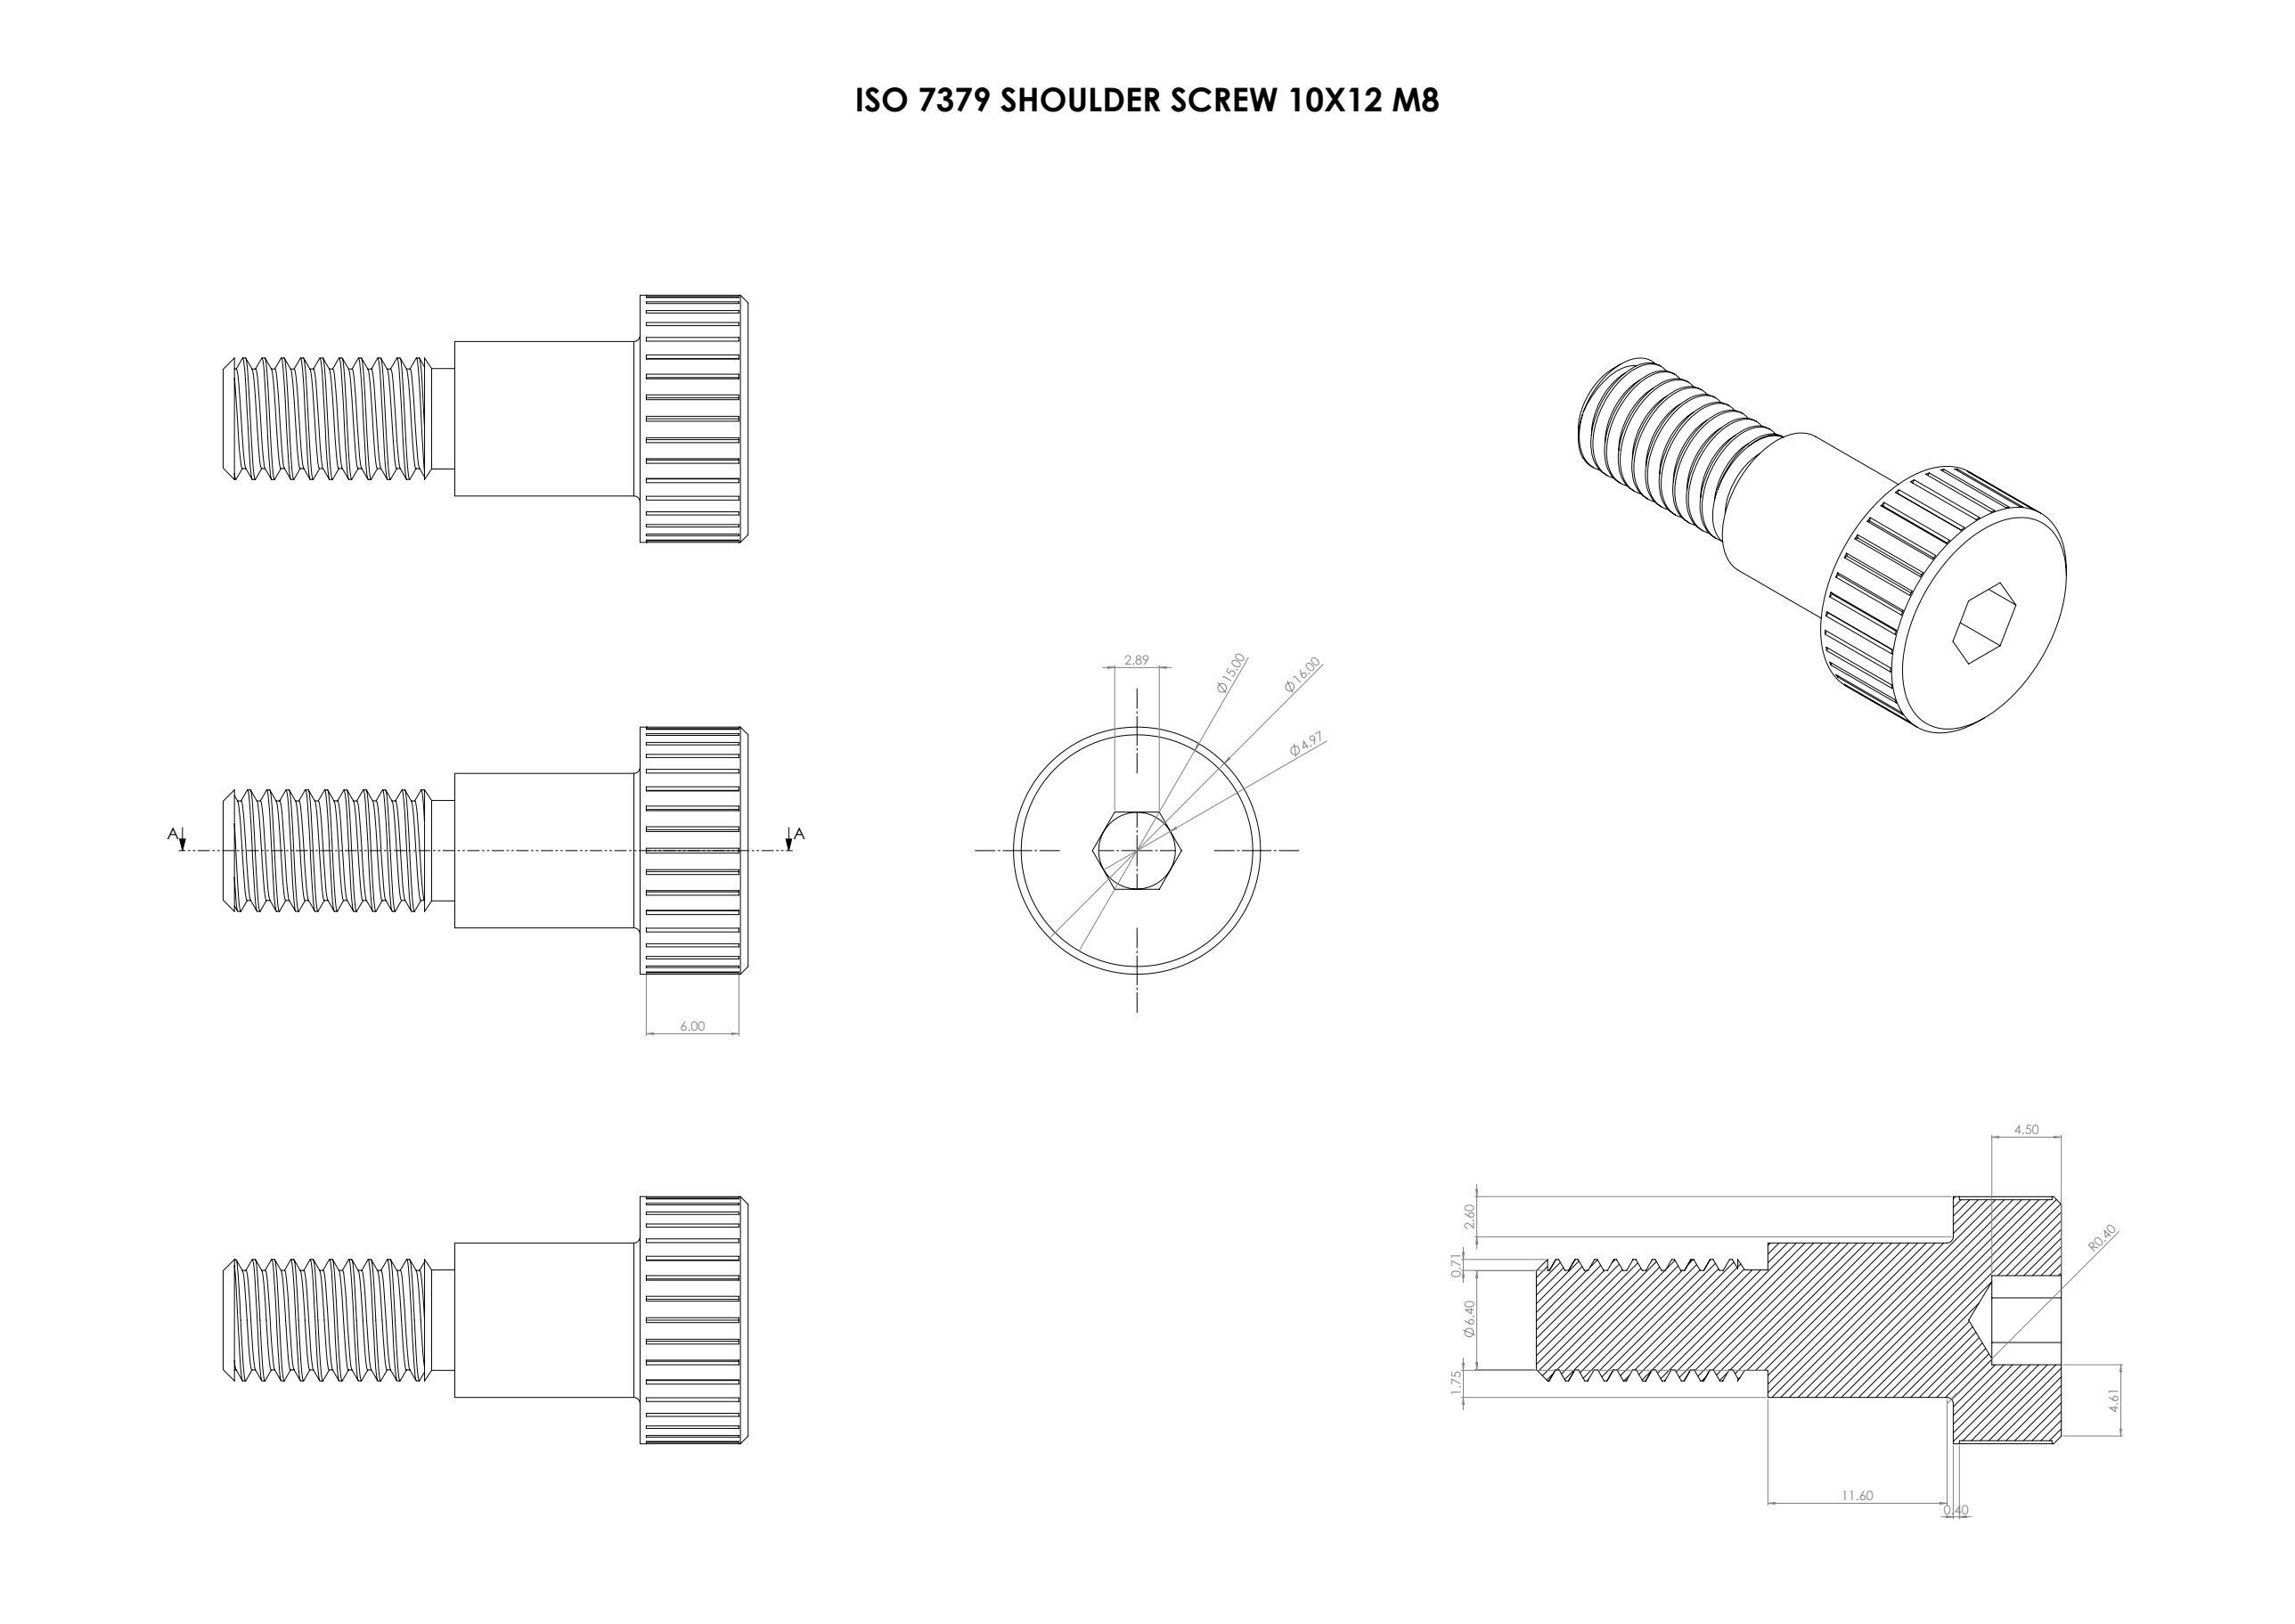
ISO-10303-21;
HEADER;
/* Generated by software containing ST-Developer
 * from STEP Tools, Inc. (www.steptools.com) 
 */

FILE_DESCRIPTION(
/* description */ (''),
/* implementation_level */ '2;1');

FILE_NAME(
/* name */ '11_ISO_7379_Shoulder_Screw_10x12_M8.step',
/* time_stamp */ '2026-10-21T01:56:51-07:00',
/* author */ (''),
/* organization */ (''),
/* preprocessor_version */ 'ST-DEVELOPER v20.2',
/* originating_system */ 'Autodesk Translation Framework v15.15.0.0',
/* authorisation */ '');

FILE_SCHEMA (('AUTOMOTIVE_DESIGN { 1 0 10303 214 3 1 1 }'));
ENDSEC;

DATA;
#10=MECHANICAL_DESIGN_GEOMETRIC_PRESENTATION_REPRESENTATION('',(#275),#82384);
#159=TOROIDAL_SURFACE('',#32042,5.4,0.4);
#237=SHAPE_REPRESENTATION_RELATIONSHIP('SRR','None',#82471,#256);
#256=ADVANCED_BREP_SHAPE_REPRESENTATION('',(#294),#82370);
#275=STYLED_ITEM('',(#82638),#294);
#294=MANIFOLD_SOLID_BREP('Body1',#30666);
#419=B_SPLINE_SURFACE_WITH_KNOTS('',3,3,((#47318,#47319,#47320,#47321,#47322,
#47323,#47324,#47325,#47326,#47327,#47328,#47329,#47330,#47331,#47332,#47333,
#47334,#47335,#47336,#47337,#47338,#47339,#47340,#47341,#47342,#47343,#47344,
#47345,#47346,#47347,#47348,#47349,#47350,#47351,#47352,#47353,#47354,#47355,
#47356,#47357,#47358,#47359,#47360,#47361,#47362,#47363,#47364,#47365,#47366,
#47367,#47368,#47369,#47370,#47371,#47372,#47373,#47374,#47375,#47376,#47377,
#47378,#47379,#47380,#47381,#47382,#47383,#47384),(#47385,#47386,#47387,
#47388,#47389,#47390,#47391,#47392,#47393,#47394,#47395,#47396,#47397,#47398,
#47399,#47400,#47401,#47402,#47403,#47404,#47405,#47406,#47407,#47408,#47409,
#47410,#47411,#47412,#47413,#47414,#47415,#47416,#47417,#47418,#47419,#47420,
#47421,#47422,#47423,#47424,#47425,#47426,#47427,#47428,#47429,#47430,#47431,
#47432,#47433,#47434,#47435,#47436,#47437,#47438,#47439,#47440,#47441,#47442,
#47443,#47444,#47445,#47446,#47447,#47448,#47449,#47450,#47451),(#47452,
#47453,#47454,#47455,#47456,#47457,#47458,#47459,#47460,#47461,#47462,#47463,
#47464,#47465,#47466,#47467,#47468,#47469,#47470,#47471,#47472,#47473,#47474,
#47475,#47476,#47477,#47478,#47479,#47480,#47481,#47482,#47483,#47484,#47485,
#47486,#47487,#47488,#47489,#47490,#47491,#47492,#47493,#47494,#47495,#47496,
#47497,#47498,#47499,#47500,#47501,#47502,#47503,#47504,#47505,#47506,#47507,
#47508,#47509,#47510,#47511,#47512,#47513,#47514,#47515,#47516,#47517,#47518),
(#47519,#47520,#47521,#47522,#47523,#47524,#47525,#47526,#47527,#47528,
#47529,#47530,#47531,#47532,#47533,#47534,#47535,#47536,#47537,#47538,#47539,
#47540,#47541,#47542,#47543,#47544,#47545,#47546,#47547,#47548,#47549,#47550,
#47551,#47552,#47553,#47554,#47555,#47556,#47557,#47558,#47559,#47560,#47561,
#47562,#47563,#47564,#47565,#47566,#47567,#47568,#47569,#47570,#47571,#47572,
#47573,#47574,#47575,#47576,#47577,#47578,#47579,#47580,#47581,#47582,#47583,
#47584,#47585)),.UNSPECIFIED.,.F.,.F.,.F.,(4,4),(4,1,1,1,1,1,1,1,1,1,1,
1,1,1,1,1,1,1,1,1,1,1,1,1,1,1,1,1,1,1,1,1,1,1,1,1,1,1,1,1,1,1,1,1,1,1,1,
1,1,1,1,1,1,1,1,1,1,1,1,1,1,1,1,1,4),(0.,0.0820126057383863),(8.31473274985803,
9.31389506365537,10.3130573774527,11.3122196912501,12.3113820050474,13.3105443188447,
14.3097066326421,15.3088689464394,16.3080312602368,17.3071935740341,18.3063558878314,
19.3055182016288,20.3046805154261,21.3038428292235,22.3030051430208,23.3021674568182,
24.3013297706155,25.3004920844128,26.2996543982102,27.2988167120075,28.2979790258049,
29.2971413396022,30.2963036533995,31.2954659671969,32.2946282809942,33.2937905947916,
34.2929529085889,35.2921152223863,36.2912775361836,37.2904398499809,38.2896021637783,
39.2887644775756,40.287926791373,41.2870891051703,42.2862514189677,43.285413732765,
44.2845760465623,45.2837383603597,46.282900674157,47.2820629879544,48.2812253017517,
49.280387615549,50.2795499293464,51.2787122431437,52.2778745569411,53.2770368707384,
54.2761991845358,55.2753614983331,56.2745238121304,57.2736861259278,58.2728484397251,
59.2720107535225,60.2711730673198,61.2703353811171,62.2694976949145,63.2686600087118,
64.2678223225092,65.2669846363065,66.2661469501039,67.2653092639012,68.2644715776985,
69.2636338914959,70.2627962052932,71.2619585190906,72.2611208328879),
 .UNSPECIFIED.);
#420=B_SPLINE_SURFACE_WITH_KNOTS('',3,3,((#47821,#47822,#47823,#47824,#47825,
#47826,#47827,#47828,#47829,#47830,#47831,#47832,#47833,#47834,#47835,#47836,
#47837,#47838,#47839,#47840,#47841,#47842,#47843,#47844,#47845,#47846,#47847,
#47848,#47849,#47850,#47851,#47852,#47853,#47854,#47855,#47856,#47857,#47858,
#47859,#47860,#47861,#47862,#47863,#47864,#47865,#47866,#47867,#47868,#47869,
#47870,#47871,#47872,#47873,#47874,#47875,#47876,#47877,#47878,#47879,#47880,
#47881,#47882,#47883,#47884,#47885,#47886,#47887),(#47888,#47889,#47890,
#47891,#47892,#47893,#47894,#47895,#47896,#47897,#47898,#47899,#47900,#47901,
#47902,#47903,#47904,#47905,#47906,#47907,#47908,#47909,#47910,#47911,#47912,
#47913,#47914,#47915,#47916,#47917,#47918,#47919,#47920,#47921,#47922,#47923,
#47924,#47925,#47926,#47927,#47928,#47929,#47930,#47931,#47932,#47933,#47934,
#47935,#47936,#47937,#47938,#47939,#47940,#47941,#47942,#47943,#47944,#47945,
#47946,#47947,#47948,#47949,#47950,#47951,#47952,#47953,#47954),(#47955,
#47956,#47957,#47958,#47959,#47960,#47961,#47962,#47963,#47964,#47965,#47966,
#47967,#47968,#47969,#47970,#47971,#47972,#47973,#47974,#47975,#47976,#47977,
#47978,#47979,#47980,#47981,#47982,#47983,#47984,#47985,#47986,#47987,#47988,
#47989,#47990,#47991,#47992,#47993,#47994,#47995,#47996,#47997,#47998,#47999,
#48000,#48001,#48002,#48003,#48004,#48005,#48006,#48007,#48008,#48009,#48010,
#48011,#48012,#48013,#48014,#48015,#48016,#48017,#48018,#48019,#48020,#48021),
(#48022,#48023,#48024,#48025,#48026,#48027,#48028,#48029,#48030,#48031,
#48032,#48033,#48034,#48035,#48036,#48037,#48038,#48039,#48040,#48041,#48042,
#48043,#48044,#48045,#48046,#48047,#48048,#48049,#48050,#48051,#48052,#48053,
#48054,#48055,#48056,#48057,#48058,#48059,#48060,#48061,#48062,#48063,#48064,
#48065,#48066,#48067,#48068,#48069,#48070,#48071,#48072,#48073,#48074,#48075,
#48076,#48077,#48078,#48079,#48080,#48081,#48082,#48083,#48084,#48085,#48086,
#48087,#48088)),.UNSPECIFIED.,.F.,.F.,.F.,(4,4),(4,1,1,1,1,1,1,1,1,1,1,
1,1,1,1,1,1,1,1,1,1,1,1,1,1,1,1,1,1,1,1,1,1,1,1,1,1,1,1,1,1,1,1,1,1,1,1,
1,1,1,1,1,1,1,1,1,1,1,1,1,1,1,1,1,4),(0.,0.0820126057383863),(11.6152142277547,
12.614376541552,13.6135388553494,14.6127011691467,15.6118634829441,16.6110257967414,
17.6101881105388,18.6093504243361,19.6085127381334,20.6076750519308,21.6068373657281,
22.6059996795255,23.6051619933228,24.6043243071202,25.6034866209175,26.6026489347148,
27.6018112485122,28.6009735623095,29.6001358761069,30.5992981899042,31.5984605037015,
32.5976228174989,33.5967851312962,34.5959474450936,35.5951097588909,36.5942720726883,
37.5934343864856,38.5925967002829,39.5917590140803,40.5909213278776,41.590083641675,
42.5892459554723,43.5884082692696,44.587570583067,45.5867328968643,46.5858952106617,
47.585057524459,48.5842198382564,49.5833821520537,50.582544465851,51.5817067796484,
52.5808690934457,53.5800314072431,54.5791937210404,55.5783560348378,56.5775183486351,
57.5766806624324,58.5758429762298,59.5750052900271,60.5741676038245,61.5733299176218,
62.5724922314191,63.5716545452165,64.5708168590138,65.5699791728112,66.5691414866085,
67.5683038004059,68.5674661142032,69.5666284280005,70.5657907417979,71.5649530555952,
72.5641153693926,73.5632776831899,74.5624399969873,75.5616023107846),
 .UNSPECIFIED.);
#548=CYLINDRICAL_SURFACE('',#31785,3.933);
#549=CYLINDRICAL_SURFACE('',#31787,3.933);
#550=CYLINDRICAL_SURFACE('',#31788,3.933);
#551=CYLINDRICAL_SURFACE('',#31789,3.933);
#552=CYLINDRICAL_SURFACE('',#31790,3.933);
#553=CYLINDRICAL_SURFACE('',#31791,3.933);
#554=CYLINDRICAL_SURFACE('',#31792,3.933);
#555=CYLINDRICAL_SURFACE('',#31793,3.933);
#556=CYLINDRICAL_SURFACE('',#31794,3.933);
#557=CYLINDRICAL_SURFACE('',#31795,3.933);
#558=CYLINDRICAL_SURFACE('',#31796,3.22275);
#559=CYLINDRICAL_SURFACE('',#31798,3.22275);
#560=CYLINDRICAL_SURFACE('',#31799,3.22275);
#561=CYLINDRICAL_SURFACE('',#31800,3.22275);
#562=CYLINDRICAL_SURFACE('',#31801,3.22275);
#563=CYLINDRICAL_SURFACE('',#31802,3.22275);
#564=CYLINDRICAL_SURFACE('',#31803,3.22275);
#565=CYLINDRICAL_SURFACE('',#31804,3.22275);
#566=CYLINDRICAL_SURFACE('',#31805,3.22275);
#567=CYLINDRICAL_SURFACE('',#31806,3.22275);
#568=CYLINDRICAL_SURFACE('',#31814,3.22275);
#569=CYLINDRICAL_SURFACE('',#32047,5.);
#570=CYLINDRICAL_SURFACE('',#32054,3.933);
#571=CYLINDRICAL_SURFACE('',#32058,3.25);
#572=CYLINDRICAL_SURFACE('',#32061,8.);
#1430=CIRCLE('',#31786,3.933);
#1431=CIRCLE('',#31797,3.22275);
#1432=CIRCLE('',#31808,3.933);
#1433=CIRCLE('',#31809,3.933);
#1434=CIRCLE('',#31811,3.933);
#1435=CIRCLE('',#31812,3.933);
#1436=CIRCLE('',#31813,3.22275);
#1437=CIRCLE('',#31817,8.);
#1438=CIRCLE('',#31820,8.);
#1439=CIRCLE('',#31823,8.);
#1440=CIRCLE('',#31826,8.);
#1441=CIRCLE('',#31829,8.);
#1442=CIRCLE('',#31832,8.);
#1443=CIRCLE('',#31835,8.);
#1444=CIRCLE('',#31838,8.);
#1445=CIRCLE('',#31841,8.);
#1446=CIRCLE('',#31844,8.);
#1447=CIRCLE('',#31847,8.);
#1448=CIRCLE('',#31850,8.);
#1449=CIRCLE('',#31853,8.);
#1450=CIRCLE('',#31856,8.);
#1451=CIRCLE('',#31859,8.);
#1452=CIRCLE('',#31862,8.);
#1453=CIRCLE('',#31865,8.);
#1454=CIRCLE('',#31868,8.);
#1455=CIRCLE('',#31871,8.);
#1456=CIRCLE('',#31874,8.);
#1457=CIRCLE('',#31877,8.);
#1458=CIRCLE('',#31880,8.);
#1459=CIRCLE('',#31883,8.);
#1460=CIRCLE('',#31886,8.);
#1461=CIRCLE('',#31889,8.);
#1462=CIRCLE('',#31892,8.);
#1463=CIRCLE('',#31895,8.);
#1464=CIRCLE('',#31898,8.);
#1465=CIRCLE('',#31901,8.);
#1466=CIRCLE('',#31904,8.);
#1467=CIRCLE('',#31907,8.);
#1468=CIRCLE('',#31910,8.);
#1469=CIRCLE('',#31913,8.);
#1470=CIRCLE('',#31916,8.);
#1471=CIRCLE('',#31919,8.);
#1472=CIRCLE('',#31920,8.);
#1473=CIRCLE('',#31923,8.);
#1474=CIRCLE('',#31924,8.);
#1475=CIRCLE('',#31927,8.);
#1476=CIRCLE('',#31930,8.);
#1477=CIRCLE('',#31933,8.);
#1478=CIRCLE('',#31936,8.);
#1479=CIRCLE('',#31939,8.);
#1480=CIRCLE('',#31942,8.);
#1481=CIRCLE('',#31945,8.);
#1482=CIRCLE('',#31948,8.);
#1483=CIRCLE('',#31951,8.);
#1484=CIRCLE('',#31954,8.);
#1485=CIRCLE('',#31957,8.);
#1486=CIRCLE('',#31960,8.);
#1487=CIRCLE('',#31963,8.);
#1488=CIRCLE('',#31966,8.);
#1489=CIRCLE('',#31969,8.);
#1490=CIRCLE('',#31972,8.);
#1491=CIRCLE('',#31975,8.);
#1492=CIRCLE('',#31978,8.);
#1493=CIRCLE('',#31981,8.);
#1494=CIRCLE('',#31984,8.);
#1495=CIRCLE('',#31987,8.);
#1496=CIRCLE('',#31990,8.);
#1497=CIRCLE('',#31993,8.);
#1498=CIRCLE('',#31996,8.);
#1499=CIRCLE('',#31999,8.);
#1500=CIRCLE('',#32002,8.);
#1501=CIRCLE('',#32005,8.);
#1502=CIRCLE('',#32008,8.);
#1503=CIRCLE('',#32011,8.);
#1504=CIRCLE('',#32014,8.);
#1505=CIRCLE('',#32017,8.);
#1506=CIRCLE('',#32020,8.);
#1507=CIRCLE('',#32023,8.);
#1508=CIRCLE('',#32026,8.);
#1509=CIRCLE('',#32029,8.);
#1510=CIRCLE('',#32032,8.);
#1511=CIRCLE('',#32034,2.48346726553949);
#1512=CIRCLE('',#32043,5.);
#1513=CIRCLE('',#32044,0.4);
#1514=CIRCLE('',#32045,5.4);
#1515=CIRCLE('',#32046,5.);
#1516=CIRCLE('',#32048,5.);
#1517=CIRCLE('',#32050,8.);
#1518=CIRCLE('',#32052,3.2);
#1519=CIRCLE('',#32055,3.933);
#1520=CIRCLE('',#32057,3.25);
#1521=CIRCLE('',#32059,3.25);
#1522=CIRCLE('',#32062,8.);
#1523=CIRCLE('',#32064,7.5);
#2031=CONICAL_SURFACE('',#32033,1.25,1.02681050468488);
#2032=CONICAL_SURFACE('',#32053,3.6,0.785398163397448);
#2033=CONICAL_SURFACE('',#32056,3.625,0.982793723247331);
#2034=CONICAL_SURFACE('',#32063,7.75,0.78539816339745);
#2326=B_SPLINE_CURVE_WITH_KNOTS('',3,(#46419,#46420,#46421,#46422,#46423,
#46424,#46425,#46426,#46427,#46428),.UNSPECIFIED.,.F.,.F.,(4,3,3,4),(-4.0927490401942,
-3.99664925518937,-2.99748694139203,-2.06120159751576),.UNSPECIFIED.);
#2327=B_SPLINE_CURVE_WITH_KNOTS('',3,(#46431,#46432,#46433,#46434,#46435,
#46436,#46437),.UNSPECIFIED.,.F.,.F.,(4,3,4),(0.,0.999162313797346,1.11004521091126),
 .UNSPECIFIED.);
#2328=B_SPLINE_CURVE_WITH_KNOTS('',3,(#46442,#46443,#46444,#46445,#46446,
#46447,#46448,#46449,#46450,#46451,#46452,#46453,#46454,#46455,#46456,#46457,
#46458,#46459,#46460,#46461,#46462,#46463),.UNSPECIFIED.,.F.,.F.,(4,3,3,
3,3,3,3,4),(-10.3759343473738,-9.99162313797342,-8.99246082417608,-7.99329851037874,
-6.9941361965814,-5.99497388278405,-4.99581156898671,-4.0927490401942),
 .UNSPECIFIED.);
#2329=B_SPLINE_CURVE_WITH_KNOTS('',3,(#46464,#46465,#46466,#46467,#46468,
#46469,#46470,#46471,#46472,#46473,#46474,#46475,#46476,#46477,#46478,#46479,
#46480,#46481,#46482,#46483,#46484,#46485),.UNSPECIFIED.,.F.,.F.,(4,3,3,
3,3,3,3,4),(1.11004521091126,1.99832462759469,2.99748694139203,3.99664925518937,
4.99581156898671,5.99497388278405,6.9941361965814,7.39323051809085),
 .UNSPECIFIED.);
#2330=B_SPLINE_CURVE_WITH_KNOTS('',3,(#46490,#46491,#46492,#46493,#46494,
#46495,#46496,#46497,#46498,#46499,#46500,#46501,#46502,#46503,#46504,#46505,
#46506,#46507,#46508,#46509,#46510,#46511),.UNSPECIFIED.,.F.,.F.,(4,3,3,
3,3,3,3,4),(-16.6591196545534,-15.9865970207575,-14.9874347069601,-13.9882723931628,
-12.9891100793654,-11.9899477655681,-10.9907854517708,-10.3759343473738),
 .UNSPECIFIED.);
#2331=B_SPLINE_CURVE_WITH_KNOTS('',3,(#46512,#46513,#46514,#46515,#46516,
#46517,#46518,#46519,#46520,#46521,#46522,#46523,#46524,#46525,#46526,#46527,
#46528,#46529,#46530,#46531,#46532,#46533),.UNSPECIFIED.,.F.,.F.,(4,3,3,
3,3,3,3,4),(7.39323051809085,7.99329851037874,8.99246082417608,9.99162313797342,
10.9907854517708,11.9899477655681,12.9891100793654,13.6764158252704),
 .UNSPECIFIED.);
#2332=B_SPLINE_CURVE_WITH_KNOTS('',3,(#46538,#46539,#46540,#46541,#46542,
#46543,#46544,#46545,#46546,#46547,#46548,#46549,#46550,#46551,#46552,#46553,
#46554,#46555,#46556,#46557,#46558,#46559),.UNSPECIFIED.,.F.,.F.,(4,3,3,
3,3,3,3,4),(-22.942304961733,-21.9815709035415,-20.9824085897442,-19.9832462759468,
-18.9840839621495,-17.9849216483522,-16.9857593345548,-16.6591196545534),
 .UNSPECIFIED.);
#2333=B_SPLINE_CURVE_WITH_KNOTS('',3,(#46560,#46561,#46562,#46563,#46564,
#46565,#46566,#46567,#46568,#46569,#46570,#46571,#46572,#46573,#46574,#46575,
#46576,#46577,#46578,#46579,#46580,#46581),.UNSPECIFIED.,.F.,.F.,(4,3,3,
3,3,3,3,4),(13.6764158252704,13.9882723931628,14.9874347069601,15.9865970207575,
16.9857593345548,17.9849216483522,18.9840839621495,19.95960113245),
 .UNSPECIFIED.);
#2334=B_SPLINE_CURVE_WITH_KNOTS('',3,(#46586,#46587,#46588,#46589,#46590,
#46591,#46592,#46593,#46594,#46595,#46596,#46597,#46598,#46599,#46600,#46601,
#46602,#46603,#46604,#46605,#46606,#46607,#46608,#46609,#46610),
 .UNSPECIFIED.,.F.,.F.,(4,3,3,3,3,3,3,3,4),(-29.2254902689126,-28.9757071001229,
-27.9765447863256,-26.9773824725282,-25.9782201587309,-24.9790578449336,
-23.9798955311362,-22.9807332173389,-22.942304961733),.UNSPECIFIED.);
#2335=B_SPLINE_CURVE_WITH_KNOTS('',3,(#46611,#46612,#46613,#46614,#46615,
#46616,#46617,#46618,#46619,#46620,#46621,#46622,#46623,#46624,#46625,#46626,
#46627,#46628,#46629,#46630,#46631,#46632,#46633,#46634,#46635),
 .UNSPECIFIED.,.F.,.F.,(4,3,3,3,3,3,3,3,4),(19.95960113245,19.9832462759468,
20.9824085897442,21.9815709035415,22.9807332173389,23.9798955311362,24.9790578449335,
25.9782201587309,26.2427864396296),.UNSPECIFIED.);
#2336=B_SPLINE_CURVE_WITH_KNOTS('',3,(#46640,#46641,#46642,#46643,#46644,
#46645,#46646,#46647,#46648,#46649,#46650,#46651,#46652,#46653,#46654,#46655,
#46656,#46657,#46658,#46659,#46660,#46661),.UNSPECIFIED.,.F.,.F.,(4,3,3,
3,3,3,3,4),(-35.5086755760921,-34.970680982907,-33.9715186691096,-32.9723563553123,
-31.9731940415149,-30.9740317277176,-29.9748694139203,-29.2254902689126),
 .UNSPECIFIED.);
#2337=B_SPLINE_CURVE_WITH_KNOTS('',3,(#46662,#46663,#46664,#46665,#46666,
#46667,#46668,#46669,#46670,#46671,#46672,#46673,#46674,#46675,#46676,#46677,
#46678,#46679,#46680,#46681,#46682,#46683),.UNSPECIFIED.,.F.,.F.,(4,3,3,
3,3,3,3,4),(26.2427864396296,26.9773824725282,27.9765447863256,28.9757071001229,
29.9748694139203,30.9740317277176,31.9731940415149,32.5259717468092),
 .UNSPECIFIED.);
#2338=B_SPLINE_CURVE_WITH_KNOTS('',3,(#46688,#46689,#46690,#46691,#46692,
#46693,#46694,#46695,#46696,#46697,#46698,#46699,#46700,#46701,#46702,#46703,
#46704,#46705,#46706,#46707,#46708,#46709),.UNSPECIFIED.,.F.,.F.,(4,3,3,
3,3,3,3,4),(-41.7918608832717,-40.965654865691,-39.9664925518937,-38.9673302380963,
-37.968167924299,-36.9690056105017,-35.9698432967043,-35.5086755760921),
 .UNSPECIFIED.);
#2339=B_SPLINE_CURVE_WITH_KNOTS('',3,(#46710,#46711,#46712,#46713,#46714,
#46715,#46716,#46717,#46718,#46719,#46720,#46721,#46722,#46723,#46724,#46725,
#46726,#46727,#46728,#46729,#46730,#46731),.UNSPECIFIED.,.F.,.F.,(4,3,3,
3,3,3,3,4),(32.5259717468092,32.9723563553123,33.9715186691096,34.970680982907,
35.9698432967043,36.9690056105017,37.968167924299,38.8091570539888),
 .UNSPECIFIED.);
#2340=B_SPLINE_CURVE_WITH_KNOTS('',3,(#46736,#46737,#46738,#46739,#46740,
#46741,#46742,#46743,#46744,#46745,#46746,#46747,#46748,#46749,#46750,#46751,
#46752,#46753,#46754,#46755,#46756,#46757,#46758,#46759,#46760),
 .UNSPECIFIED.,.F.,.F.,(4,3,3,3,3,3,3,3,4),(-48.0750461904513,-47.9597910622724,
-46.9606287484751,-45.9614664346777,-44.9623041208804,-43.9631418070831,
-42.9639794932857,-41.9648171794884,-41.7918608832717),.UNSPECIFIED.);
#2341=B_SPLINE_CURVE_WITH_KNOTS('',3,(#46761,#46762,#46763,#46764,#46765,
#46766,#46767,#46768,#46769,#46770,#46771,#46772,#46773,#46774,#46775,#46776,
#46777,#46778,#46779,#46780,#46781,#46782,#46783,#46784,#46785),
 .UNSPECIFIED.,.F.,.F.,(4,3,3,3,3,3,3,3,4),(38.8091570539888,38.9673302380963,
39.9664925518937,40.965654865691,41.9648171794884,42.9639794932857,43.963141807083,
44.9623041208804,45.0923423611684),.UNSPECIFIED.);
#2342=B_SPLINE_CURVE_WITH_KNOTS('',3,(#46790,#46791,#46792,#46793,#46794,
#46795,#46796,#46797,#46798,#46799,#46800,#46801,#46802,#46803,#46804,#46805,
#46806,#46807,#46808,#46809,#46810,#46811),.UNSPECIFIED.,.F.,.F.,(4,3,3,
3,3,3,3,4),(-54.3582314976309,-53.9547649450565,-52.9556026312591,-51.9564403174618,
-50.9572780036644,-49.9581156898671,-48.9589533760698,-48.0750461904513),
 .UNSPECIFIED.);
#2343=B_SPLINE_CURVE_WITH_KNOTS('',3,(#46812,#46813,#46814,#46815,#46816,
#46817,#46818,#46819,#46820,#46821,#46822,#46823,#46824,#46825,#46826,#46827,
#46828,#46829,#46830,#46831,#46832,#46833),.UNSPECIFIED.,.F.,.F.,(4,3,3,
3,3,3,3,4),(45.0923423611684,45.9614664346777,46.9606287484751,47.9597910622724,
48.9589533760698,49.9581156898671,50.9572780036644,51.375527668348),
 .UNSPECIFIED.);
#2344=B_SPLINE_CURVE_WITH_KNOTS('',3,(#46838,#46839,#46840,#46841,#46842,
#46843,#46844,#46845,#46846,#46847,#46848,#46849,#46850,#46851,#46852,#46853,
#46854,#46855,#46856,#46857,#46858,#46859),.UNSPECIFIED.,.F.,.F.,(4,3,3,
3,3,3,3,4),(-60.6414168048105,-59.9497388278405,-58.9505765140432,-57.9514142002458,
-56.9522518864485,-55.9530895726512,-54.9539272588538,-54.3582314976309),
 .UNSPECIFIED.);
#2345=B_SPLINE_CURVE_WITH_KNOTS('',3,(#46860,#46861,#46862,#46863,#46864,
#46865,#46866,#46867,#46868,#46869,#46870,#46871,#46872,#46873,#46874,#46875,
#46876,#46877,#46878,#46879,#46880,#46881),.UNSPECIFIED.,.F.,.F.,(4,3,3,
3,3,3,3,4),(51.375527668348,51.9564403174618,52.9556026312591,53.9547649450565,
54.9539272588538,55.9530895726512,56.9522518864485,57.6587129755276),
 .UNSPECIFIED.);
#2346=B_SPLINE_CURVE_WITH_KNOTS('',3,(#46887,#46888,#46889,#46890,#46891),
 .UNSPECIFIED.,.F.,.F.,(4,1,4),(72.2566310325653,72.5641153693926,73.5004007132688),
 .UNSPECIFIED.);
#2347=B_SPLINE_CURVE_WITH_KNOTS('',3,(#46894,#46895,#46896,#46897),
 .UNSPECIFIED.,.F.,.F.,(4,4),(72.2566310325652,72.2611208328879),
 .UNSPECIFIED.);
#2348=B_SPLINE_CURVE_WITH_KNOTS('',3,(#46902,#46903,#46904,#46905,#46906,
#46907,#46908,#46909,#46910,#46911),.UNSPECIFIED.,.F.,.F.,(4,1,1,1,1,1,
1,4),(65.9734457253856,66.5691414866085,67.5683038004059,68.5674661142032,
69.5666284280005,70.5657907417979,71.5649530555952,72.2566310325653),
 .UNSPECIFIED.);
#2349=B_SPLINE_CURVE_WITH_KNOTS('',3,(#46912,#46913,#46914,#46915,#46916,
#46917,#46918,#46919,#46920,#46921),.UNSPECIFIED.,.F.,.F.,(4,1,1,1,1,1,
1,4),(65.9734457253856,66.2661469501039,67.2653092639012,68.2644715776985,
69.2636338914959,70.2627962052932,71.2619585190906,72.2566310325652),
 .UNSPECIFIED.);
#2350=B_SPLINE_CURVE_WITH_KNOTS('',3,(#46926,#46927,#46928,#46929,#46930,
#46931,#46932,#46933,#46934,#46935),.UNSPECIFIED.,.F.,.F.,(4,1,1,1,1,1,
1,4),(59.6902604182061,60.5741676038245,61.5733299176218,62.5724922314191,
63.5716545452165,64.5708168590138,65.5699791728112,65.9734457253856),
 .UNSPECIFIED.);
#2351=B_SPLINE_CURVE_WITH_KNOTS('',3,(#46936,#46937,#46938,#46939,#46940,
#46941,#46942,#46943,#46944,#46945),.UNSPECIFIED.,.F.,.F.,(4,1,1,1,1,1,
1,4),(59.6902604182061,60.2711730673198,61.2703353811171,62.2694976949145,
63.2686600087118,64.2678223225092,65.2669846363065,65.9734457253856),
 .UNSPECIFIED.);
#2352=B_SPLINE_CURVE_WITH_KNOTS('',3,(#46950,#46951,#46952,#46953,#46954,
#46955,#46956,#46957,#46958,#46959,#46960),.UNSPECIFIED.,.F.,.F.,(4,1,1,
1,1,1,1,1,4),(53.4070751110265,53.5800314072431,54.5791937210404,55.5783560348378,
56.5775183486351,57.5766806624324,58.5758429762298,59.5750052900271,59.6902604182061),
 .UNSPECIFIED.);
#2353=B_SPLINE_CURVE_WITH_KNOTS('',3,(#46961,#46962,#46963,#46964,#46965,
#46966,#46967,#46968,#46969,#46970),.UNSPECIFIED.,.F.,.F.,(4,1,1,1,1,1,
1,4),(53.4070751110265,54.2761991845358,55.2753614983331,56.2745238121304,
57.2736861259278,58.2728484397251,59.2720107535225,59.6902604182061),
 .UNSPECIFIED.);
#2354=B_SPLINE_CURVE_WITH_KNOTS('',3,(#46975,#46976,#46977,#46978,#46979,
#46980,#46981,#46982,#46983,#46984),.UNSPECIFIED.,.F.,.F.,(4,1,1,1,1,1,
1,4),(47.1238898038469,47.585057524459,48.5842198382564,49.5833821520537,
50.582544465851,51.5817067796484,52.5808690934457,53.4070751110265),
 .UNSPECIFIED.);
#2355=B_SPLINE_CURVE_WITH_KNOTS('',3,(#46985,#46986,#46987,#46988,#46989,
#46990,#46991,#46992,#46993,#46994,#46995),.UNSPECIFIED.,.F.,.F.,(4,1,1,
1,1,1,1,1,4),(47.1238898038469,47.2820629879544,48.2812253017517,49.280387615549,
50.2795499293464,51.2787122431437,52.2778745569411,53.2770368707384,53.4070751110265),
 .UNSPECIFIED.);
#2356=B_SPLINE_CURVE_WITH_KNOTS('',3,(#47000,#47001,#47002,#47003,#47004,
#47005,#47006,#47007,#47008,#47009),.UNSPECIFIED.,.F.,.F.,(4,1,1,1,1,1,
1,4),(40.8407044966673,41.590083641675,42.5892459554723,43.5884082692696,
44.587570583067,45.5867328968643,46.5858952106617,47.1238898038469),
 .UNSPECIFIED.);
#2357=B_SPLINE_CURVE_WITH_KNOTS('',3,(#47010,#47011,#47012,#47013,#47014,
#47015,#47016,#47017,#47018,#47019),.UNSPECIFIED.,.F.,.F.,(4,1,1,1,1,1,
1,4),(40.8407044966673,41.2870891051703,42.2862514189677,43.285413732765,
44.2845760465623,45.2837383603597,46.282900674157,47.1238898038469),
 .UNSPECIFIED.);
#2358=B_SPLINE_CURVE_WITH_KNOTS('',3,(#47024,#47025,#47026,#47027,#47028,
#47029,#47030,#47031,#47032,#47033,#47034),.UNSPECIFIED.,.F.,.F.,(4,1,1,
1,1,1,1,1,4),(34.5575191894877,34.5959474450936,35.5951097588909,36.5942720726883,
37.5934343864856,38.5925967002829,39.5917590140803,40.5909213278776,40.8407044966673),
 .UNSPECIFIED.);
#2359=B_SPLINE_CURVE_WITH_KNOTS('',3,(#47035,#47036,#47037,#47038,#47039,
#47040,#47041,#47042,#47043,#47044),.UNSPECIFIED.,.F.,.F.,(4,1,1,1,1,1,
1,4),(34.5575191894877,35.2921152223863,36.2912775361836,37.2904398499809,
38.2896021637783,39.2887644775756,40.287926791373,40.8407044966673),
 .UNSPECIFIED.);
#2360=B_SPLINE_CURVE_WITH_KNOTS('',3,(#47049,#47050,#47051,#47052,#47053,
#47054,#47055,#47056,#47057,#47058),.UNSPECIFIED.,.F.,.F.,(4,1,1,1,1,1,
1,4),(28.2743338823081,28.6009735623095,29.6001358761069,30.5992981899042,
31.5984605037015,32.5976228174989,33.5967851312962,34.5575191894877),
 .UNSPECIFIED.);
#2361=B_SPLINE_CURVE_WITH_KNOTS('',3,(#47059,#47060,#47061,#47062,#47063,
#47064,#47065,#47066,#47067,#47068,#47069),.UNSPECIFIED.,.F.,.F.,(4,1,1,
1,1,1,1,1,4),(28.2743338823081,28.2979790258049,29.2971413396022,30.2963036533995,
31.2954659671969,32.2946282809942,33.2937905947916,34.2929529085889,34.5575191894877),
 .UNSPECIFIED.);
#2362=B_SPLINE_CURVE_WITH_KNOTS('',3,(#47074,#47075,#47076,#47077,#47078,
#47079,#47080,#47081,#47082,#47083),.UNSPECIFIED.,.F.,.F.,(4,1,1,1,1,1,
1,4),(21.9911485751285,22.6059996795255,23.6051619933228,24.6043243071202,
25.6034866209175,26.6026489347148,27.6018112485122,28.2743338823081),
 .UNSPECIFIED.);
#2363=B_SPLINE_CURVE_WITH_KNOTS('',3,(#47084,#47085,#47086,#47087,#47088,
#47089,#47090,#47091,#47092,#47093),.UNSPECIFIED.,.F.,.F.,(4,1,1,1,1,1,
1,4),(21.9911485751285,22.3030051430208,23.3021674568182,24.3013297706155,
25.3004920844128,26.2996543982102,27.2988167120075,28.2743338823081),
 .UNSPECIFIED.);
#2364=B_SPLINE_CURVE_WITH_KNOTS('',3,(#47098,#47099,#47100,#47101,#47102,
#47103,#47104,#47105,#47106,#47107),.UNSPECIFIED.,.F.,.F.,(4,1,1,1,1,1,
1,4),(15.7079632679489,16.6110257967414,17.6101881105388,18.6093504243361,
19.6085127381334,20.6076750519308,21.6068373657281,21.9911485751285),
 .UNSPECIFIED.);
#2365=B_SPLINE_CURVE_WITH_KNOTS('',3,(#47108,#47109,#47110,#47111,#47112,
#47113,#47114,#47115,#47116,#47117),.UNSPECIFIED.,.F.,.F.,(4,1,1,1,1,1,
1,4),(15.7079632679489,16.3080312602368,17.3071935740341,18.3063558878314,
19.3055182016288,20.3046805154261,21.3038428292235,21.9911485751285),
 .UNSPECIFIED.);
#2366=B_SPLINE_CURVE_WITH_KNOTS('',3,(#47120,#47121,#47122,#47123,#47124,
#47125,#47126,#47127,#47128,#47129,#47130,#47131,#47132,#47133,#47134,#47135,
#47136,#47137,#47138,#47139,#47140,#47141,#47142,#47143,#47144,#47145,#47146,
#47147,#47148,#47149,#47150,#47151,#47152,#47153,#47154,#47155,#47156,#47157,
#47158,#47159,#47160,#47161,#47162,#47163,#47164,#47165,#47166,#47167,#47168,
#47169,#47170,#47171,#47172,#47173,#47174,#47175,#47176,#47177,#47178,#47179,
#47180,#47181,#47182,#47183,#47184,#47185,#47186,#47187,#47188,#47189,#47190,
#47191,#47192,#47193,#47194,#47195,#47196,#47197,#47198,#47199,#47200,#47201,
#47202,#47203,#47204,#47205,#47206,#47207,#47208,#47209,#47210,#47211,#47212,
#47213,#47214,#47215,#47216),.UNSPECIFIED.,.F.,.F.,(4,3,3,3,3,3,3,3,3,3,
3,3,3,3,3,3,3,3,3,3,3,3,3,3,3,3,3,3,3,3,3,3,4),(-0.744397949170578,-0.723859366608779,
-0.692778390163693,-0.673163388835089,-0.66062832497008,-0.654997428133838,
-0.623000635306235,-0.592492852006209,-0.579145696812448,-0.572539965631915,
-0.567831580001411,-0.534463688691448,-0.50057067124518,-0.46675792585302,
-0.444803036616271,-0.438632777591669,-0.432866104431837,-0.397950947955525,
-0.378938368906026,-0.345225723678728,-0.310871405360981,-0.300047867503053,
-0.295192728302996,-0.260846341462991,-0.225369180435003,-0.189533834845717,
-0.165842105490003,-0.154268999879935,-0.147059086804718,-0.110294315103539,
-0.0734873168420825,-0.0367436584210412,0.),.UNSPECIFIED.);
#2367=B_SPLINE_CURVE_WITH_KNOTS('',3,(#47221,#47222,#47223,#47224,#47225,
#47226,#47227,#47228,#47229,#47230,#47231,#47232,#47233,#47234,#47235,#47236,
#47237,#47238,#47239,#47240,#47241,#47242,#47243,#47244,#47245,#47246,#47247,
#47248,#47249,#47250,#47251,#47252,#47253,#47254,#47255,#47256,#47257,#47258,
#47259,#47260,#47261,#47262,#47263,#47264,#47265,#47266,#47267,#47268,#47269,
#47270,#47271,#47272,#47273,#47274,#47275,#47276,#47277,#47278,#47279,#47280,
#47281,#47282,#47283,#47284,#47285,#47286,#47287,#47288,#47289,#47290,#47291,
#47292,#47293,#47294,#47295,#47296,#47297,#47298,#47299,#47300,#47301,#47302,
#47303,#47304,#47305,#47306,#47307,#47308,#47309,#47310,#47311,#47312,#47313,
#47314,#47315,#47316,#47317),.UNSPECIFIED.,.F.,.F.,(4,3,3,3,3,3,3,3,3,3,
3,3,3,3,3,3,3,3,3,3,3,3,3,3,3,3,3,3,3,3,3,3,4),(-0.741270768406328,-0.716584367599815,
-0.680056248148676,-0.658907114297353,-0.642813303176804,-0.636134709402922,
-0.599326634043495,-0.567119568103997,-0.553028976755466,-0.544366227927849,
-0.537678034880734,-0.502276348317679,-0.467136809341096,-0.43303532712436,
-0.410194021975148,-0.39912856359863,-0.394448100777585,-0.360831295807122,
-0.341670106527509,-0.307405657582616,-0.272989575876299,-0.262610092909626,
-0.257322277143721,-0.223891952452371,-0.190429464967423,-0.15737798688834,
-0.137705738527298,-0.128679290433546,-0.124522260753379,-0.0923095570632588,
-0.0605443501164106,-0.0297602312950581,0.),.UNSPECIFIED.);
#2368=B_SPLINE_CURVE_WITH_KNOTS('',3,(#47586,#47587,#47588,#47589,#47590,
#47591,#47592,#47593,#47594,#47595,#47596,#47597,#47598,#47599,#47600,#47601),
 .UNSPECIFIED.,.F.,.F.,(4,3,3,3,3,4),(57.6587129755276,57.9514142002458,
58.9505765140432,59.9497388278405,60.9489011416379,61.8851864855141),
 .UNSPECIFIED.);
#2369=B_SPLINE_CURVE_WITH_KNOTS('',3,(#47603,#47604,#47605,#47606,#47607,
#47608,#47609,#47610,#47611,#47612,#47613,#47614,#47615,#47616,#47617,#47618,
#47619,#47620,#47621,#47622,#47623,#47624,#47625,#47626,#47627,#47628,#47629,
#47630,#47631,#47632,#47633,#47634,#47635,#47636,#47637,#47638,#47639,#47640,
#47641,#47642,#47643,#47644,#47645,#47646,#47647,#47648,#47649,#47650,#47651,
#47652,#47653,#47654,#47655,#47656,#47657,#47658,#47659,#47660,#47661,#47662,
#47663,#47664,#47665,#47666,#47667,#47668,#47669,#47670,#47671,#47672,#47673,
#47674,#47675,#47676,#47677,#47678,#47679,#47680,#47681,#47682,#47683,#47684,
#47685,#47686,#47687,#47688,#47689,#47690,#47691,#47692,#47693,#47694,#47695,
#47696,#47697,#47698,#47699),.UNSPECIFIED.,.F.,.F.,(4,3,3,3,3,3,3,3,3,3,
3,3,3,3,3,3,3,3,3,3,3,3,3,3,3,3,3,3,3,3,3,3,4),(-0.744397949170611,-0.723859366608811,
-0.692778425140133,-0.673163421625501,-0.66062836032772,-0.654997464717496,
-0.623000702910192,-0.592492911159671,-0.579145752268819,-0.572540185113237,
-0.567831953655538,-0.53446408683659,-0.50057107660485,-0.466758326635226,
-0.444803337202926,-0.438637144898971,-0.432867617692046,-0.397952458797699,
-0.378938368906029,-0.345225738440821,-0.310871437714059,-0.300047912343567,
-0.295192811934132,-0.260846440789055,-0.225369298521846,-0.189533961517898,
-0.16584221632816,-0.154269162505787,-0.147059061291272,-0.110294295968454,
-0.0734872911176007,-0.0367436455588004,0.),.UNSPECIFIED.);
#2370=B_SPLINE_CURVE_WITH_KNOTS('',3,(#47700,#47701,#47702,#47703,#47704,
#47705,#47706,#47707,#47708),.UNSPECIFIED.,.F.,.F.,(4,1,1,1,1,1,4),(10.3759343473738,
11.3122196912501,12.3113820050474,13.3105443188447,14.3097066326421,15.3088689464394,
15.7079632679489),.UNSPECIFIED.);
#2371=B_SPLINE_CURVE_WITH_KNOTS('',3,(#47714,#47715,#47716,#47717,#47718,
#47719,#47720,#47721,#47722,#47723,#47724,#47725,#47726,#47727,#47728,#47729,
#47730,#47731,#47732,#47733,#47734,#47735,#47736,#47737,#47738,#47739,#47740,
#47741,#47742,#47743,#47744,#47745,#47746,#47747,#47748,#47749,#47750,#47751,
#47752,#47753,#47754,#47755,#47756,#47757,#47758,#47759,#47760,#47761,#47762,
#47763,#47764,#47765,#47766,#47767,#47768,#47769,#47770,#47771,#47772,#47773,
#47774,#47775,#47776,#47777,#47778,#47779,#47780,#47781,#47782,#47783,#47784,
#47785,#47786,#47787,#47788,#47789,#47790,#47791,#47792,#47793,#47794,#47795,
#47796,#47797,#47798,#47799,#47800,#47801,#47802,#47803,#47804,#47805,#47806,
#47807,#47808,#47809,#47810),.UNSPECIFIED.,.F.,.F.,(4,3,3,3,3,3,3,3,3,3,
3,3,3,3,3,3,3,3,3,3,3,3,3,3,3,3,3,3,3,3,3,3,4),(-0.741270768406356,-0.716584367599843,
-0.680056245830011,-0.658907112123604,-0.642813301702322,-0.636134706984057,
-0.599326631926989,-0.567119566252054,-0.55302897501927,-0.54436621135304,
-0.537678029406459,-0.502276340484753,-0.467136787004678,-0.433035266636814,
-0.410193976609488,-0.399128488173405,-0.394447934771061,-0.360831102765067,
-0.341670106527508,-0.307405637245107,-0.272989559930472,-0.262610069828679,
-0.257322284490531,-0.223891948269394,-0.190429473282791,-0.157378031219309,
-0.137705777316896,-0.128679430637047,-0.124522456571441,-0.0923097812005346,
-0.0605446165933425,-0.0297605544881402,0.),.UNSPECIFIED.);
#2372=B_SPLINE_CURVE_WITH_KNOTS('',3,(#47813,#47814,#47815,#47816,#47817,
#47818,#47819,#47820),.UNSPECIFIED.,.F.,.F.,(4,1,1,1,1,4),(11.6152142277547,
12.614376541552,13.6135388553494,14.6127011691467,15.6118634829441,15.7079632679489),
 .UNSPECIFIED.);
#2373=B_SPLINE_CURVE_WITH_KNOTS('',3,(#48089,#48090,#48091,#48092,#48093,
#48094,#48095,#48096,#48097,#48098,#48099,#48100,#48101),.UNSPECIFIED.,
 .F.,.F.,(4,3,3,3,4),(-63.9463880830299,-62.9472257692326,-61.9480634554352,
-60.9489011416379,-60.6414168048105),.UNSPECIFIED.);
#3445=FACE_BOUND('',#6276,.T.);
#3446=FACE_BOUND('',#6280,.T.);
#3447=FACE_BOUND('',#6287,.T.);
#3448=FACE_BOUND('',#6289,.T.);
#3449=FACE_BOUND('',#6290,.T.);
#3450=FACE_BOUND('',#6291,.T.);
#3451=FACE_BOUND('',#6292,.T.);
#3452=FACE_BOUND('',#6293,.T.);
#3453=FACE_BOUND('',#6294,.T.);
#3454=FACE_BOUND('',#6295,.T.);
#3455=FACE_BOUND('',#6296,.T.);
#3456=FACE_BOUND('',#6297,.T.);
#3457=FACE_BOUND('',#6298,.T.);
#3458=FACE_BOUND('',#6299,.T.);
#3459=FACE_BOUND('',#6300,.T.);
#3460=FACE_BOUND('',#6301,.T.);
#3461=FACE_BOUND('',#6302,.T.);
#3462=FACE_BOUND('',#6303,.T.);
#3463=FACE_BOUND('',#6304,.T.);
#3464=FACE_BOUND('',#6305,.T.);
#3465=FACE_BOUND('',#6306,.T.);
#3466=FACE_BOUND('',#6307,.T.);
#3467=FACE_BOUND('',#6308,.T.);
#3468=FACE_BOUND('',#6309,.T.);
#3469=FACE_BOUND('',#6310,.T.);
#3470=FACE_BOUND('',#6311,.T.);
#3471=FACE_BOUND('',#6312,.T.);
#3472=FACE_BOUND('',#6313,.T.);
#3473=FACE_BOUND('',#6314,.T.);
#3474=FACE_BOUND('',#6315,.T.);
#3475=FACE_BOUND('',#6316,.T.);
#3476=FACE_BOUND('',#6317,.T.);
#3477=FACE_BOUND('',#6318,.T.);
#3478=FACE_BOUND('',#6319,.T.);
#3479=FACE_BOUND('',#6320,.T.);
#3480=FACE_BOUND('',#6321,.T.);
#3481=FACE_BOUND('',#6322,.T.);
#3482=FACE_BOUND('',#6323,.T.);
#3483=FACE_BOUND('',#6326,.T.);
#4182=FACE_OUTER_BOUND('',#6099,.T.);
#4183=FACE_OUTER_BOUND('',#6100,.T.);
#4184=FACE_OUTER_BOUND('',#6101,.T.);
#4185=FACE_OUTER_BOUND('',#6102,.T.);
#4186=FACE_OUTER_BOUND('',#6103,.T.);
#4187=FACE_OUTER_BOUND('',#6104,.T.);
#4188=FACE_OUTER_BOUND('',#6105,.T.);
#4189=FACE_OUTER_BOUND('',#6106,.T.);
#4190=FACE_OUTER_BOUND('',#6107,.T.);
#4191=FACE_OUTER_BOUND('',#6108,.T.);
#4192=FACE_OUTER_BOUND('',#6109,.T.);
#4193=FACE_OUTER_BOUND('',#6110,.T.);
#4194=FACE_OUTER_BOUND('',#6111,.T.);
#4195=FACE_OUTER_BOUND('',#6112,.T.);
#4196=FACE_OUTER_BOUND('',#6113,.T.);
#4197=FACE_OUTER_BOUND('',#6114,.T.);
#4198=FACE_OUTER_BOUND('',#6115,.T.);
#4199=FACE_OUTER_BOUND('',#6116,.T.);
#4200=FACE_OUTER_BOUND('',#6117,.T.);
#4201=FACE_OUTER_BOUND('',#6118,.T.);
#4202=FACE_OUTER_BOUND('',#6119,.T.);
#4203=FACE_OUTER_BOUND('',#6120,.T.);
#4204=FACE_OUTER_BOUND('',#6121,.T.);
#4205=FACE_OUTER_BOUND('',#6122,.T.);
#4206=FACE_OUTER_BOUND('',#6123,.T.);
#4207=FACE_OUTER_BOUND('',#6124,.T.);
#4208=FACE_OUTER_BOUND('',#6125,.T.);
#4209=FACE_OUTER_BOUND('',#6126,.T.);
#4210=FACE_OUTER_BOUND('',#6127,.T.);
#4211=FACE_OUTER_BOUND('',#6128,.T.);
#4212=FACE_OUTER_BOUND('',#6129,.T.);
#4213=FACE_OUTER_BOUND('',#6130,.T.);
#4214=FACE_OUTER_BOUND('',#6131,.T.);
#4215=FACE_OUTER_BOUND('',#6132,.T.);
#4216=FACE_OUTER_BOUND('',#6133,.T.);
#4217=FACE_OUTER_BOUND('',#6134,.T.);
#4218=FACE_OUTER_BOUND('',#6135,.T.);
#4219=FACE_OUTER_BOUND('',#6136,.T.);
#4220=FACE_OUTER_BOUND('',#6137,.T.);
#4221=FACE_OUTER_BOUND('',#6138,.T.);
#4222=FACE_OUTER_BOUND('',#6139,.T.);
#4223=FACE_OUTER_BOUND('',#6140,.T.);
#4224=FACE_OUTER_BOUND('',#6141,.T.);
#4225=FACE_OUTER_BOUND('',#6142,.T.);
#4226=FACE_OUTER_BOUND('',#6143,.T.);
#4227=FACE_OUTER_BOUND('',#6144,.T.);
#4228=FACE_OUTER_BOUND('',#6145,.T.);
#4229=FACE_OUTER_BOUND('',#6146,.T.);
#4230=FACE_OUTER_BOUND('',#6147,.T.);
#4231=FACE_OUTER_BOUND('',#6148,.T.);
#4232=FACE_OUTER_BOUND('',#6149,.T.);
#4233=FACE_OUTER_BOUND('',#6150,.T.);
#4234=FACE_OUTER_BOUND('',#6151,.T.);
#4235=FACE_OUTER_BOUND('',#6152,.T.);
#4236=FACE_OUTER_BOUND('',#6153,.T.);
#4237=FACE_OUTER_BOUND('',#6154,.T.);
#4238=FACE_OUTER_BOUND('',#6155,.T.);
#4239=FACE_OUTER_BOUND('',#6156,.T.);
#4240=FACE_OUTER_BOUND('',#6157,.T.);
#4241=FACE_OUTER_BOUND('',#6158,.T.);
#4242=FACE_OUTER_BOUND('',#6159,.T.);
#4243=FACE_OUTER_BOUND('',#6160,.T.);
#4244=FACE_OUTER_BOUND('',#6161,.T.);
#4245=FACE_OUTER_BOUND('',#6162,.T.);
#4246=FACE_OUTER_BOUND('',#6163,.T.);
#4247=FACE_OUTER_BOUND('',#6164,.T.);
#4248=FACE_OUTER_BOUND('',#6165,.T.);
#4249=FACE_OUTER_BOUND('',#6166,.T.);
#4250=FACE_OUTER_BOUND('',#6167,.T.);
#4251=FACE_OUTER_BOUND('',#6168,.T.);
#4252=FACE_OUTER_BOUND('',#6169,.T.);
#4253=FACE_OUTER_BOUND('',#6170,.T.);
#4254=FACE_OUTER_BOUND('',#6171,.T.);
#4255=FACE_OUTER_BOUND('',#6172,.T.);
#4256=FACE_OUTER_BOUND('',#6173,.T.);
#4257=FACE_OUTER_BOUND('',#6174,.T.);
#4258=FACE_OUTER_BOUND('',#6175,.T.);
#4259=FACE_OUTER_BOUND('',#6176,.T.);
#4260=FACE_OUTER_BOUND('',#6177,.T.);
#4261=FACE_OUTER_BOUND('',#6178,.T.);
#4262=FACE_OUTER_BOUND('',#6179,.T.);
#4263=FACE_OUTER_BOUND('',#6180,.T.);
#4264=FACE_OUTER_BOUND('',#6181,.T.);
#4265=FACE_OUTER_BOUND('',#6182,.T.);
#4266=FACE_OUTER_BOUND('',#6183,.T.);
#4267=FACE_OUTER_BOUND('',#6184,.T.);
#4268=FACE_OUTER_BOUND('',#6185,.T.);
#4269=FACE_OUTER_BOUND('',#6186,.T.);
#4270=FACE_OUTER_BOUND('',#6187,.T.);
#4271=FACE_OUTER_BOUND('',#6188,.T.);
#4272=FACE_OUTER_BOUND('',#6189,.T.);
#4273=FACE_OUTER_BOUND('',#6190,.T.);
#4274=FACE_OUTER_BOUND('',#6191,.T.);
#4275=FACE_OUTER_BOUND('',#6192,.T.);
#4276=FACE_OUTER_BOUND('',#6193,.T.);
#4277=FACE_OUTER_BOUND('',#6194,.T.);
#4278=FACE_OUTER_BOUND('',#6195,.T.);
#4279=FACE_OUTER_BOUND('',#6196,.T.);
#4280=FACE_OUTER_BOUND('',#6197,.T.);
#4281=FACE_OUTER_BOUND('',#6198,.T.);
#4282=FACE_OUTER_BOUND('',#6199,.T.);
#4283=FACE_OUTER_BOUND('',#6200,.T.);
#4284=FACE_OUTER_BOUND('',#6201,.T.);
#4285=FACE_OUTER_BOUND('',#6202,.T.);
#4286=FACE_OUTER_BOUND('',#6203,.T.);
#4287=FACE_OUTER_BOUND('',#6204,.T.);
#4288=FACE_OUTER_BOUND('',#6205,.T.);
#4289=FACE_OUTER_BOUND('',#6206,.T.);
#4290=FACE_OUTER_BOUND('',#6207,.T.);
#4291=FACE_OUTER_BOUND('',#6208,.T.);
#4292=FACE_OUTER_BOUND('',#6209,.T.);
#4293=FACE_OUTER_BOUND('',#6210,.T.);
#4294=FACE_OUTER_BOUND('',#6211,.T.);
#4295=FACE_OUTER_BOUND('',#6212,.T.);
#4296=FACE_OUTER_BOUND('',#6213,.T.);
#4297=FACE_OUTER_BOUND('',#6214,.T.);
#4298=FACE_OUTER_BOUND('',#6215,.T.);
#4299=FACE_OUTER_BOUND('',#6216,.T.);
#4300=FACE_OUTER_BOUND('',#6217,.T.);
#4301=FACE_OUTER_BOUND('',#6218,.T.);
#4302=FACE_OUTER_BOUND('',#6219,.T.);
#4303=FACE_OUTER_BOUND('',#6220,.T.);
#4304=FACE_OUTER_BOUND('',#6221,.T.);
#4305=FACE_OUTER_BOUND('',#6222,.T.);
#4306=FACE_OUTER_BOUND('',#6223,.T.);
#4307=FACE_OUTER_BOUND('',#6224,.T.);
#4308=FACE_OUTER_BOUND('',#6225,.T.);
#4309=FACE_OUTER_BOUND('',#6226,.T.);
#4310=FACE_OUTER_BOUND('',#6227,.T.);
#4311=FACE_OUTER_BOUND('',#6228,.T.);
#4312=FACE_OUTER_BOUND('',#6229,.T.);
#4313=FACE_OUTER_BOUND('',#6230,.T.);
#4314=FACE_OUTER_BOUND('',#6231,.T.);
#4315=FACE_OUTER_BOUND('',#6232,.T.);
#4316=FACE_OUTER_BOUND('',#6233,.T.);
#4317=FACE_OUTER_BOUND('',#6234,.T.);
#4318=FACE_OUTER_BOUND('',#6235,.T.);
#4319=FACE_OUTER_BOUND('',#6236,.T.);
#4320=FACE_OUTER_BOUND('',#6237,.T.);
#4321=FACE_OUTER_BOUND('',#6238,.T.);
#4322=FACE_OUTER_BOUND('',#6239,.T.);
#4323=FACE_OUTER_BOUND('',#6240,.T.);
#4324=FACE_OUTER_BOUND('',#6241,.T.);
#4325=FACE_OUTER_BOUND('',#6242,.T.);
#4326=FACE_OUTER_BOUND('',#6243,.T.);
#4327=FACE_OUTER_BOUND('',#6244,.T.);
#4328=FACE_OUTER_BOUND('',#6245,.T.);
#4329=FACE_OUTER_BOUND('',#6246,.T.);
#4330=FACE_OUTER_BOUND('',#6247,.T.);
#4331=FACE_OUTER_BOUND('',#6248,.T.);
#4332=FACE_OUTER_BOUND('',#6249,.T.);
#4333=FACE_OUTER_BOUND('',#6250,.T.);
#4334=FACE_OUTER_BOUND('',#6251,.T.);
#4335=FACE_OUTER_BOUND('',#6252,.T.);
#4336=FACE_OUTER_BOUND('',#6253,.T.);
#4337=FACE_OUTER_BOUND('',#6254,.T.);
#4338=FACE_OUTER_BOUND('',#6255,.T.);
#4339=FACE_OUTER_BOUND('',#6256,.T.);
#4340=FACE_OUTER_BOUND('',#6257,.T.);
#4341=FACE_OUTER_BOUND('',#6258,.T.);
#4342=FACE_OUTER_BOUND('',#6259,.T.);
#4343=FACE_OUTER_BOUND('',#6260,.T.);
#4344=FACE_OUTER_BOUND('',#6261,.T.);
#4345=FACE_OUTER_BOUND('',#6262,.T.);
#4346=FACE_OUTER_BOUND('',#6263,.T.);
#4347=FACE_OUTER_BOUND('',#6264,.T.);
#4348=FACE_OUTER_BOUND('',#6265,.T.);
#4349=FACE_OUTER_BOUND('',#6266,.T.);
#4350=FACE_OUTER_BOUND('',#6267,.T.);
#4351=FACE_OUTER_BOUND('',#6268,.T.);
#4352=FACE_OUTER_BOUND('',#6269,.T.);
#4353=FACE_OUTER_BOUND('',#6270,.T.);
#4354=FACE_OUTER_BOUND('',#6271,.T.);
#4355=FACE_OUTER_BOUND('',#6272,.T.);
#4356=FACE_OUTER_BOUND('',#6273,.T.);
#4357=FACE_OUTER_BOUND('',#6274,.T.);
#4358=FACE_OUTER_BOUND('',#6275,.T.);
#4359=FACE_OUTER_BOUND('',#6277,.T.);
#4360=FACE_OUTER_BOUND('',#6278,.T.);
#4361=FACE_OUTER_BOUND('',#6279,.T.);
#4362=FACE_OUTER_BOUND('',#6281,.T.);
#4363=FACE_OUTER_BOUND('',#6282,.T.);
#4364=FACE_OUTER_BOUND('',#6283,.T.);
#4365=FACE_OUTER_BOUND('',#6284,.T.);
#4366=FACE_OUTER_BOUND('',#6285,.T.);
#4367=FACE_OUTER_BOUND('',#6286,.T.);
#4368=FACE_OUTER_BOUND('',#6288,.T.);
#4369=FACE_OUTER_BOUND('',#6324,.T.);
#4370=FACE_OUTER_BOUND('',#6325,.T.);
#6099=EDGE_LOOP('',(#22147,#22148,#22149,#22150));
#6100=EDGE_LOOP('',(#22151,#22152,#22153,#22154));
#6101=EDGE_LOOP('',(#22155,#22156,#22157,#22158));
#6102=EDGE_LOOP('',(#22159,#22160,#22161,#22162));
#6103=EDGE_LOOP('',(#22163,#22164,#22165,#22166));
#6104=EDGE_LOOP('',(#22167,#22168,#22169,#22170));
#6105=EDGE_LOOP('',(#22171,#22172,#22173,#22174));
#6106=EDGE_LOOP('',(#22175,#22176,#22177,#22178));
#6107=EDGE_LOOP('',(#22179,#22180,#22181,#22182));
#6108=EDGE_LOOP('',(#22183,#22184,#22185,#22186));
#6109=EDGE_LOOP('',(#22187,#22188,#22189,#22190));
#6110=EDGE_LOOP('',(#22191,#22192,#22193,#22194));
#6111=EDGE_LOOP('',(#22195,#22196,#22197,#22198));
#6112=EDGE_LOOP('',(#22199,#22200,#22201,#22202));
#6113=EDGE_LOOP('',(#22203,#22204,#22205,#22206));
#6114=EDGE_LOOP('',(#22207,#22208,#22209,#22210));
#6115=EDGE_LOOP('',(#22211,#22212,#22213,#22214));
#6116=EDGE_LOOP('',(#22215,#22216,#22217,#22218));
#6117=EDGE_LOOP('',(#22219,#22220,#22221,#22222));
#6118=EDGE_LOOP('',(#22223,#22224,#22225,#22226));
#6119=EDGE_LOOP('',(#22227,#22228,#22229,#22230,#22231));
#6120=EDGE_LOOP('',(#22232,#22233,#22234,#22235,#22236,#22237,#22238,#22239,
#22240,#22241,#22242,#22243,#22244,#22245,#22246,#22247,#22248,#22249,#22250,
#22251,#22252,#22253,#22254,#22255));
#6121=EDGE_LOOP('',(#22256,#22257,#22258,#22259,#22260));
#6122=EDGE_LOOP('',(#22261,#22262,#22263,#22264));
#6123=EDGE_LOOP('',(#22265,#22266,#22267,#22268,#22269,#22270,#22271,#22272,
#22273,#22274,#22275,#22276,#22277,#22278,#22279,#22280,#22281,#22282,#22283,
#22284,#22285,#22286,#22287,#22288));
#6124=EDGE_LOOP('',(#22289,#22290,#22291,#22292));
#6125=EDGE_LOOP('',(#22293,#22294,#22295));
#6126=EDGE_LOOP('',(#22296,#22297,#22298,#22299));
#6127=EDGE_LOOP('',(#22300,#22301,#22302));
#6128=EDGE_LOOP('',(#22303,#22304,#22305,#22306));
#6129=EDGE_LOOP('',(#22307,#22308,#22309));
#6130=EDGE_LOOP('',(#22310,#22311,#22312,#22313));
#6131=EDGE_LOOP('',(#22314,#22315,#22316));
#6132=EDGE_LOOP('',(#22317,#22318,#22319,#22320));
#6133=EDGE_LOOP('',(#22321,#22322,#22323));
#6134=EDGE_LOOP('',(#22324,#22325,#22326,#22327));
#6135=EDGE_LOOP('',(#22328,#22329,#22330));
#6136=EDGE_LOOP('',(#22331,#22332,#22333,#22334));
#6137=EDGE_LOOP('',(#22335,#22336,#22337));
#6138=EDGE_LOOP('',(#22338,#22339,#22340,#22341));
#6139=EDGE_LOOP('',(#22342,#22343,#22344));
#6140=EDGE_LOOP('',(#22345,#22346,#22347,#22348));
#6141=EDGE_LOOP('',(#22349,#22350,#22351));
#6142=EDGE_LOOP('',(#22352,#22353,#22354,#22355));
#6143=EDGE_LOOP('',(#22356,#22357,#22358));
#6144=EDGE_LOOP('',(#22359,#22360,#22361,#22362));
#6145=EDGE_LOOP('',(#22363,#22364,#22365));
#6146=EDGE_LOOP('',(#22366,#22367,#22368,#22369));
#6147=EDGE_LOOP('',(#22370,#22371,#22372));
#6148=EDGE_LOOP('',(#22373,#22374,#22375,#22376));
#6149=EDGE_LOOP('',(#22377,#22378,#22379));
#6150=EDGE_LOOP('',(#22380,#22381,#22382,#22383));
#6151=EDGE_LOOP('',(#22384,#22385,#22386));
#6152=EDGE_LOOP('',(#22387,#22388,#22389,#22390));
#6153=EDGE_LOOP('',(#22391,#22392,#22393));
#6154=EDGE_LOOP('',(#22394,#22395,#22396,#22397));
#6155=EDGE_LOOP('',(#22398,#22399,#22400));
#6156=EDGE_LOOP('',(#22401,#22402,#22403,#22404));
#6157=EDGE_LOOP('',(#22405,#22406,#22407));
#6158=EDGE_LOOP('',(#22408,#22409,#22410,#22411));
#6159=EDGE_LOOP('',(#22412,#22413,#22414));
#6160=EDGE_LOOP('',(#22415,#22416,#22417,#22418));
#6161=EDGE_LOOP('',(#22419,#22420,#22421));
#6162=EDGE_LOOP('',(#22422,#22423,#22424,#22425));
#6163=EDGE_LOOP('',(#22426,#22427,#22428));
#6164=EDGE_LOOP('',(#22429,#22430,#22431,#22432));
#6165=EDGE_LOOP('',(#22433,#22434,#22435));
#6166=EDGE_LOOP('',(#22436,#22437,#22438,#22439));
#6167=EDGE_LOOP('',(#22440,#22441,#22442));
#6168=EDGE_LOOP('',(#22443,#22444,#22445,#22446));
#6169=EDGE_LOOP('',(#22447,#22448,#22449));
#6170=EDGE_LOOP('',(#22450,#22451,#22452,#22453));
#6171=EDGE_LOOP('',(#22454,#22455,#22456));
#6172=EDGE_LOOP('',(#22457,#22458,#22459,#22460));
#6173=EDGE_LOOP('',(#22461,#22462,#22463));
#6174=EDGE_LOOP('',(#22464,#22465,#22466,#22467));
#6175=EDGE_LOOP('',(#22468,#22469,#22470));
#6176=EDGE_LOOP('',(#22471,#22472,#22473,#22474));
#6177=EDGE_LOOP('',(#22475,#22476,#22477));
#6178=EDGE_LOOP('',(#22478,#22479,#22480,#22481));
#6179=EDGE_LOOP('',(#22482,#22483,#22484));
#6180=EDGE_LOOP('',(#22485,#22486,#22487,#22488));
#6181=EDGE_LOOP('',(#22489,#22490,#22491));
#6182=EDGE_LOOP('',(#22492,#22493,#22494,#22495));
#6183=EDGE_LOOP('',(#22496,#22497,#22498));
#6184=EDGE_LOOP('',(#22499,#22500,#22501,#22502));
#6185=EDGE_LOOP('',(#22503,#22504,#22505));
#6186=EDGE_LOOP('',(#22506,#22507,#22508,#22509));
#6187=EDGE_LOOP('',(#22510,#22511,#22512));
#6188=EDGE_LOOP('',(#22513,#22514,#22515,#22516));
#6189=EDGE_LOOP('',(#22517,#22518,#22519));
#6190=EDGE_LOOP('',(#22520,#22521,#22522,#22523));
#6191=EDGE_LOOP('',(#22524,#22525,#22526));
#6192=EDGE_LOOP('',(#22527,#22528,#22529,#22530));
#6193=EDGE_LOOP('',(#22531,#22532,#22533,#22534));
#6194=EDGE_LOOP('',(#22535,#22536,#22537,#22538));
#6195=EDGE_LOOP('',(#22539,#22540,#22541,#22542));
#6196=EDGE_LOOP('',(#22543,#22544,#22545,#22546));
#6197=EDGE_LOOP('',(#22547,#22548,#22549));
#6198=EDGE_LOOP('',(#22550,#22551,#22552,#22553));
#6199=EDGE_LOOP('',(#22554,#22555,#22556));
#6200=EDGE_LOOP('',(#22557,#22558,#22559,#22560));
#6201=EDGE_LOOP('',(#22561,#22562,#22563));
#6202=EDGE_LOOP('',(#22564,#22565,#22566,#22567));
#6203=EDGE_LOOP('',(#22568,#22569,#22570));
#6204=EDGE_LOOP('',(#22571,#22572,#22573,#22574));
#6205=EDGE_LOOP('',(#22575,#22576,#22577));
#6206=EDGE_LOOP('',(#22578,#22579,#22580,#22581));
#6207=EDGE_LOOP('',(#22582,#22583,#22584));
#6208=EDGE_LOOP('',(#22585,#22586,#22587,#22588));
#6209=EDGE_LOOP('',(#22589,#22590,#22591));
#6210=EDGE_LOOP('',(#22592,#22593,#22594,#22595));
#6211=EDGE_LOOP('',(#22596,#22597,#22598));
#6212=EDGE_LOOP('',(#22599,#22600,#22601,#22602));
#6213=EDGE_LOOP('',(#22603,#22604,#22605));
#6214=EDGE_LOOP('',(#22606,#22607,#22608,#22609));
#6215=EDGE_LOOP('',(#22610,#22611,#22612));
#6216=EDGE_LOOP('',(#22613,#22614,#22615,#22616));
#6217=EDGE_LOOP('',(#22617,#22618,#22619));
#6218=EDGE_LOOP('',(#22620,#22621,#22622,#22623));
#6219=EDGE_LOOP('',(#22624,#22625,#22626));
#6220=EDGE_LOOP('',(#22627,#22628,#22629,#22630));
#6221=EDGE_LOOP('',(#22631,#22632,#22633));
#6222=EDGE_LOOP('',(#22634,#22635,#22636,#22637));
#6223=EDGE_LOOP('',(#22638,#22639,#22640));
#6224=EDGE_LOOP('',(#22641,#22642,#22643,#22644));
#6225=EDGE_LOOP('',(#22645,#22646,#22647));
#6226=EDGE_LOOP('',(#22648,#22649,#22650,#22651));
#6227=EDGE_LOOP('',(#22652,#22653,#22654));
#6228=EDGE_LOOP('',(#22655,#22656,#22657,#22658));
#6229=EDGE_LOOP('',(#22659,#22660,#22661));
#6230=EDGE_LOOP('',(#22662,#22663,#22664,#22665));
#6231=EDGE_LOOP('',(#22666,#22667,#22668));
#6232=EDGE_LOOP('',(#22669,#22670,#22671,#22672));
#6233=EDGE_LOOP('',(#22673,#22674,#22675));
#6234=EDGE_LOOP('',(#22676,#22677,#22678,#22679));
#6235=EDGE_LOOP('',(#22680,#22681,#22682));
#6236=EDGE_LOOP('',(#22683,#22684,#22685,#22686));
#6237=EDGE_LOOP('',(#22687,#22688,#22689));
#6238=EDGE_LOOP('',(#22690,#22691,#22692,#22693));
#6239=EDGE_LOOP('',(#22694,#22695,#22696));
#6240=EDGE_LOOP('',(#22697,#22698,#22699,#22700));
#6241=EDGE_LOOP('',(#22701,#22702,#22703));
#6242=EDGE_LOOP('',(#22704,#22705,#22706,#22707));
#6243=EDGE_LOOP('',(#22708,#22709,#22710));
#6244=EDGE_LOOP('',(#22711,#22712,#22713,#22714));
#6245=EDGE_LOOP('',(#22715,#22716,#22717));
#6246=EDGE_LOOP('',(#22718,#22719,#22720,#22721));
#6247=EDGE_LOOP('',(#22722,#22723,#22724));
#6248=EDGE_LOOP('',(#22725,#22726,#22727,#22728));
#6249=EDGE_LOOP('',(#22729,#22730,#22731));
#6250=EDGE_LOOP('',(#22732,#22733,#22734,#22735));
#6251=EDGE_LOOP('',(#22736,#22737,#22738));
#6252=EDGE_LOOP('',(#22739,#22740,#22741,#22742));
#6253=EDGE_LOOP('',(#22743,#22744,#22745));
#6254=EDGE_LOOP('',(#22746,#22747,#22748,#22749));
#6255=EDGE_LOOP('',(#22750,#22751,#22752));
#6256=EDGE_LOOP('',(#22753,#22754,#22755,#22756));
#6257=EDGE_LOOP('',(#22757,#22758,#22759));
#6258=EDGE_LOOP('',(#22760,#22761,#22762,#22763));
#6259=EDGE_LOOP('',(#22764,#22765,#22766));
#6260=EDGE_LOOP('',(#22767,#22768,#22769,#22770));
#6261=EDGE_LOOP('',(#22771,#22772,#22773));
#6262=EDGE_LOOP('',(#22774,#22775,#22776,#22777));
#6263=EDGE_LOOP('',(#22778,#22779,#22780));
#6264=EDGE_LOOP('',(#22781,#22782,#22783,#22784));
#6265=EDGE_LOOP('',(#22785,#22786,#22787));
#6266=EDGE_LOOP('',(#22788,#22789,#22790,#22791));
#6267=EDGE_LOOP('',(#22792,#22793,#22794));
#6268=EDGE_LOOP('',(#22795,#22796,#22797));
#6269=EDGE_LOOP('',(#22798,#22799,#22800,#22801));
#6270=EDGE_LOOP('',(#22802,#22803,#22804,#22805));
#6271=EDGE_LOOP('',(#22806,#22807,#22808,#22809));
#6272=EDGE_LOOP('',(#22810,#22811,#22812,#22813));
#6273=EDGE_LOOP('',(#22814,#22815,#22816,#22817));
#6274=EDGE_LOOP('',(#22818,#22819,#22820,#22821));
#6275=EDGE_LOOP('',(#22822,#22823,#22824,#22825,#22826,#22827));
#6276=EDGE_LOOP('',(#22828));
#6277=EDGE_LOOP('',(#22829,#22830,#22831,#22832,#22833));
#6278=EDGE_LOOP('',(#22834,#22835,#22836,#22837,#22838));
#6279=EDGE_LOOP('',(#22839));
#6280=EDGE_LOOP('',(#22840));
#6281=EDGE_LOOP('',(#22841));
#6282=EDGE_LOOP('',(#22842,#22843,#22844,#22845,#22846,#22847));
#6283=EDGE_LOOP('',(#22848,#22849,#22850,#22851));
#6284=EDGE_LOOP('',(#22852,#22853,#22854,#22855,#22856,#22857));
#6285=EDGE_LOOP('',(#22858,#22859,#22860,#22861));
#6286=EDGE_LOOP('',(#22862));
#6287=EDGE_LOOP('',(#22863));
#6288=EDGE_LOOP('',(#22864,#22865,#22866,#22867,#22868,#22869,#22870,#22871,
#22872,#22873,#22874,#22875));
#6289=EDGE_LOOP('',(#22876,#22877,#22878,#22879));
#6290=EDGE_LOOP('',(#22880,#22881,#22882,#22883));
#6291=EDGE_LOOP('',(#22884,#22885,#22886,#22887));
#6292=EDGE_LOOP('',(#22888,#22889,#22890,#22891));
#6293=EDGE_LOOP('',(#22892,#22893,#22894,#22895));
#6294=EDGE_LOOP('',(#22896,#22897,#22898,#22899));
#6295=EDGE_LOOP('',(#22900,#22901,#22902,#22903));
#6296=EDGE_LOOP('',(#22904,#22905,#22906,#22907));
#6297=EDGE_LOOP('',(#22908,#22909,#22910,#22911));
#6298=EDGE_LOOP('',(#22912,#22913,#22914,#22915));
#6299=EDGE_LOOP('',(#22916,#22917,#22918,#22919));
#6300=EDGE_LOOP('',(#22920,#22921,#22922,#22923));
#6301=EDGE_LOOP('',(#22924,#22925,#22926,#22927));
#6302=EDGE_LOOP('',(#22928,#22929,#22930,#22931));
#6303=EDGE_LOOP('',(#22932,#22933,#22934,#22935));
#6304=EDGE_LOOP('',(#22936,#22937,#22938,#22939));
#6305=EDGE_LOOP('',(#22940,#22941,#22942,#22943));
#6306=EDGE_LOOP('',(#22944,#22945,#22946,#22947));
#6307=EDGE_LOOP('',(#22948,#22949,#22950,#22951));
#6308=EDGE_LOOP('',(#22952,#22953,#22954,#22955));
#6309=EDGE_LOOP('',(#22956,#22957,#22958,#22959));
#6310=EDGE_LOOP('',(#22960,#22961,#22962,#22963));
#6311=EDGE_LOOP('',(#22964,#22965,#22966,#22967));
#6312=EDGE_LOOP('',(#22968,#22969,#22970,#22971));
#6313=EDGE_LOOP('',(#22972,#22973,#22974,#22975));
#6314=EDGE_LOOP('',(#22976,#22977,#22978,#22979));
#6315=EDGE_LOOP('',(#22980,#22981,#22982,#22983));
#6316=EDGE_LOOP('',(#22984,#22985,#22986,#22987));
#6317=EDGE_LOOP('',(#22988,#22989,#22990,#22991));
#6318=EDGE_LOOP('',(#22992,#22993,#22994,#22995));
#6319=EDGE_LOOP('',(#22996,#22997,#22998,#22999));
#6320=EDGE_LOOP('',(#23000,#23001,#23002,#23003));
#6321=EDGE_LOOP('',(#23004,#23005,#23006,#23007));
#6322=EDGE_LOOP('',(#23008,#23009,#23010,#23011));
#6323=EDGE_LOOP('',(#23012,#23013,#23014,#23015));
#6324=EDGE_LOOP('',(#23016,#23017,#23018,#23019));
#6325=EDGE_LOOP('',(#23020));
#6326=EDGE_LOOP('',(#23021,#23022,#23023,#23024,#23025,#23026));
#8176=LINE('',#46417,#10482);
#8177=LINE('',#46441,#10483);
#8178=LINE('',#46489,#10484);
#8179=LINE('',#46537,#10485);
#8180=LINE('',#46585,#10486);
#8181=LINE('',#46639,#10487);
#8182=LINE('',#46687,#10488);
#8183=LINE('',#46735,#10489);
#8184=LINE('',#46789,#10490);
#8185=LINE('',#46837,#10491);
#8186=LINE('',#46885,#10492);
#8187=LINE('',#46901,#10493);
#8188=LINE('',#46925,#10494);
#8189=LINE('',#46949,#10495);
#8190=LINE('',#46974,#10496);
#8191=LINE('',#46999,#10497);
#8192=LINE('',#47023,#10498);
#8193=LINE('',#47048,#10499);
#8194=LINE('',#47073,#10500);
#8195=LINE('',#47097,#10501);
#8196=LINE('',#48105,#10502);
#8197=LINE('',#48107,#10503);
#8198=LINE('',#48109,#10504);
#8199=LINE('',#48110,#10505);
#8200=LINE('',#48114,#10506);
#8201=LINE('',#48117,#10507);
#8202=LINE('',#48118,#10508);
#8203=LINE('',#48124,#10509);
#8204=LINE('',#48126,#10510);
#8205=LINE('',#48128,#10511);
#8206=LINE('',#48129,#10512);
#8207=LINE('',#48133,#10513);
#8208=LINE('',#48136,#10514);
#8209=LINE('',#48137,#10515);
#8210=LINE('',#48143,#10516);
#8211=LINE('',#48145,#10517);
#8212=LINE('',#48147,#10518);
#8213=LINE('',#48148,#10519);
#8214=LINE('',#48152,#10520);
#8215=LINE('',#48155,#10521);
#8216=LINE('',#48156,#10522);
#8217=LINE('',#48162,#10523);
#8218=LINE('',#48164,#10524);
#8219=LINE('',#48166,#10525);
#8220=LINE('',#48167,#10526);
#8221=LINE('',#48171,#10527);
#8222=LINE('',#48174,#10528);
#8223=LINE('',#48175,#10529);
#8224=LINE('',#48181,#10530);
#8225=LINE('',#48183,#10531);
#8226=LINE('',#48185,#10532);
#8227=LINE('',#48186,#10533);
#8228=LINE('',#48190,#10534);
#8229=LINE('',#48193,#10535);
#8230=LINE('',#48194,#10536);
#8231=LINE('',#48200,#10537);
#8232=LINE('',#48202,#10538);
#8233=LINE('',#48204,#10539);
#8234=LINE('',#48205,#10540);
#8235=LINE('',#48209,#10541);
#8236=LINE('',#48212,#10542);
#8237=LINE('',#48213,#10543);
#8238=LINE('',#48219,#10544);
#8239=LINE('',#48221,#10545);
#8240=LINE('',#48223,#10546);
#8241=LINE('',#48224,#10547);
#8242=LINE('',#48228,#10548);
#8243=LINE('',#48231,#10549);
#8244=LINE('',#48232,#10550);
#8245=LINE('',#48238,#10551);
#8246=LINE('',#48240,#10552);
#8247=LINE('',#48242,#10553);
#8248=LINE('',#48243,#10554);
#8249=LINE('',#48247,#10555);
#8250=LINE('',#48250,#10556);
#8251=LINE('',#48251,#10557);
#8252=LINE('',#48257,#10558);
#8253=LINE('',#48259,#10559);
#8254=LINE('',#48261,#10560);
#8255=LINE('',#48262,#10561);
#8256=LINE('',#48266,#10562);
#8257=LINE('',#48269,#10563);
#8258=LINE('',#48270,#10564);
#8259=LINE('',#48276,#10565);
#8260=LINE('',#48278,#10566);
#8261=LINE('',#48280,#10567);
#8262=LINE('',#48281,#10568);
#8263=LINE('',#48285,#10569);
#8264=LINE('',#48288,#10570);
#8265=LINE('',#48289,#10571);
#8266=LINE('',#48295,#10572);
#8267=LINE('',#48297,#10573);
#8268=LINE('',#48299,#10574);
#8269=LINE('',#48300,#10575);
#8270=LINE('',#48304,#10576);
#8271=LINE('',#48307,#10577);
#8272=LINE('',#48308,#10578);
#8273=LINE('',#48314,#10579);
#8274=LINE('',#48316,#10580);
#8275=LINE('',#48318,#10581);
#8276=LINE('',#48319,#10582);
#8277=LINE('',#48323,#10583);
#8278=LINE('',#48326,#10584);
#8279=LINE('',#48327,#10585);
#8280=LINE('',#48333,#10586);
#8281=LINE('',#48335,#10587);
#8282=LINE('',#48337,#10588);
#8283=LINE('',#48338,#10589);
#8284=LINE('',#48342,#10590);
#8285=LINE('',#48345,#10591);
#8286=LINE('',#48346,#10592);
#8287=LINE('',#48352,#10593);
#8288=LINE('',#48354,#10594);
#8289=LINE('',#48356,#10595);
#8290=LINE('',#48357,#10596);
#8291=LINE('',#48361,#10597);
#8292=LINE('',#48364,#10598);
#8293=LINE('',#48365,#10599);
#8294=LINE('',#48371,#10600);
#8295=LINE('',#48373,#10601);
#8296=LINE('',#48375,#10602);
#8297=LINE('',#48376,#10603);
#8298=LINE('',#48380,#10604);
#8299=LINE('',#48383,#10605);
#8300=LINE('',#48384,#10606);
#8301=LINE('',#48390,#10607);
#8302=LINE('',#48392,#10608);
#8303=LINE('',#48394,#10609);
#8304=LINE('',#48395,#10610);
#8305=LINE('',#48399,#10611);
#8306=LINE('',#48402,#10612);
#8307=LINE('',#48403,#10613);
#8308=LINE('',#48409,#10614);
#8309=LINE('',#48411,#10615);
#8310=LINE('',#48413,#10616);
#8311=LINE('',#48414,#10617);
#8312=LINE('',#48418,#10618);
#8313=LINE('',#48421,#10619);
#8314=LINE('',#48422,#10620);
#8315=LINE('',#48428,#10621);
#8316=LINE('',#48430,#10622);
#8317=LINE('',#48432,#10623);
#8318=LINE('',#48433,#10624);
#8319=LINE('',#48438,#10625);
#8320=LINE('',#48442,#10626);
#8321=LINE('',#48443,#10627);
#8322=LINE('',#48451,#10628);
#8323=LINE('',#48453,#10629);
#8324=LINE('',#48455,#10630);
#8325=LINE('',#48456,#10631);
#8326=LINE('',#48460,#10632);
#8327=LINE('',#48463,#10633);
#8328=LINE('',#48464,#10634);
#8329=LINE('',#48470,#10635);
#8330=LINE('',#48472,#10636);
#8331=LINE('',#48474,#10637);
#8332=LINE('',#48475,#10638);
#8333=LINE('',#48479,#10639);
#8334=LINE('',#48482,#10640);
#8335=LINE('',#48483,#10641);
#8336=LINE('',#48489,#10642);
#8337=LINE('',#48491,#10643);
#8338=LINE('',#48493,#10644);
#8339=LINE('',#48494,#10645);
#8340=LINE('',#48498,#10646);
#8341=LINE('',#48501,#10647);
#8342=LINE('',#48502,#10648);
#8343=LINE('',#48508,#10649);
#8344=LINE('',#48510,#10650);
#8345=LINE('',#48512,#10651);
#8346=LINE('',#48513,#10652);
#8347=LINE('',#48517,#10653);
#8348=LINE('',#48520,#10654);
#8349=LINE('',#48521,#10655);
#8350=LINE('',#48527,#10656);
#8351=LINE('',#48529,#10657);
#8352=LINE('',#48531,#10658);
#8353=LINE('',#48532,#10659);
#8354=LINE('',#48536,#10660);
#8355=LINE('',#48539,#10661);
#8356=LINE('',#48540,#10662);
#8357=LINE('',#48546,#10663);
#8358=LINE('',#48548,#10664);
#8359=LINE('',#48550,#10665);
#8360=LINE('',#48551,#10666);
#8361=LINE('',#48555,#10667);
#8362=LINE('',#48558,#10668);
#8363=LINE('',#48559,#10669);
#8364=LINE('',#48565,#10670);
#8365=LINE('',#48567,#10671);
#8366=LINE('',#48569,#10672);
#8367=LINE('',#48570,#10673);
#8368=LINE('',#48574,#10674);
#8369=LINE('',#48577,#10675);
#8370=LINE('',#48578,#10676);
#8371=LINE('',#48584,#10677);
#8372=LINE('',#48586,#10678);
#8373=LINE('',#48588,#10679);
#8374=LINE('',#48589,#10680);
#8375=LINE('',#48593,#10681);
#8376=LINE('',#48596,#10682);
#8377=LINE('',#48597,#10683);
#8378=LINE('',#48603,#10684);
#8379=LINE('',#48605,#10685);
#8380=LINE('',#48607,#10686);
#8381=LINE('',#48608,#10687);
#8382=LINE('',#48612,#10688);
#8383=LINE('',#48615,#10689);
#8384=LINE('',#48616,#10690);
#8385=LINE('',#48622,#10691);
#8386=LINE('',#48624,#10692);
#8387=LINE('',#48626,#10693);
#8388=LINE('',#48627,#10694);
#8389=LINE('',#48631,#10695);
#8390=LINE('',#48634,#10696);
#8391=LINE('',#48635,#10697);
#8392=LINE('',#48641,#10698);
#8393=LINE('',#48643,#10699);
#8394=LINE('',#48645,#10700);
#8395=LINE('',#48646,#10701);
#8396=LINE('',#48650,#10702);
#8397=LINE('',#48653,#10703);
#8398=LINE('',#48654,#10704);
#8399=LINE('',#48660,#10705);
#8400=LINE('',#48662,#10706);
#8401=LINE('',#48664,#10707);
#8402=LINE('',#48665,#10708);
#8403=LINE('',#48669,#10709);
#8404=LINE('',#48672,#10710);
#8405=LINE('',#48673,#10711);
#8406=LINE('',#48679,#10712);
#8407=LINE('',#48681,#10713);
#8408=LINE('',#48683,#10714);
#8409=LINE('',#48684,#10715);
#8410=LINE('',#48688,#10716);
#8411=LINE('',#48691,#10717);
#8412=LINE('',#48692,#10718);
#8413=LINE('',#48698,#10719);
#8414=LINE('',#48700,#10720);
#8415=LINE('',#48702,#10721);
#8416=LINE('',#48703,#10722);
#8417=LINE('',#48707,#10723);
#8418=LINE('',#48710,#10724);
#8419=LINE('',#48711,#10725);
#8420=LINE('',#48717,#10726);
#8421=LINE('',#48719,#10727);
#8422=LINE('',#48721,#10728);
#8423=LINE('',#48722,#10729);
#8424=LINE('',#48726,#10730);
#8425=LINE('',#48729,#10731);
#8426=LINE('',#48730,#10732);
#8427=LINE('',#48736,#10733);
#8428=LINE('',#48738,#10734);
#8429=LINE('',#48740,#10735);
#8430=LINE('',#48741,#10736);
#8431=LINE('',#48745,#10737);
#8432=LINE('',#48748,#10738);
#8433=LINE('',#48749,#10739);
#8434=LINE('',#48755,#10740);
#8435=LINE('',#48757,#10741);
#8436=LINE('',#48759,#10742);
#8437=LINE('',#48760,#10743);
#8438=LINE('',#48764,#10744);
#8439=LINE('',#48767,#10745);
#8440=LINE('',#48768,#10746);
#8441=LINE('',#48774,#10747);
#8442=LINE('',#48776,#10748);
#8443=LINE('',#48778,#10749);
#8444=LINE('',#48779,#10750);
#8445=LINE('',#48783,#10751);
#8446=LINE('',#48786,#10752);
#8447=LINE('',#48787,#10753);
#8448=LINE('',#48793,#10754);
#8449=LINE('',#48798,#10755);
#8450=LINE('',#48800,#10756);
#8451=LINE('',#48802,#10757);
#8452=LINE('',#48803,#10758);
#8453=LINE('',#48806,#10759);
#8454=LINE('',#48808,#10760);
#8455=LINE('',#48809,#10761);
#8456=LINE('',#48812,#10762);
#8457=LINE('',#48814,#10763);
#8458=LINE('',#48815,#10764);
#8459=LINE('',#48818,#10765);
#8460=LINE('',#48820,#10766);
#8461=LINE('',#48821,#10767);
#8462=LINE('',#48824,#10768);
#8463=LINE('',#48826,#10769);
#8464=LINE('',#48827,#10770);
#8465=LINE('',#48829,#10771);
#8466=LINE('',#48830,#10772);
#8467=LINE('',#48842,#10773);
#8468=LINE('',#48851,#10774);
#8469=LINE('',#48857,#10775);
#8470=LINE('',#48861,#10776);
#8471=LINE('',#48866,#10777);
#8472=LINE('',#48867,#10778);
#8473=LINE('',#48871,#10779);
#10482=VECTOR('',#35999,4.);
#10483=VECTOR('',#36004,4.);
#10484=VECTOR('',#36007,4.);
#10485=VECTOR('',#36010,4.);
#10486=VECTOR('',#36013,4.);
#10487=VECTOR('',#36016,4.);
#10488=VECTOR('',#36019,4.);
#10489=VECTOR('',#36022,4.);
#10490=VECTOR('',#36025,4.);
#10491=VECTOR('',#36028,4.);
#10492=VECTOR('',#36031,3.22275);
#10493=VECTOR('',#36036,3.22275);
#10494=VECTOR('',#36039,3.22275);
#10495=VECTOR('',#36042,3.22275);
#10496=VECTOR('',#36045,3.22275);
#10497=VECTOR('',#36048,3.22275);
#10498=VECTOR('',#36051,3.22275);
#10499=VECTOR('',#36054,3.22275);
#10500=VECTOR('',#36057,3.22275);
#10501=VECTOR('',#36060,3.22275);
#10502=VECTOR('',#36079,10.);
#10503=VECTOR('',#36080,10.);
#10504=VECTOR('',#36081,10.);
#10505=VECTOR('',#36082,10.);
#10506=VECTOR('',#36087,10.);
#10507=VECTOR('',#36090,10.);
#10508=VECTOR('',#36091,10.);
#10509=VECTOR('',#36098,10.);
#10510=VECTOR('',#36099,10.);
#10511=VECTOR('',#36100,10.);
#10512=VECTOR('',#36101,10.);
#10513=VECTOR('',#36106,10.);
#10514=VECTOR('',#36109,10.);
#10515=VECTOR('',#36110,10.);
#10516=VECTOR('',#36117,10.);
#10517=VECTOR('',#36118,10.);
#10518=VECTOR('',#36119,10.);
#10519=VECTOR('',#36120,10.);
#10520=VECTOR('',#36125,10.);
#10521=VECTOR('',#36128,10.);
#10522=VECTOR('',#36129,10.);
#10523=VECTOR('',#36136,10.);
#10524=VECTOR('',#36137,10.);
#10525=VECTOR('',#36138,10.);
#10526=VECTOR('',#36139,10.);
#10527=VECTOR('',#36144,10.);
#10528=VECTOR('',#36147,10.);
#10529=VECTOR('',#36148,10.);
#10530=VECTOR('',#36155,10.);
#10531=VECTOR('',#36156,10.);
#10532=VECTOR('',#36157,10.);
#10533=VECTOR('',#36158,10.);
#10534=VECTOR('',#36163,10.);
#10535=VECTOR('',#36166,10.);
#10536=VECTOR('',#36167,10.);
#10537=VECTOR('',#36174,10.);
#10538=VECTOR('',#36175,10.);
#10539=VECTOR('',#36176,10.);
#10540=VECTOR('',#36177,10.);
#10541=VECTOR('',#36182,10.);
#10542=VECTOR('',#36185,10.);
#10543=VECTOR('',#36186,10.);
#10544=VECTOR('',#36193,10.);
#10545=VECTOR('',#36194,10.);
#10546=VECTOR('',#36195,10.);
#10547=VECTOR('',#36196,10.);
#10548=VECTOR('',#36201,10.);
#10549=VECTOR('',#36204,10.);
#10550=VECTOR('',#36205,10.);
#10551=VECTOR('',#36212,10.);
#10552=VECTOR('',#36213,10.);
#10553=VECTOR('',#36214,10.);
#10554=VECTOR('',#36215,10.);
#10555=VECTOR('',#36220,10.);
#10556=VECTOR('',#36223,10.);
#10557=VECTOR('',#36224,10.);
#10558=VECTOR('',#36231,10.);
#10559=VECTOR('',#36232,10.);
#10560=VECTOR('',#36233,10.);
#10561=VECTOR('',#36234,10.);
#10562=VECTOR('',#36239,10.);
#10563=VECTOR('',#36242,10.);
#10564=VECTOR('',#36243,10.);
#10565=VECTOR('',#36250,10.);
#10566=VECTOR('',#36251,10.);
#10567=VECTOR('',#36252,10.);
#10568=VECTOR('',#36253,10.);
#10569=VECTOR('',#36258,10.);
#10570=VECTOR('',#36261,10.);
#10571=VECTOR('',#36262,10.);
#10572=VECTOR('',#36269,10.);
#10573=VECTOR('',#36270,10.);
#10574=VECTOR('',#36271,10.);
#10575=VECTOR('',#36272,10.);
#10576=VECTOR('',#36277,10.);
#10577=VECTOR('',#36280,10.);
#10578=VECTOR('',#36281,10.);
#10579=VECTOR('',#36288,10.);
#10580=VECTOR('',#36289,10.);
#10581=VECTOR('',#36290,10.);
#10582=VECTOR('',#36291,10.);
#10583=VECTOR('',#36296,10.);
#10584=VECTOR('',#36299,10.);
#10585=VECTOR('',#36300,10.);
#10586=VECTOR('',#36307,10.);
#10587=VECTOR('',#36308,10.);
#10588=VECTOR('',#36309,10.);
#10589=VECTOR('',#36310,10.);
#10590=VECTOR('',#36315,10.);
#10591=VECTOR('',#36318,10.);
#10592=VECTOR('',#36319,10.);
#10593=VECTOR('',#36326,10.);
#10594=VECTOR('',#36327,10.);
#10595=VECTOR('',#36328,10.);
#10596=VECTOR('',#36329,10.);
#10597=VECTOR('',#36334,10.);
#10598=VECTOR('',#36337,10.);
#10599=VECTOR('',#36338,10.);
#10600=VECTOR('',#36345,10.);
#10601=VECTOR('',#36346,10.);
#10602=VECTOR('',#36347,10.);
#10603=VECTOR('',#36348,10.);
#10604=VECTOR('',#36353,10.);
#10605=VECTOR('',#36356,10.);
#10606=VECTOR('',#36357,10.);
#10607=VECTOR('',#36364,10.);
#10608=VECTOR('',#36365,10.);
#10609=VECTOR('',#36366,10.);
#10610=VECTOR('',#36367,10.);
#10611=VECTOR('',#36372,10.);
#10612=VECTOR('',#36375,10.);
#10613=VECTOR('',#36376,10.);
#10614=VECTOR('',#36383,10.);
#10615=VECTOR('',#36384,10.);
#10616=VECTOR('',#36385,10.);
#10617=VECTOR('',#36386,10.);
#10618=VECTOR('',#36391,10.);
#10619=VECTOR('',#36394,10.);
#10620=VECTOR('',#36395,10.);
#10621=VECTOR('',#36402,10.);
#10622=VECTOR('',#36403,10.);
#10623=VECTOR('',#36404,10.);
#10624=VECTOR('',#36405,10.);
#10625=VECTOR('',#36410,10.);
#10626=VECTOR('',#36415,10.);
#10627=VECTOR('',#36416,10.);
#10628=VECTOR('',#36425,10.);
#10629=VECTOR('',#36426,10.);
#10630=VECTOR('',#36427,10.);
#10631=VECTOR('',#36428,10.);
#10632=VECTOR('',#36433,10.);
#10633=VECTOR('',#36436,10.);
#10634=VECTOR('',#36437,10.);
#10635=VECTOR('',#36444,10.);
#10636=VECTOR('',#36445,10.);
#10637=VECTOR('',#36446,10.);
#10638=VECTOR('',#36447,10.);
#10639=VECTOR('',#36452,10.);
#10640=VECTOR('',#36455,10.);
#10641=VECTOR('',#36456,10.);
#10642=VECTOR('',#36463,10.);
#10643=VECTOR('',#36464,10.);
#10644=VECTOR('',#36465,10.);
#10645=VECTOR('',#36466,10.);
#10646=VECTOR('',#36471,10.);
#10647=VECTOR('',#36474,10.);
#10648=VECTOR('',#36475,10.);
#10649=VECTOR('',#36482,10.);
#10650=VECTOR('',#36483,10.);
#10651=VECTOR('',#36484,10.);
#10652=VECTOR('',#36485,10.);
#10653=VECTOR('',#36490,10.);
#10654=VECTOR('',#36493,10.);
#10655=VECTOR('',#36494,10.);
#10656=VECTOR('',#36501,10.);
#10657=VECTOR('',#36502,10.);
#10658=VECTOR('',#36503,10.);
#10659=VECTOR('',#36504,10.);
#10660=VECTOR('',#36509,10.);
#10661=VECTOR('',#36512,10.);
#10662=VECTOR('',#36513,10.);
#10663=VECTOR('',#36520,10.);
#10664=VECTOR('',#36521,10.);
#10665=VECTOR('',#36522,10.);
#10666=VECTOR('',#36523,10.);
#10667=VECTOR('',#36528,10.);
#10668=VECTOR('',#36531,10.);
#10669=VECTOR('',#36532,10.);
#10670=VECTOR('',#36539,10.);
#10671=VECTOR('',#36540,10.);
#10672=VECTOR('',#36541,10.);
#10673=VECTOR('',#36542,10.);
#10674=VECTOR('',#36547,10.);
#10675=VECTOR('',#36550,10.);
#10676=VECTOR('',#36551,10.);
#10677=VECTOR('',#36558,10.);
#10678=VECTOR('',#36559,10.);
#10679=VECTOR('',#36560,10.);
#10680=VECTOR('',#36561,10.);
#10681=VECTOR('',#36566,10.);
#10682=VECTOR('',#36569,10.);
#10683=VECTOR('',#36570,10.);
#10684=VECTOR('',#36577,10.);
#10685=VECTOR('',#36578,10.);
#10686=VECTOR('',#36579,10.);
#10687=VECTOR('',#36580,10.);
#10688=VECTOR('',#36585,10.);
#10689=VECTOR('',#36588,10.);
#10690=VECTOR('',#36589,10.);
#10691=VECTOR('',#36596,10.);
#10692=VECTOR('',#36597,10.);
#10693=VECTOR('',#36598,10.);
#10694=VECTOR('',#36599,10.);
#10695=VECTOR('',#36604,10.);
#10696=VECTOR('',#36607,10.);
#10697=VECTOR('',#36608,10.);
#10698=VECTOR('',#36615,10.);
#10699=VECTOR('',#36616,10.);
#10700=VECTOR('',#36617,10.);
#10701=VECTOR('',#36618,10.);
#10702=VECTOR('',#36623,10.);
#10703=VECTOR('',#36626,10.);
#10704=VECTOR('',#36627,10.);
#10705=VECTOR('',#36634,10.);
#10706=VECTOR('',#36635,10.);
#10707=VECTOR('',#36636,10.);
#10708=VECTOR('',#36637,10.);
#10709=VECTOR('',#36642,10.);
#10710=VECTOR('',#36645,10.);
#10711=VECTOR('',#36646,10.);
#10712=VECTOR('',#36653,10.);
#10713=VECTOR('',#36654,10.);
#10714=VECTOR('',#36655,10.);
#10715=VECTOR('',#36656,10.);
#10716=VECTOR('',#36661,10.);
#10717=VECTOR('',#36664,10.);
#10718=VECTOR('',#36665,10.);
#10719=VECTOR('',#36672,10.);
#10720=VECTOR('',#36673,10.);
#10721=VECTOR('',#36674,10.);
#10722=VECTOR('',#36675,10.);
#10723=VECTOR('',#36680,10.);
#10724=VECTOR('',#36683,10.);
#10725=VECTOR('',#36684,10.);
#10726=VECTOR('',#36691,10.);
#10727=VECTOR('',#36692,10.);
#10728=VECTOR('',#36693,10.);
#10729=VECTOR('',#36694,10.);
#10730=VECTOR('',#36699,10.);
#10731=VECTOR('',#36702,10.);
#10732=VECTOR('',#36703,10.);
#10733=VECTOR('',#36710,10.);
#10734=VECTOR('',#36711,10.);
#10735=VECTOR('',#36712,10.);
#10736=VECTOR('',#36713,10.);
#10737=VECTOR('',#36718,10.);
#10738=VECTOR('',#36721,10.);
#10739=VECTOR('',#36722,10.);
#10740=VECTOR('',#36729,10.);
#10741=VECTOR('',#36730,10.);
#10742=VECTOR('',#36731,10.);
#10743=VECTOR('',#36732,10.);
#10744=VECTOR('',#36737,10.);
#10745=VECTOR('',#36740,10.);
#10746=VECTOR('',#36741,10.);
#10747=VECTOR('',#36748,10.);
#10748=VECTOR('',#36749,10.);
#10749=VECTOR('',#36750,10.);
#10750=VECTOR('',#36751,10.);
#10751=VECTOR('',#36756,10.);
#10752=VECTOR('',#36759,10.);
#10753=VECTOR('',#36760,10.);
#10754=VECTOR('',#36767,1.25);
#10755=VECTOR('',#36772,10.);
#10756=VECTOR('',#36773,10.);
#10757=VECTOR('',#36774,10.);
#10758=VECTOR('',#36775,10.);
#10759=VECTOR('',#36778,10.);
#10760=VECTOR('',#36779,10.);
#10761=VECTOR('',#36780,10.);
#10762=VECTOR('',#36783,10.);
#10763=VECTOR('',#36784,10.);
#10764=VECTOR('',#36785,10.);
#10765=VECTOR('',#36788,10.);
#10766=VECTOR('',#36789,10.);
#10767=VECTOR('',#36790,10.);
#10768=VECTOR('',#36793,10.);
#10769=VECTOR('',#36794,10.);
#10770=VECTOR('',#36795,10.);
#10771=VECTOR('',#36798,10.);
#10772=VECTOR('',#36799,10.);
#10773=VECTOR('',#36814,5.);
#10774=VECTOR('',#36827,3.6);
#10775=VECTOR('',#36836,3.625);
#10776=VECTOR('',#36841,3.25);
#10777=VECTOR('',#36848,8.);
#10778=VECTOR('',#36849,8.);
#10779=VECTOR('',#36854,7.75);
#12883=VERTEX_POINT('',#46415);
#12884=VERTEX_POINT('',#46416);
#12885=VERTEX_POINT('',#46418);
#12886=VERTEX_POINT('',#46429);
#12887=VERTEX_POINT('',#46439);
#12888=VERTEX_POINT('',#46440);
#12889=VERTEX_POINT('',#46487);
#12890=VERTEX_POINT('',#46488);
#12891=VERTEX_POINT('',#46535);
#12892=VERTEX_POINT('',#46536);
#12893=VERTEX_POINT('',#46583);
#12894=VERTEX_POINT('',#46584);
#12895=VERTEX_POINT('',#46637);
#12896=VERTEX_POINT('',#46638);
#12897=VERTEX_POINT('',#46685);
#12898=VERTEX_POINT('',#46686);
#12899=VERTEX_POINT('',#46733);
#12900=VERTEX_POINT('',#46734);
#12901=VERTEX_POINT('',#46787);
#12902=VERTEX_POINT('',#46788);
#12903=VERTEX_POINT('',#46835);
#12904=VERTEX_POINT('',#46836);
#12905=VERTEX_POINT('',#46883);
#12906=VERTEX_POINT('',#46884);
#12907=VERTEX_POINT('',#46886);
#12908=VERTEX_POINT('',#46892);
#12909=VERTEX_POINT('',#46899);
#12910=VERTEX_POINT('',#46900);
#12911=VERTEX_POINT('',#46923);
#12912=VERTEX_POINT('',#46924);
#12913=VERTEX_POINT('',#46947);
#12914=VERTEX_POINT('',#46948);
#12915=VERTEX_POINT('',#46972);
#12916=VERTEX_POINT('',#46973);
#12917=VERTEX_POINT('',#46997);
#12918=VERTEX_POINT('',#46998);
#12919=VERTEX_POINT('',#47021);
#12920=VERTEX_POINT('',#47022);
#12921=VERTEX_POINT('',#47046);
#12922=VERTEX_POINT('',#47047);
#12923=VERTEX_POINT('',#47071);
#12924=VERTEX_POINT('',#47072);
#12925=VERTEX_POINT('',#47095);
#12926=VERTEX_POINT('',#47096);
#12927=VERTEX_POINT('',#47119);
#12928=VERTEX_POINT('',#47217);
#12929=VERTEX_POINT('',#47219);
#12930=VERTEX_POINT('',#47602);
#12931=VERTEX_POINT('',#47710);
#12932=VERTEX_POINT('',#47713);
#12933=VERTEX_POINT('',#48103);
#12934=VERTEX_POINT('',#48104);
#12935=VERTEX_POINT('',#48106);
#12936=VERTEX_POINT('',#48108);
#12937=VERTEX_POINT('',#48112);
#12938=VERTEX_POINT('',#48116);
#12939=VERTEX_POINT('',#48122);
#12940=VERTEX_POINT('',#48123);
#12941=VERTEX_POINT('',#48125);
#12942=VERTEX_POINT('',#48127);
#12943=VERTEX_POINT('',#48131);
#12944=VERTEX_POINT('',#48135);
#12945=VERTEX_POINT('',#48141);
#12946=VERTEX_POINT('',#48142);
#12947=VERTEX_POINT('',#48144);
#12948=VERTEX_POINT('',#48146);
#12949=VERTEX_POINT('',#48150);
#12950=VERTEX_POINT('',#48154);
#12951=VERTEX_POINT('',#48160);
#12952=VERTEX_POINT('',#48161);
#12953=VERTEX_POINT('',#48163);
#12954=VERTEX_POINT('',#48165);
#12955=VERTEX_POINT('',#48169);
#12956=VERTEX_POINT('',#48173);
#12957=VERTEX_POINT('',#48179);
#12958=VERTEX_POINT('',#48180);
#12959=VERTEX_POINT('',#48182);
#12960=VERTEX_POINT('',#48184);
#12961=VERTEX_POINT('',#48188);
#12962=VERTEX_POINT('',#48192);
#12963=VERTEX_POINT('',#48198);
#12964=VERTEX_POINT('',#48199);
#12965=VERTEX_POINT('',#48201);
#12966=VERTEX_POINT('',#48203);
#12967=VERTEX_POINT('',#48207);
#12968=VERTEX_POINT('',#48211);
#12969=VERTEX_POINT('',#48217);
#12970=VERTEX_POINT('',#48218);
#12971=VERTEX_POINT('',#48220);
#12972=VERTEX_POINT('',#48222);
#12973=VERTEX_POINT('',#48226);
#12974=VERTEX_POINT('',#48230);
#12975=VERTEX_POINT('',#48236);
#12976=VERTEX_POINT('',#48237);
#12977=VERTEX_POINT('',#48239);
#12978=VERTEX_POINT('',#48241);
#12979=VERTEX_POINT('',#48245);
#12980=VERTEX_POINT('',#48249);
#12981=VERTEX_POINT('',#48255);
#12982=VERTEX_POINT('',#48256);
#12983=VERTEX_POINT('',#48258);
#12984=VERTEX_POINT('',#48260);
#12985=VERTEX_POINT('',#48264);
#12986=VERTEX_POINT('',#48268);
#12987=VERTEX_POINT('',#48274);
#12988=VERTEX_POINT('',#48275);
#12989=VERTEX_POINT('',#48277);
#12990=VERTEX_POINT('',#48279);
#12991=VERTEX_POINT('',#48283);
#12992=VERTEX_POINT('',#48287);
#12993=VERTEX_POINT('',#48293);
#12994=VERTEX_POINT('',#48294);
#12995=VERTEX_POINT('',#48296);
#12996=VERTEX_POINT('',#48298);
#12997=VERTEX_POINT('',#48302);
#12998=VERTEX_POINT('',#48306);
#12999=VERTEX_POINT('',#48312);
#13000=VERTEX_POINT('',#48313);
#13001=VERTEX_POINT('',#48315);
#13002=VERTEX_POINT('',#48317);
#13003=VERTEX_POINT('',#48321);
#13004=VERTEX_POINT('',#48325);
#13005=VERTEX_POINT('',#48331);
#13006=VERTEX_POINT('',#48332);
#13007=VERTEX_POINT('',#48334);
#13008=VERTEX_POINT('',#48336);
#13009=VERTEX_POINT('',#48340);
#13010=VERTEX_POINT('',#48344);
#13011=VERTEX_POINT('',#48350);
#13012=VERTEX_POINT('',#48351);
#13013=VERTEX_POINT('',#48353);
#13014=VERTEX_POINT('',#48355);
#13015=VERTEX_POINT('',#48359);
#13016=VERTEX_POINT('',#48363);
#13017=VERTEX_POINT('',#48369);
#13018=VERTEX_POINT('',#48370);
#13019=VERTEX_POINT('',#48372);
#13020=VERTEX_POINT('',#48374);
#13021=VERTEX_POINT('',#48378);
#13022=VERTEX_POINT('',#48382);
#13023=VERTEX_POINT('',#48388);
#13024=VERTEX_POINT('',#48389);
#13025=VERTEX_POINT('',#48391);
#13026=VERTEX_POINT('',#48393);
#13027=VERTEX_POINT('',#48397);
#13028=VERTEX_POINT('',#48401);
#13029=VERTEX_POINT('',#48407);
#13030=VERTEX_POINT('',#48408);
#13031=VERTEX_POINT('',#48410);
#13032=VERTEX_POINT('',#48412);
#13033=VERTEX_POINT('',#48416);
#13034=VERTEX_POINT('',#48420);
#13035=VERTEX_POINT('',#48426);
#13036=VERTEX_POINT('',#48427);
#13037=VERTEX_POINT('',#48429);
#13038=VERTEX_POINT('',#48431);
#13039=VERTEX_POINT('',#48435);
#13040=VERTEX_POINT('',#48437);
#13041=VERTEX_POINT('',#48441);
#13042=VERTEX_POINT('',#48445);
#13043=VERTEX_POINT('',#48449);
#13044=VERTEX_POINT('',#48450);
#13045=VERTEX_POINT('',#48452);
#13046=VERTEX_POINT('',#48454);
#13047=VERTEX_POINT('',#48458);
#13048=VERTEX_POINT('',#48462);
#13049=VERTEX_POINT('',#48468);
#13050=VERTEX_POINT('',#48469);
#13051=VERTEX_POINT('',#48471);
#13052=VERTEX_POINT('',#48473);
#13053=VERTEX_POINT('',#48477);
#13054=VERTEX_POINT('',#48481);
#13055=VERTEX_POINT('',#48487);
#13056=VERTEX_POINT('',#48488);
#13057=VERTEX_POINT('',#48490);
#13058=VERTEX_POINT('',#48492);
#13059=VERTEX_POINT('',#48496);
#13060=VERTEX_POINT('',#48500);
#13061=VERTEX_POINT('',#48506);
#13062=VERTEX_POINT('',#48507);
#13063=VERTEX_POINT('',#48509);
#13064=VERTEX_POINT('',#48511);
#13065=VERTEX_POINT('',#48515);
#13066=VERTEX_POINT('',#48519);
#13067=VERTEX_POINT('',#48525);
#13068=VERTEX_POINT('',#48526);
#13069=VERTEX_POINT('',#48528);
#13070=VERTEX_POINT('',#48530);
#13071=VERTEX_POINT('',#48534);
#13072=VERTEX_POINT('',#48538);
#13073=VERTEX_POINT('',#48544);
#13074=VERTEX_POINT('',#48545);
#13075=VERTEX_POINT('',#48547);
#13076=VERTEX_POINT('',#48549);
#13077=VERTEX_POINT('',#48553);
#13078=VERTEX_POINT('',#48557);
#13079=VERTEX_POINT('',#48563);
#13080=VERTEX_POINT('',#48564);
#13081=VERTEX_POINT('',#48566);
#13082=VERTEX_POINT('',#48568);
#13083=VERTEX_POINT('',#48572);
#13084=VERTEX_POINT('',#48576);
#13085=VERTEX_POINT('',#48582);
#13086=VERTEX_POINT('',#48583);
#13087=VERTEX_POINT('',#48585);
#13088=VERTEX_POINT('',#48587);
#13089=VERTEX_POINT('',#48591);
#13090=VERTEX_POINT('',#48595);
#13091=VERTEX_POINT('',#48601);
#13092=VERTEX_POINT('',#48602);
#13093=VERTEX_POINT('',#48604);
#13094=VERTEX_POINT('',#48606);
#13095=VERTEX_POINT('',#48610);
#13096=VERTEX_POINT('',#48614);
#13097=VERTEX_POINT('',#48620);
#13098=VERTEX_POINT('',#48621);
#13099=VERTEX_POINT('',#48623);
#13100=VERTEX_POINT('',#48625);
#13101=VERTEX_POINT('',#48629);
#13102=VERTEX_POINT('',#48633);
#13103=VERTEX_POINT('',#48639);
#13104=VERTEX_POINT('',#48640);
#13105=VERTEX_POINT('',#48642);
#13106=VERTEX_POINT('',#48644);
#13107=VERTEX_POINT('',#48648);
#13108=VERTEX_POINT('',#48652);
#13109=VERTEX_POINT('',#48658);
#13110=VERTEX_POINT('',#48659);
#13111=VERTEX_POINT('',#48661);
#13112=VERTEX_POINT('',#48663);
#13113=VERTEX_POINT('',#48667);
#13114=VERTEX_POINT('',#48671);
#13115=VERTEX_POINT('',#48677);
#13116=VERTEX_POINT('',#48678);
#13117=VERTEX_POINT('',#48680);
#13118=VERTEX_POINT('',#48682);
#13119=VERTEX_POINT('',#48686);
#13120=VERTEX_POINT('',#48690);
#13121=VERTEX_POINT('',#48696);
#13122=VERTEX_POINT('',#48697);
#13123=VERTEX_POINT('',#48699);
#13124=VERTEX_POINT('',#48701);
#13125=VERTEX_POINT('',#48705);
#13126=VERTEX_POINT('',#48709);
#13127=VERTEX_POINT('',#48715);
#13128=VERTEX_POINT('',#48716);
#13129=VERTEX_POINT('',#48718);
#13130=VERTEX_POINT('',#48720);
#13131=VERTEX_POINT('',#48724);
#13132=VERTEX_POINT('',#48728);
#13133=VERTEX_POINT('',#48734);
#13134=VERTEX_POINT('',#48735);
#13135=VERTEX_POINT('',#48737);
#13136=VERTEX_POINT('',#48739);
#13137=VERTEX_POINT('',#48743);
#13138=VERTEX_POINT('',#48747);
#13139=VERTEX_POINT('',#48753);
#13140=VERTEX_POINT('',#48754);
#13141=VERTEX_POINT('',#48756);
#13142=VERTEX_POINT('',#48758);
#13143=VERTEX_POINT('',#48762);
#13144=VERTEX_POINT('',#48766);
#13145=VERTEX_POINT('',#48772);
#13146=VERTEX_POINT('',#48773);
#13147=VERTEX_POINT('',#48775);
#13148=VERTEX_POINT('',#48777);
#13149=VERTEX_POINT('',#48781);
#13150=VERTEX_POINT('',#48785);
#13151=VERTEX_POINT('',#48791);
#13152=VERTEX_POINT('',#48792);
#13153=VERTEX_POINT('',#48796);
#13154=VERTEX_POINT('',#48797);
#13155=VERTEX_POINT('',#48799);
#13156=VERTEX_POINT('',#48801);
#13157=VERTEX_POINT('',#48805);
#13158=VERTEX_POINT('',#48807);
#13159=VERTEX_POINT('',#48811);
#13160=VERTEX_POINT('',#48813);
#13161=VERTEX_POINT('',#48817);
#13162=VERTEX_POINT('',#48819);
#13163=VERTEX_POINT('',#48823);
#13164=VERTEX_POINT('',#48825);
#13165=VERTEX_POINT('',#48833);
#13166=VERTEX_POINT('',#48834);
#13167=VERTEX_POINT('',#48836);
#13168=VERTEX_POINT('',#48841);
#13169=VERTEX_POINT('',#48845);
#13170=VERTEX_POINT('',#48848);
#13171=VERTEX_POINT('',#48855);
#13172=VERTEX_POINT('',#48859);
#13173=VERTEX_POINT('',#48864);
#13174=VERTEX_POINT('',#48869);
#16295=EDGE_CURVE('',#12883,#12884,#8176,.T.);
#16296=EDGE_CURVE('',#12883,#12885,#2326,.T.);
#16297=EDGE_CURVE('',#12885,#12886,#1430,.T.);
#16298=EDGE_CURVE('',#12886,#12884,#2327,.T.);
#16299=EDGE_CURVE('',#12887,#12888,#8177,.T.);
#16300=EDGE_CURVE('',#12887,#12883,#2328,.T.);
#16301=EDGE_CURVE('',#12884,#12888,#2329,.T.);
#16302=EDGE_CURVE('',#12889,#12890,#8178,.T.);
#16303=EDGE_CURVE('',#12889,#12887,#2330,.T.);
#16304=EDGE_CURVE('',#12888,#12890,#2331,.T.);
#16305=EDGE_CURVE('',#12891,#12892,#8179,.T.);
#16306=EDGE_CURVE('',#12891,#12889,#2332,.T.);
#16307=EDGE_CURVE('',#12890,#12892,#2333,.T.);
#16308=EDGE_CURVE('',#12893,#12894,#8180,.T.);
#16309=EDGE_CURVE('',#12893,#12891,#2334,.T.);
#16310=EDGE_CURVE('',#12892,#12894,#2335,.T.);
#16311=EDGE_CURVE('',#12895,#12896,#8181,.T.);
#16312=EDGE_CURVE('',#12895,#12893,#2336,.T.);
#16313=EDGE_CURVE('',#12894,#12896,#2337,.T.);
#16314=EDGE_CURVE('',#12897,#12898,#8182,.T.);
#16315=EDGE_CURVE('',#12897,#12895,#2338,.T.);
#16316=EDGE_CURVE('',#12896,#12898,#2339,.T.);
#16317=EDGE_CURVE('',#12899,#12900,#8183,.T.);
#16318=EDGE_CURVE('',#12899,#12897,#2340,.T.);
#16319=EDGE_CURVE('',#12898,#12900,#2341,.T.);
#16320=EDGE_CURVE('',#12901,#12902,#8184,.T.);
#16321=EDGE_CURVE('',#12901,#12899,#2342,.T.);
#16322=EDGE_CURVE('',#12900,#12902,#2343,.T.);
#16323=EDGE_CURVE('',#12903,#12904,#8185,.T.);
#16324=EDGE_CURVE('',#12903,#12901,#2344,.T.);
#16325=EDGE_CURVE('',#12902,#12904,#2345,.T.);
#16326=EDGE_CURVE('',#12905,#12906,#8186,.T.);
#16327=EDGE_CURVE('',#12905,#12907,#2346,.T.);
#16328=EDGE_CURVE('',#12908,#12907,#1431,.T.);
#16329=EDGE_CURVE('',#12906,#12908,#2347,.T.);
#16330=EDGE_CURVE('',#12909,#12910,#8187,.T.);
#16331=EDGE_CURVE('',#12909,#12905,#2348,.T.);
#16332=EDGE_CURVE('',#12910,#12906,#2349,.T.);
#16333=EDGE_CURVE('',#12911,#12912,#8188,.T.);
#16334=EDGE_CURVE('',#12911,#12909,#2350,.T.);
#16335=EDGE_CURVE('',#12912,#12910,#2351,.T.);
#16336=EDGE_CURVE('',#12913,#12914,#8189,.T.);
#16337=EDGE_CURVE('',#12913,#12911,#2352,.T.);
#16338=EDGE_CURVE('',#12914,#12912,#2353,.T.);
#16339=EDGE_CURVE('',#12915,#12916,#8190,.T.);
#16340=EDGE_CURVE('',#12915,#12913,#2354,.T.);
#16341=EDGE_CURVE('',#12916,#12914,#2355,.T.);
#16342=EDGE_CURVE('',#12917,#12918,#8191,.T.);
#16343=EDGE_CURVE('',#12917,#12915,#2356,.T.);
#16344=EDGE_CURVE('',#12918,#12916,#2357,.T.);
#16345=EDGE_CURVE('',#12919,#12920,#8192,.T.);
#16346=EDGE_CURVE('',#12919,#12917,#2358,.T.);
#16347=EDGE_CURVE('',#12920,#12918,#2359,.T.);
#16348=EDGE_CURVE('',#12921,#12922,#8193,.T.);
#16349=EDGE_CURVE('',#12921,#12919,#2360,.T.);
#16350=EDGE_CURVE('',#12922,#12920,#2361,.T.);
#16351=EDGE_CURVE('',#12923,#12924,#8194,.T.);
#16352=EDGE_CURVE('',#12923,#12921,#2362,.T.);
#16353=EDGE_CURVE('',#12924,#12922,#2363,.T.);
#16354=EDGE_CURVE('',#12925,#12926,#8195,.T.);
#16355=EDGE_CURVE('',#12925,#12923,#2364,.T.);
#16356=EDGE_CURVE('',#12926,#12924,#2365,.T.);
#16357=EDGE_CURVE('',#12907,#12927,#2366,.T.);
#16358=EDGE_CURVE('',#12928,#12927,#1432,.F.);
#16359=EDGE_CURVE('',#12929,#12928,#1433,.F.);
#16360=EDGE_CURVE('',#12929,#12908,#2367,.T.);
#16361=EDGE_CURVE('',#12904,#12929,#2368,.T.);
#16362=EDGE_CURVE('',#12930,#12886,#2369,.T.);
#16363=EDGE_CURVE('',#12930,#12926,#2370,.T.);
#16364=EDGE_CURVE('',#12886,#12931,#1434,.T.);
#16365=EDGE_CURVE('',#12931,#12885,#1435,.T.);
#16366=EDGE_CURVE('',#12885,#12932,#2371,.T.);
#16367=EDGE_CURVE('',#12932,#12930,#1436,.T.);
#16368=EDGE_CURVE('',#12932,#12925,#2372,.T.);
#16369=EDGE_CURVE('',#12927,#12903,#2373,.T.);
#16370=EDGE_CURVE('',#12933,#12934,#8196,.T.);
#16371=EDGE_CURVE('',#12933,#12935,#8197,.T.);
#16372=EDGE_CURVE('',#12936,#12935,#8198,.T.);
#16373=EDGE_CURVE('',#12934,#12936,#8199,.T.);
#16374=EDGE_CURVE('',#12934,#12937,#1437,.T.);
#16375=EDGE_CURVE('',#12936,#12937,#8200,.T.);
#16376=EDGE_CURVE('',#12937,#12938,#8201,.T.);
#16377=EDGE_CURVE('',#12935,#12938,#8202,.T.);
#16378=EDGE_CURVE('',#12938,#12933,#1438,.T.);
#16379=EDGE_CURVE('',#12939,#12940,#8203,.T.);
#16380=EDGE_CURVE('',#12939,#12941,#8204,.T.);
#16381=EDGE_CURVE('',#12942,#12941,#8205,.T.);
#16382=EDGE_CURVE('',#12940,#12942,#8206,.T.);
#16383=EDGE_CURVE('',#12940,#12943,#1439,.T.);
#16384=EDGE_CURVE('',#12942,#12943,#8207,.T.);
#16385=EDGE_CURVE('',#12943,#12944,#8208,.T.);
#16386=EDGE_CURVE('',#12941,#12944,#8209,.T.);
#16387=EDGE_CURVE('',#12944,#12939,#1440,.T.);
#16388=EDGE_CURVE('',#12945,#12946,#8210,.T.);
#16389=EDGE_CURVE('',#12945,#12947,#8211,.T.);
#16390=EDGE_CURVE('',#12948,#12947,#8212,.T.);
#16391=EDGE_CURVE('',#12946,#12948,#8213,.T.);
#16392=EDGE_CURVE('',#12946,#12949,#1441,.T.);
#16393=EDGE_CURVE('',#12948,#12949,#8214,.T.);
#16394=EDGE_CURVE('',#12949,#12950,#8215,.T.);
#16395=EDGE_CURVE('',#12947,#12950,#8216,.T.);
#16396=EDGE_CURVE('',#12950,#12945,#1442,.T.);
#16397=EDGE_CURVE('',#12951,#12952,#8217,.T.);
#16398=EDGE_CURVE('',#12951,#12953,#8218,.T.);
#16399=EDGE_CURVE('',#12954,#12953,#8219,.T.);
#16400=EDGE_CURVE('',#12952,#12954,#8220,.T.);
#16401=EDGE_CURVE('',#12952,#12955,#1443,.T.);
#16402=EDGE_CURVE('',#12954,#12955,#8221,.T.);
#16403=EDGE_CURVE('',#12955,#12956,#8222,.T.);
#16404=EDGE_CURVE('',#12953,#12956,#8223,.T.);
#16405=EDGE_CURVE('',#12956,#12951,#1444,.T.);
#16406=EDGE_CURVE('',#12957,#12958,#8224,.T.);
#16407=EDGE_CURVE('',#12957,#12959,#8225,.T.);
#16408=EDGE_CURVE('',#12960,#12959,#8226,.T.);
#16409=EDGE_CURVE('',#12958,#12960,#8227,.T.);
#16410=EDGE_CURVE('',#12958,#12961,#1445,.T.);
#16411=EDGE_CURVE('',#12960,#12961,#8228,.T.);
#16412=EDGE_CURVE('',#12961,#12962,#8229,.T.);
#16413=EDGE_CURVE('',#12959,#12962,#8230,.T.);
#16414=EDGE_CURVE('',#12962,#12957,#1446,.T.);
#16415=EDGE_CURVE('',#12963,#12964,#8231,.T.);
#16416=EDGE_CURVE('',#12963,#12965,#8232,.T.);
#16417=EDGE_CURVE('',#12966,#12965,#8233,.T.);
#16418=EDGE_CURVE('',#12964,#12966,#8234,.T.);
#16419=EDGE_CURVE('',#12964,#12967,#1447,.T.);
#16420=EDGE_CURVE('',#12966,#12967,#8235,.T.);
#16421=EDGE_CURVE('',#12967,#12968,#8236,.T.);
#16422=EDGE_CURVE('',#12965,#12968,#8237,.T.);
#16423=EDGE_CURVE('',#12968,#12963,#1448,.T.);
#16424=EDGE_CURVE('',#12969,#12970,#8238,.T.);
#16425=EDGE_CURVE('',#12969,#12971,#8239,.T.);
#16426=EDGE_CURVE('',#12972,#12971,#8240,.T.);
#16427=EDGE_CURVE('',#12970,#12972,#8241,.T.);
#16428=EDGE_CURVE('',#12970,#12973,#1449,.T.);
#16429=EDGE_CURVE('',#12972,#12973,#8242,.T.);
#16430=EDGE_CURVE('',#12973,#12974,#8243,.T.);
#16431=EDGE_CURVE('',#12971,#12974,#8244,.T.);
#16432=EDGE_CURVE('',#12974,#12969,#1450,.T.);
#16433=EDGE_CURVE('',#12975,#12976,#8245,.T.);
#16434=EDGE_CURVE('',#12975,#12977,#8246,.T.);
#16435=EDGE_CURVE('',#12978,#12977,#8247,.T.);
#16436=EDGE_CURVE('',#12976,#12978,#8248,.T.);
#16437=EDGE_CURVE('',#12976,#12979,#1451,.T.);
#16438=EDGE_CURVE('',#12978,#12979,#8249,.T.);
#16439=EDGE_CURVE('',#12979,#12980,#8250,.T.);
#16440=EDGE_CURVE('',#12977,#12980,#8251,.T.);
#16441=EDGE_CURVE('',#12980,#12975,#1452,.T.);
#16442=EDGE_CURVE('',#12981,#12982,#8252,.T.);
#16443=EDGE_CURVE('',#12981,#12983,#8253,.T.);
#16444=EDGE_CURVE('',#12984,#12983,#8254,.T.);
#16445=EDGE_CURVE('',#12982,#12984,#8255,.T.);
#16446=EDGE_CURVE('',#12982,#12985,#1453,.T.);
#16447=EDGE_CURVE('',#12984,#12985,#8256,.T.);
#16448=EDGE_CURVE('',#12985,#12986,#8257,.T.);
#16449=EDGE_CURVE('',#12983,#12986,#8258,.T.);
#16450=EDGE_CURVE('',#12986,#12981,#1454,.T.);
#16451=EDGE_CURVE('',#12987,#12988,#8259,.T.);
#16452=EDGE_CURVE('',#12987,#12989,#8260,.T.);
#16453=EDGE_CURVE('',#12990,#12989,#8261,.T.);
#16454=EDGE_CURVE('',#12988,#12990,#8262,.T.);
#16455=EDGE_CURVE('',#12988,#12991,#1455,.T.);
#16456=EDGE_CURVE('',#12990,#12991,#8263,.T.);
#16457=EDGE_CURVE('',#12991,#12992,#8264,.T.);
#16458=EDGE_CURVE('',#12989,#12992,#8265,.T.);
#16459=EDGE_CURVE('',#12992,#12987,#1456,.T.);
#16460=EDGE_CURVE('',#12993,#12994,#8266,.T.);
#16461=EDGE_CURVE('',#12993,#12995,#8267,.T.);
#16462=EDGE_CURVE('',#12996,#12995,#8268,.T.);
#16463=EDGE_CURVE('',#12994,#12996,#8269,.T.);
#16464=EDGE_CURVE('',#12994,#12997,#1457,.T.);
#16465=EDGE_CURVE('',#12996,#12997,#8270,.T.);
#16466=EDGE_CURVE('',#12997,#12998,#8271,.T.);
#16467=EDGE_CURVE('',#12995,#12998,#8272,.T.);
#16468=EDGE_CURVE('',#12998,#12993,#1458,.T.);
#16469=EDGE_CURVE('',#12999,#13000,#8273,.T.);
#16470=EDGE_CURVE('',#12999,#13001,#8274,.T.);
#16471=EDGE_CURVE('',#13002,#13001,#8275,.T.);
#16472=EDGE_CURVE('',#13000,#13002,#8276,.T.);
#16473=EDGE_CURVE('',#13000,#13003,#1459,.T.);
#16474=EDGE_CURVE('',#13002,#13003,#8277,.T.);
#16475=EDGE_CURVE('',#13003,#13004,#8278,.T.);
#16476=EDGE_CURVE('',#13001,#13004,#8279,.T.);
#16477=EDGE_CURVE('',#13004,#12999,#1460,.T.);
#16478=EDGE_CURVE('',#13005,#13006,#8280,.T.);
#16479=EDGE_CURVE('',#13005,#13007,#8281,.T.);
#16480=EDGE_CURVE('',#13008,#13007,#8282,.T.);
#16481=EDGE_CURVE('',#13006,#13008,#8283,.T.);
#16482=EDGE_CURVE('',#13006,#13009,#1461,.T.);
#16483=EDGE_CURVE('',#13008,#13009,#8284,.T.);
#16484=EDGE_CURVE('',#13009,#13010,#8285,.T.);
#16485=EDGE_CURVE('',#13007,#13010,#8286,.T.);
#16486=EDGE_CURVE('',#13010,#13005,#1462,.T.);
#16487=EDGE_CURVE('',#13011,#13012,#8287,.T.);
#16488=EDGE_CURVE('',#13011,#13013,#8288,.T.);
#16489=EDGE_CURVE('',#13014,#13013,#8289,.T.);
#16490=EDGE_CURVE('',#13012,#13014,#8290,.T.);
#16491=EDGE_CURVE('',#13012,#13015,#1463,.T.);
#16492=EDGE_CURVE('',#13014,#13015,#8291,.T.);
#16493=EDGE_CURVE('',#13015,#13016,#8292,.T.);
#16494=EDGE_CURVE('',#13013,#13016,#8293,.T.);
#16495=EDGE_CURVE('',#13016,#13011,#1464,.T.);
#16496=EDGE_CURVE('',#13017,#13018,#8294,.T.);
#16497=EDGE_CURVE('',#13017,#13019,#8295,.T.);
#16498=EDGE_CURVE('',#13020,#13019,#8296,.T.);
#16499=EDGE_CURVE('',#13018,#13020,#8297,.T.);
#16500=EDGE_CURVE('',#13018,#13021,#1465,.T.);
#16501=EDGE_CURVE('',#13020,#13021,#8298,.T.);
#16502=EDGE_CURVE('',#13021,#13022,#8299,.T.);
#16503=EDGE_CURVE('',#13019,#13022,#8300,.T.);
#16504=EDGE_CURVE('',#13022,#13017,#1466,.T.);
#16505=EDGE_CURVE('',#13023,#13024,#8301,.T.);
#16506=EDGE_CURVE('',#13023,#13025,#8302,.T.);
#16507=EDGE_CURVE('',#13026,#13025,#8303,.T.);
#16508=EDGE_CURVE('',#13024,#13026,#8304,.T.);
#16509=EDGE_CURVE('',#13024,#13027,#1467,.T.);
#16510=EDGE_CURVE('',#13026,#13027,#8305,.T.);
#16511=EDGE_CURVE('',#13027,#13028,#8306,.T.);
#16512=EDGE_CURVE('',#13025,#13028,#8307,.T.);
#16513=EDGE_CURVE('',#13028,#13023,#1468,.T.);
#16514=EDGE_CURVE('',#13029,#13030,#8308,.T.);
#16515=EDGE_CURVE('',#13029,#13031,#8309,.T.);
#16516=EDGE_CURVE('',#13032,#13031,#8310,.T.);
#16517=EDGE_CURVE('',#13030,#13032,#8311,.T.);
#16518=EDGE_CURVE('',#13030,#13033,#1469,.T.);
#16519=EDGE_CURVE('',#13032,#13033,#8312,.T.);
#16520=EDGE_CURVE('',#13033,#13034,#8313,.T.);
#16521=EDGE_CURVE('',#13031,#13034,#8314,.T.);
#16522=EDGE_CURVE('',#13034,#13029,#1470,.T.);
#16523=EDGE_CURVE('',#13035,#13036,#8315,.T.);
#16524=EDGE_CURVE('',#13035,#13037,#8316,.T.);
#16525=EDGE_CURVE('',#13038,#13037,#8317,.T.);
#16526=EDGE_CURVE('',#13036,#13038,#8318,.T.);
#16527=EDGE_CURVE('',#13036,#13039,#1471,.T.);
#16528=EDGE_CURVE('',#13038,#13040,#8319,.T.);
#16529=EDGE_CURVE('',#13039,#13040,#1472,.T.);
#16530=EDGE_CURVE('',#13040,#13041,#8320,.T.);
#16531=EDGE_CURVE('',#13037,#13041,#8321,.T.);
#16532=EDGE_CURVE('',#13041,#13042,#1473,.T.);
#16533=EDGE_CURVE('',#13042,#13035,#1474,.T.);
#16534=EDGE_CURVE('',#13043,#13044,#8322,.T.);
#16535=EDGE_CURVE('',#13043,#13045,#8323,.T.);
#16536=EDGE_CURVE('',#13046,#13045,#8324,.T.);
#16537=EDGE_CURVE('',#13044,#13046,#8325,.T.);
#16538=EDGE_CURVE('',#13044,#13047,#1475,.T.);
#16539=EDGE_CURVE('',#13046,#13047,#8326,.T.);
#16540=EDGE_CURVE('',#13047,#13048,#8327,.T.);
#16541=EDGE_CURVE('',#13045,#13048,#8328,.T.);
#16542=EDGE_CURVE('',#13048,#13043,#1476,.T.);
#16543=EDGE_CURVE('',#13049,#13050,#8329,.T.);
#16544=EDGE_CURVE('',#13049,#13051,#8330,.T.);
#16545=EDGE_CURVE('',#13052,#13051,#8331,.T.);
#16546=EDGE_CURVE('',#13050,#13052,#8332,.T.);
#16547=EDGE_CURVE('',#13050,#13053,#1477,.T.);
#16548=EDGE_CURVE('',#13052,#13053,#8333,.T.);
#16549=EDGE_CURVE('',#13053,#13054,#8334,.T.);
#16550=EDGE_CURVE('',#13051,#13054,#8335,.T.);
#16551=EDGE_CURVE('',#13054,#13049,#1478,.T.);
#16552=EDGE_CURVE('',#13055,#13056,#8336,.T.);
#16553=EDGE_CURVE('',#13055,#13057,#8337,.T.);
#16554=EDGE_CURVE('',#13058,#13057,#8338,.T.);
#16555=EDGE_CURVE('',#13056,#13058,#8339,.T.);
#16556=EDGE_CURVE('',#13056,#13059,#1479,.T.);
#16557=EDGE_CURVE('',#13058,#13059,#8340,.T.);
#16558=EDGE_CURVE('',#13059,#13060,#8341,.T.);
#16559=EDGE_CURVE('',#13057,#13060,#8342,.T.);
#16560=EDGE_CURVE('',#13060,#13055,#1480,.T.);
#16561=EDGE_CURVE('',#13061,#13062,#8343,.T.);
#16562=EDGE_CURVE('',#13061,#13063,#8344,.T.);
#16563=EDGE_CURVE('',#13064,#13063,#8345,.T.);
#16564=EDGE_CURVE('',#13062,#13064,#8346,.T.);
#16565=EDGE_CURVE('',#13062,#13065,#1481,.T.);
#16566=EDGE_CURVE('',#13064,#13065,#8347,.T.);
#16567=EDGE_CURVE('',#13065,#13066,#8348,.T.);
#16568=EDGE_CURVE('',#13063,#13066,#8349,.T.);
#16569=EDGE_CURVE('',#13066,#13061,#1482,.T.);
#16570=EDGE_CURVE('',#13067,#13068,#8350,.T.);
#16571=EDGE_CURVE('',#13067,#13069,#8351,.T.);
#16572=EDGE_CURVE('',#13070,#13069,#8352,.T.);
#16573=EDGE_CURVE('',#13068,#13070,#8353,.T.);
#16574=EDGE_CURVE('',#13068,#13071,#1483,.T.);
#16575=EDGE_CURVE('',#13070,#13071,#8354,.T.);
#16576=EDGE_CURVE('',#13071,#13072,#8355,.T.);
#16577=EDGE_CURVE('',#13069,#13072,#8356,.T.);
#16578=EDGE_CURVE('',#13072,#13067,#1484,.T.);
#16579=EDGE_CURVE('',#13073,#13074,#8357,.T.);
#16580=EDGE_CURVE('',#13073,#13075,#8358,.T.);
#16581=EDGE_CURVE('',#13076,#13075,#8359,.T.);
#16582=EDGE_CURVE('',#13074,#13076,#8360,.T.);
#16583=EDGE_CURVE('',#13074,#13077,#1485,.T.);
#16584=EDGE_CURVE('',#13076,#13077,#8361,.T.);
#16585=EDGE_CURVE('',#13077,#13078,#8362,.T.);
#16586=EDGE_CURVE('',#13075,#13078,#8363,.T.);
#16587=EDGE_CURVE('',#13078,#13073,#1486,.T.);
#16588=EDGE_CURVE('',#13079,#13080,#8364,.T.);
#16589=EDGE_CURVE('',#13079,#13081,#8365,.T.);
#16590=EDGE_CURVE('',#13082,#13081,#8366,.T.);
#16591=EDGE_CURVE('',#13080,#13082,#8367,.T.);
#16592=EDGE_CURVE('',#13080,#13083,#1487,.T.);
#16593=EDGE_CURVE('',#13082,#13083,#8368,.T.);
#16594=EDGE_CURVE('',#13083,#13084,#8369,.T.);
#16595=EDGE_CURVE('',#13081,#13084,#8370,.T.);
#16596=EDGE_CURVE('',#13084,#13079,#1488,.T.);
#16597=EDGE_CURVE('',#13085,#13086,#8371,.T.);
#16598=EDGE_CURVE('',#13085,#13087,#8372,.T.);
#16599=EDGE_CURVE('',#13088,#13087,#8373,.T.);
#16600=EDGE_CURVE('',#13086,#13088,#8374,.T.);
#16601=EDGE_CURVE('',#13086,#13089,#1489,.T.);
#16602=EDGE_CURVE('',#13088,#13089,#8375,.T.);
#16603=EDGE_CURVE('',#13089,#13090,#8376,.T.);
#16604=EDGE_CURVE('',#13087,#13090,#8377,.T.);
#16605=EDGE_CURVE('',#13090,#13085,#1490,.T.);
#16606=EDGE_CURVE('',#13091,#13092,#8378,.T.);
#16607=EDGE_CURVE('',#13091,#13093,#8379,.T.);
#16608=EDGE_CURVE('',#13094,#13093,#8380,.T.);
#16609=EDGE_CURVE('',#13092,#13094,#8381,.T.);
#16610=EDGE_CURVE('',#13092,#13095,#1491,.T.);
#16611=EDGE_CURVE('',#13094,#13095,#8382,.T.);
#16612=EDGE_CURVE('',#13095,#13096,#8383,.T.);
#16613=EDGE_CURVE('',#13093,#13096,#8384,.T.);
#16614=EDGE_CURVE('',#13096,#13091,#1492,.T.);
#16615=EDGE_CURVE('',#13097,#13098,#8385,.T.);
#16616=EDGE_CURVE('',#13097,#13099,#8386,.T.);
#16617=EDGE_CURVE('',#13100,#13099,#8387,.T.);
#16618=EDGE_CURVE('',#13098,#13100,#8388,.T.);
#16619=EDGE_CURVE('',#13098,#13101,#1493,.T.);
#16620=EDGE_CURVE('',#13100,#13101,#8389,.T.);
#16621=EDGE_CURVE('',#13101,#13102,#8390,.T.);
#16622=EDGE_CURVE('',#13099,#13102,#8391,.T.);
#16623=EDGE_CURVE('',#13102,#13097,#1494,.T.);
#16624=EDGE_CURVE('',#13103,#13104,#8392,.T.);
#16625=EDGE_CURVE('',#13103,#13105,#8393,.T.);
#16626=EDGE_CURVE('',#13106,#13105,#8394,.T.);
#16627=EDGE_CURVE('',#13104,#13106,#8395,.T.);
#16628=EDGE_CURVE('',#13104,#13107,#1495,.T.);
#16629=EDGE_CURVE('',#13106,#13107,#8396,.T.);
#16630=EDGE_CURVE('',#13107,#13108,#8397,.T.);
#16631=EDGE_CURVE('',#13105,#13108,#8398,.T.);
#16632=EDGE_CURVE('',#13108,#13103,#1496,.T.);
#16633=EDGE_CURVE('',#13109,#13110,#8399,.T.);
#16634=EDGE_CURVE('',#13109,#13111,#8400,.T.);
#16635=EDGE_CURVE('',#13112,#13111,#8401,.T.);
#16636=EDGE_CURVE('',#13110,#13112,#8402,.T.);
#16637=EDGE_CURVE('',#13110,#13113,#1497,.T.);
#16638=EDGE_CURVE('',#13112,#13113,#8403,.T.);
#16639=EDGE_CURVE('',#13113,#13114,#8404,.T.);
#16640=EDGE_CURVE('',#13111,#13114,#8405,.T.);
#16641=EDGE_CURVE('',#13114,#13109,#1498,.T.);
#16642=EDGE_CURVE('',#13115,#13116,#8406,.T.);
#16643=EDGE_CURVE('',#13115,#13117,#8407,.T.);
#16644=EDGE_CURVE('',#13118,#13117,#8408,.T.);
#16645=EDGE_CURVE('',#13116,#13118,#8409,.T.);
#16646=EDGE_CURVE('',#13116,#13119,#1499,.T.);
#16647=EDGE_CURVE('',#13118,#13119,#8410,.T.);
#16648=EDGE_CURVE('',#13119,#13120,#8411,.T.);
#16649=EDGE_CURVE('',#13117,#13120,#8412,.T.);
#16650=EDGE_CURVE('',#13120,#13115,#1500,.T.);
#16651=EDGE_CURVE('',#13121,#13122,#8413,.T.);
#16652=EDGE_CURVE('',#13121,#13123,#8414,.T.);
#16653=EDGE_CURVE('',#13124,#13123,#8415,.T.);
#16654=EDGE_CURVE('',#13122,#13124,#8416,.T.);
#16655=EDGE_CURVE('',#13122,#13125,#1501,.T.);
#16656=EDGE_CURVE('',#13124,#13125,#8417,.T.);
#16657=EDGE_CURVE('',#13125,#13126,#8418,.T.);
#16658=EDGE_CURVE('',#13123,#13126,#8419,.T.);
#16659=EDGE_CURVE('',#13126,#13121,#1502,.T.);
#16660=EDGE_CURVE('',#13127,#13128,#8420,.T.);
#16661=EDGE_CURVE('',#13127,#13129,#8421,.T.);
#16662=EDGE_CURVE('',#13130,#13129,#8422,.T.);
#16663=EDGE_CURVE('',#13128,#13130,#8423,.T.);
#16664=EDGE_CURVE('',#13128,#13131,#1503,.T.);
#16665=EDGE_CURVE('',#13130,#13131,#8424,.T.);
#16666=EDGE_CURVE('',#13131,#13132,#8425,.T.);
#16667=EDGE_CURVE('',#13129,#13132,#8426,.T.);
#16668=EDGE_CURVE('',#13132,#13127,#1504,.T.);
#16669=EDGE_CURVE('',#13133,#13134,#8427,.T.);
#16670=EDGE_CURVE('',#13133,#13135,#8428,.T.);
#16671=EDGE_CURVE('',#13136,#13135,#8429,.T.);
#16672=EDGE_CURVE('',#13134,#13136,#8430,.T.);
#16673=EDGE_CURVE('',#13134,#13137,#1505,.T.);
#16674=EDGE_CURVE('',#13136,#13137,#8431,.T.);
#16675=EDGE_CURVE('',#13137,#13138,#8432,.T.);
#16676=EDGE_CURVE('',#13135,#13138,#8433,.T.);
#16677=EDGE_CURVE('',#13138,#13133,#1506,.T.);
#16678=EDGE_CURVE('',#13139,#13140,#8434,.T.);
#16679=EDGE_CURVE('',#13139,#13141,#8435,.T.);
#16680=EDGE_CURVE('',#13142,#13141,#8436,.T.);
#16681=EDGE_CURVE('',#13140,#13142,#8437,.T.);
#16682=EDGE_CURVE('',#13140,#13143,#1507,.T.);
#16683=EDGE_CURVE('',#13142,#13143,#8438,.T.);
#16684=EDGE_CURVE('',#13143,#13144,#8439,.T.);
#16685=EDGE_CURVE('',#13141,#13144,#8440,.T.);
#16686=EDGE_CURVE('',#13144,#13139,#1508,.T.);
#16687=EDGE_CURVE('',#13145,#13146,#8441,.T.);
#16688=EDGE_CURVE('',#13145,#13147,#8442,.T.);
#16689=EDGE_CURVE('',#13148,#13147,#8443,.T.);
#16690=EDGE_CURVE('',#13146,#13148,#8444,.T.);
#16691=EDGE_CURVE('',#13146,#13149,#1509,.T.);
#16692=EDGE_CURVE('',#13148,#13149,#8445,.T.);
#16693=EDGE_CURVE('',#13149,#13150,#8446,.T.);
#16694=EDGE_CURVE('',#13147,#13150,#8447,.T.);
#16695=EDGE_CURVE('',#13150,#13145,#1510,.T.);
#16696=EDGE_CURVE('',#13151,#13152,#8448,.T.);
#16697=EDGE_CURVE('',#13152,#13152,#1511,.T.);
#16698=EDGE_CURVE('',#13153,#13154,#8449,.T.);
#16699=EDGE_CURVE('',#13153,#13155,#8450,.T.);
#16700=EDGE_CURVE('',#13155,#13156,#8451,.T.);
#16701=EDGE_CURVE('',#13154,#13156,#8452,.T.);
#16702=EDGE_CURVE('',#13157,#13153,#8453,.T.);
#16703=EDGE_CURVE('',#13157,#13158,#8454,.T.);
#16704=EDGE_CURVE('',#13158,#13155,#8455,.T.);
#16705=EDGE_CURVE('',#13159,#13157,#8456,.T.);
#16706=EDGE_CURVE('',#13159,#13160,#8457,.T.);
#16707=EDGE_CURVE('',#13160,#13158,#8458,.T.);
#16708=EDGE_CURVE('',#13161,#13159,#8459,.T.);
#16709=EDGE_CURVE('',#13161,#13162,#8460,.T.);
#16710=EDGE_CURVE('',#13162,#13160,#8461,.T.);
#16711=EDGE_CURVE('',#13163,#13161,#8462,.T.);
#16712=EDGE_CURVE('',#13163,#13164,#8463,.T.);
#16713=EDGE_CURVE('',#13164,#13162,#8464,.T.);
#16714=EDGE_CURVE('',#13154,#13163,#8465,.T.);
#16715=EDGE_CURVE('',#13156,#13164,#8466,.T.);
#16716=EDGE_CURVE('',#13165,#13166,#1512,.T.);
#16717=EDGE_CURVE('',#13166,#13167,#1513,.T.);
#16718=EDGE_CURVE('',#13167,#13167,#1514,.T.);
#16719=EDGE_CURVE('',#13166,#13165,#1515,.T.);
#16720=EDGE_CURVE('',#13165,#13168,#8467,.T.);
#16721=EDGE_CURVE('',#13168,#13168,#1516,.T.);
#16722=EDGE_CURVE('',#13169,#13169,#1517,.T.);
#16723=EDGE_CURVE('',#13170,#13170,#1518,.T.);
#16724=EDGE_CURVE('',#12931,#13170,#8468,.T.);
#16725=EDGE_CURVE('',#12927,#12929,#1519,.F.);
#16726=EDGE_CURVE('',#13171,#13171,#1520,.T.);
#16727=EDGE_CURVE('',#13171,#12928,#8469,.T.);
#16728=EDGE_CURVE('',#13172,#13172,#1521,.T.);
#16729=EDGE_CURVE('',#13172,#13171,#8470,.T.);
#16730=EDGE_CURVE('',#13173,#13173,#1522,.T.);
#16731=EDGE_CURVE('',#13173,#13042,#8471,.T.);
#16732=EDGE_CURVE('',#13039,#13169,#8472,.T.);
#16733=EDGE_CURVE('',#13174,#13174,#1523,.T.);
#16734=EDGE_CURVE('',#13174,#13173,#8473,.T.);
#22147=ORIENTED_EDGE('',*,*,#16295,.F.);
#22148=ORIENTED_EDGE('',*,*,#16296,.T.);
#22149=ORIENTED_EDGE('',*,*,#16297,.T.);
#22150=ORIENTED_EDGE('',*,*,#16298,.T.);
#22151=ORIENTED_EDGE('',*,*,#16299,.F.);
#22152=ORIENTED_EDGE('',*,*,#16300,.T.);
#22153=ORIENTED_EDGE('',*,*,#16295,.T.);
#22154=ORIENTED_EDGE('',*,*,#16301,.T.);
#22155=ORIENTED_EDGE('',*,*,#16302,.F.);
#22156=ORIENTED_EDGE('',*,*,#16303,.T.);
#22157=ORIENTED_EDGE('',*,*,#16299,.T.);
#22158=ORIENTED_EDGE('',*,*,#16304,.T.);
#22159=ORIENTED_EDGE('',*,*,#16305,.F.);
#22160=ORIENTED_EDGE('',*,*,#16306,.T.);
#22161=ORIENTED_EDGE('',*,*,#16302,.T.);
#22162=ORIENTED_EDGE('',*,*,#16307,.T.);
#22163=ORIENTED_EDGE('',*,*,#16308,.F.);
#22164=ORIENTED_EDGE('',*,*,#16309,.T.);
#22165=ORIENTED_EDGE('',*,*,#16305,.T.);
#22166=ORIENTED_EDGE('',*,*,#16310,.T.);
#22167=ORIENTED_EDGE('',*,*,#16311,.F.);
#22168=ORIENTED_EDGE('',*,*,#16312,.T.);
#22169=ORIENTED_EDGE('',*,*,#16308,.T.);
#22170=ORIENTED_EDGE('',*,*,#16313,.T.);
#22171=ORIENTED_EDGE('',*,*,#16314,.F.);
#22172=ORIENTED_EDGE('',*,*,#16315,.T.);
#22173=ORIENTED_EDGE('',*,*,#16311,.T.);
#22174=ORIENTED_EDGE('',*,*,#16316,.T.);
#22175=ORIENTED_EDGE('',*,*,#16317,.F.);
#22176=ORIENTED_EDGE('',*,*,#16318,.T.);
#22177=ORIENTED_EDGE('',*,*,#16314,.T.);
#22178=ORIENTED_EDGE('',*,*,#16319,.T.);
#22179=ORIENTED_EDGE('',*,*,#16320,.F.);
#22180=ORIENTED_EDGE('',*,*,#16321,.T.);
#22181=ORIENTED_EDGE('',*,*,#16317,.T.);
#22182=ORIENTED_EDGE('',*,*,#16322,.T.);
#22183=ORIENTED_EDGE('',*,*,#16323,.F.);
#22184=ORIENTED_EDGE('',*,*,#16324,.T.);
#22185=ORIENTED_EDGE('',*,*,#16320,.T.);
#22186=ORIENTED_EDGE('',*,*,#16325,.T.);
#22187=ORIENTED_EDGE('',*,*,#16326,.F.);
#22188=ORIENTED_EDGE('',*,*,#16327,.T.);
#22189=ORIENTED_EDGE('',*,*,#16328,.F.);
#22190=ORIENTED_EDGE('',*,*,#16329,.F.);
#22191=ORIENTED_EDGE('',*,*,#16330,.F.);
#22192=ORIENTED_EDGE('',*,*,#16331,.T.);
#22193=ORIENTED_EDGE('',*,*,#16326,.T.);
#22194=ORIENTED_EDGE('',*,*,#16332,.F.);
#22195=ORIENTED_EDGE('',*,*,#16333,.F.);
#22196=ORIENTED_EDGE('',*,*,#16334,.T.);
#22197=ORIENTED_EDGE('',*,*,#16330,.T.);
#22198=ORIENTED_EDGE('',*,*,#16335,.F.);
#22199=ORIENTED_EDGE('',*,*,#16336,.F.);
#22200=ORIENTED_EDGE('',*,*,#16337,.T.);
#22201=ORIENTED_EDGE('',*,*,#16333,.T.);
#22202=ORIENTED_EDGE('',*,*,#16338,.F.);
#22203=ORIENTED_EDGE('',*,*,#16339,.F.);
#22204=ORIENTED_EDGE('',*,*,#16340,.T.);
#22205=ORIENTED_EDGE('',*,*,#16336,.T.);
#22206=ORIENTED_EDGE('',*,*,#16341,.F.);
#22207=ORIENTED_EDGE('',*,*,#16342,.F.);
#22208=ORIENTED_EDGE('',*,*,#16343,.T.);
#22209=ORIENTED_EDGE('',*,*,#16339,.T.);
#22210=ORIENTED_EDGE('',*,*,#16344,.F.);
#22211=ORIENTED_EDGE('',*,*,#16345,.F.);
#22212=ORIENTED_EDGE('',*,*,#16346,.T.);
#22213=ORIENTED_EDGE('',*,*,#16342,.T.);
#22214=ORIENTED_EDGE('',*,*,#16347,.F.);
#22215=ORIENTED_EDGE('',*,*,#16348,.F.);
#22216=ORIENTED_EDGE('',*,*,#16349,.T.);
#22217=ORIENTED_EDGE('',*,*,#16345,.T.);
#22218=ORIENTED_EDGE('',*,*,#16350,.F.);
#22219=ORIENTED_EDGE('',*,*,#16351,.F.);
#22220=ORIENTED_EDGE('',*,*,#16352,.T.);
#22221=ORIENTED_EDGE('',*,*,#16348,.T.);
#22222=ORIENTED_EDGE('',*,*,#16353,.F.);
#22223=ORIENTED_EDGE('',*,*,#16354,.F.);
#22224=ORIENTED_EDGE('',*,*,#16355,.T.);
#22225=ORIENTED_EDGE('',*,*,#16351,.T.);
#22226=ORIENTED_EDGE('',*,*,#16356,.F.);
#22227=ORIENTED_EDGE('',*,*,#16328,.T.);
#22228=ORIENTED_EDGE('',*,*,#16357,.T.);
#22229=ORIENTED_EDGE('',*,*,#16358,.F.);
#22230=ORIENTED_EDGE('',*,*,#16359,.F.);
#22231=ORIENTED_EDGE('',*,*,#16360,.T.);
#22232=ORIENTED_EDGE('',*,*,#16360,.F.);
#22233=ORIENTED_EDGE('',*,*,#16361,.F.);
#22234=ORIENTED_EDGE('',*,*,#16325,.F.);
#22235=ORIENTED_EDGE('',*,*,#16322,.F.);
#22236=ORIENTED_EDGE('',*,*,#16319,.F.);
#22237=ORIENTED_EDGE('',*,*,#16316,.F.);
#22238=ORIENTED_EDGE('',*,*,#16313,.F.);
#22239=ORIENTED_EDGE('',*,*,#16310,.F.);
#22240=ORIENTED_EDGE('',*,*,#16307,.F.);
#22241=ORIENTED_EDGE('',*,*,#16304,.F.);
#22242=ORIENTED_EDGE('',*,*,#16301,.F.);
#22243=ORIENTED_EDGE('',*,*,#16298,.F.);
#22244=ORIENTED_EDGE('',*,*,#16362,.F.);
#22245=ORIENTED_EDGE('',*,*,#16363,.T.);
#22246=ORIENTED_EDGE('',*,*,#16356,.T.);
#22247=ORIENTED_EDGE('',*,*,#16353,.T.);
#22248=ORIENTED_EDGE('',*,*,#16350,.T.);
#22249=ORIENTED_EDGE('',*,*,#16347,.T.);
#22250=ORIENTED_EDGE('',*,*,#16344,.T.);
#22251=ORIENTED_EDGE('',*,*,#16341,.T.);
#22252=ORIENTED_EDGE('',*,*,#16338,.T.);
#22253=ORIENTED_EDGE('',*,*,#16335,.T.);
#22254=ORIENTED_EDGE('',*,*,#16332,.T.);
#22255=ORIENTED_EDGE('',*,*,#16329,.T.);
#22256=ORIENTED_EDGE('',*,*,#16364,.T.);
#22257=ORIENTED_EDGE('',*,*,#16365,.T.);
#22258=ORIENTED_EDGE('',*,*,#16366,.T.);
#22259=ORIENTED_EDGE('',*,*,#16367,.T.);
#22260=ORIENTED_EDGE('',*,*,#16362,.T.);
#22261=ORIENTED_EDGE('',*,*,#16354,.T.);
#22262=ORIENTED_EDGE('',*,*,#16363,.F.);
#22263=ORIENTED_EDGE('',*,*,#16367,.F.);
#22264=ORIENTED_EDGE('',*,*,#16368,.T.);
#22265=ORIENTED_EDGE('',*,*,#16357,.F.);
#22266=ORIENTED_EDGE('',*,*,#16327,.F.);
#22267=ORIENTED_EDGE('',*,*,#16331,.F.);
#22268=ORIENTED_EDGE('',*,*,#16334,.F.);
#22269=ORIENTED_EDGE('',*,*,#16337,.F.);
#22270=ORIENTED_EDGE('',*,*,#16340,.F.);
#22271=ORIENTED_EDGE('',*,*,#16343,.F.);
#22272=ORIENTED_EDGE('',*,*,#16346,.F.);
#22273=ORIENTED_EDGE('',*,*,#16349,.F.);
#22274=ORIENTED_EDGE('',*,*,#16352,.F.);
#22275=ORIENTED_EDGE('',*,*,#16355,.F.);
#22276=ORIENTED_EDGE('',*,*,#16368,.F.);
#22277=ORIENTED_EDGE('',*,*,#16366,.F.);
#22278=ORIENTED_EDGE('',*,*,#16296,.F.);
#22279=ORIENTED_EDGE('',*,*,#16300,.F.);
#22280=ORIENTED_EDGE('',*,*,#16303,.F.);
#22281=ORIENTED_EDGE('',*,*,#16306,.F.);
#22282=ORIENTED_EDGE('',*,*,#16309,.F.);
#22283=ORIENTED_EDGE('',*,*,#16312,.F.);
#22284=ORIENTED_EDGE('',*,*,#16315,.F.);
#22285=ORIENTED_EDGE('',*,*,#16318,.F.);
#22286=ORIENTED_EDGE('',*,*,#16321,.F.);
#22287=ORIENTED_EDGE('',*,*,#16324,.F.);
#22288=ORIENTED_EDGE('',*,*,#16369,.F.);
#22289=ORIENTED_EDGE('',*,*,#16370,.F.);
#22290=ORIENTED_EDGE('',*,*,#16371,.T.);
#22291=ORIENTED_EDGE('',*,*,#16372,.F.);
#22292=ORIENTED_EDGE('',*,*,#16373,.F.);
#22293=ORIENTED_EDGE('',*,*,#16374,.F.);
#22294=ORIENTED_EDGE('',*,*,#16373,.T.);
#22295=ORIENTED_EDGE('',*,*,#16375,.T.);
#22296=ORIENTED_EDGE('',*,*,#16376,.F.);
#22297=ORIENTED_EDGE('',*,*,#16375,.F.);
#22298=ORIENTED_EDGE('',*,*,#16372,.T.);
#22299=ORIENTED_EDGE('',*,*,#16377,.T.);
#22300=ORIENTED_EDGE('',*,*,#16378,.F.);
#22301=ORIENTED_EDGE('',*,*,#16377,.F.);
#22302=ORIENTED_EDGE('',*,*,#16371,.F.);
#22303=ORIENTED_EDGE('',*,*,#16379,.F.);
#22304=ORIENTED_EDGE('',*,*,#16380,.T.);
#22305=ORIENTED_EDGE('',*,*,#16381,.F.);
#22306=ORIENTED_EDGE('',*,*,#16382,.F.);
#22307=ORIENTED_EDGE('',*,*,#16383,.F.);
#22308=ORIENTED_EDGE('',*,*,#16382,.T.);
#22309=ORIENTED_EDGE('',*,*,#16384,.T.);
#22310=ORIENTED_EDGE('',*,*,#16385,.F.);
#22311=ORIENTED_EDGE('',*,*,#16384,.F.);
#22312=ORIENTED_EDGE('',*,*,#16381,.T.);
#22313=ORIENTED_EDGE('',*,*,#16386,.T.);
#22314=ORIENTED_EDGE('',*,*,#16387,.F.);
#22315=ORIENTED_EDGE('',*,*,#16386,.F.);
#22316=ORIENTED_EDGE('',*,*,#16380,.F.);
#22317=ORIENTED_EDGE('',*,*,#16388,.F.);
#22318=ORIENTED_EDGE('',*,*,#16389,.T.);
#22319=ORIENTED_EDGE('',*,*,#16390,.F.);
#22320=ORIENTED_EDGE('',*,*,#16391,.F.);
#22321=ORIENTED_EDGE('',*,*,#16392,.F.);
#22322=ORIENTED_EDGE('',*,*,#16391,.T.);
#22323=ORIENTED_EDGE('',*,*,#16393,.T.);
#22324=ORIENTED_EDGE('',*,*,#16394,.F.);
#22325=ORIENTED_EDGE('',*,*,#16393,.F.);
#22326=ORIENTED_EDGE('',*,*,#16390,.T.);
#22327=ORIENTED_EDGE('',*,*,#16395,.T.);
#22328=ORIENTED_EDGE('',*,*,#16396,.F.);
#22329=ORIENTED_EDGE('',*,*,#16395,.F.);
#22330=ORIENTED_EDGE('',*,*,#16389,.F.);
#22331=ORIENTED_EDGE('',*,*,#16397,.F.);
#22332=ORIENTED_EDGE('',*,*,#16398,.T.);
#22333=ORIENTED_EDGE('',*,*,#16399,.F.);
#22334=ORIENTED_EDGE('',*,*,#16400,.F.);
#22335=ORIENTED_EDGE('',*,*,#16401,.F.);
#22336=ORIENTED_EDGE('',*,*,#16400,.T.);
#22337=ORIENTED_EDGE('',*,*,#16402,.T.);
#22338=ORIENTED_EDGE('',*,*,#16403,.F.);
#22339=ORIENTED_EDGE('',*,*,#16402,.F.);
#22340=ORIENTED_EDGE('',*,*,#16399,.T.);
#22341=ORIENTED_EDGE('',*,*,#16404,.T.);
#22342=ORIENTED_EDGE('',*,*,#16405,.F.);
#22343=ORIENTED_EDGE('',*,*,#16404,.F.);
#22344=ORIENTED_EDGE('',*,*,#16398,.F.);
#22345=ORIENTED_EDGE('',*,*,#16406,.F.);
#22346=ORIENTED_EDGE('',*,*,#16407,.T.);
#22347=ORIENTED_EDGE('',*,*,#16408,.F.);
#22348=ORIENTED_EDGE('',*,*,#16409,.F.);
#22349=ORIENTED_EDGE('',*,*,#16410,.F.);
#22350=ORIENTED_EDGE('',*,*,#16409,.T.);
#22351=ORIENTED_EDGE('',*,*,#16411,.T.);
#22352=ORIENTED_EDGE('',*,*,#16412,.F.);
#22353=ORIENTED_EDGE('',*,*,#16411,.F.);
#22354=ORIENTED_EDGE('',*,*,#16408,.T.);
#22355=ORIENTED_EDGE('',*,*,#16413,.T.);
#22356=ORIENTED_EDGE('',*,*,#16414,.F.);
#22357=ORIENTED_EDGE('',*,*,#16413,.F.);
#22358=ORIENTED_EDGE('',*,*,#16407,.F.);
#22359=ORIENTED_EDGE('',*,*,#16415,.F.);
#22360=ORIENTED_EDGE('',*,*,#16416,.T.);
#22361=ORIENTED_EDGE('',*,*,#16417,.F.);
#22362=ORIENTED_EDGE('',*,*,#16418,.F.);
#22363=ORIENTED_EDGE('',*,*,#16419,.F.);
#22364=ORIENTED_EDGE('',*,*,#16418,.T.);
#22365=ORIENTED_EDGE('',*,*,#16420,.T.);
#22366=ORIENTED_EDGE('',*,*,#16421,.F.);
#22367=ORIENTED_EDGE('',*,*,#16420,.F.);
#22368=ORIENTED_EDGE('',*,*,#16417,.T.);
#22369=ORIENTED_EDGE('',*,*,#16422,.T.);
#22370=ORIENTED_EDGE('',*,*,#16423,.F.);
#22371=ORIENTED_EDGE('',*,*,#16422,.F.);
#22372=ORIENTED_EDGE('',*,*,#16416,.F.);
#22373=ORIENTED_EDGE('',*,*,#16424,.F.);
#22374=ORIENTED_EDGE('',*,*,#16425,.T.);
#22375=ORIENTED_EDGE('',*,*,#16426,.F.);
#22376=ORIENTED_EDGE('',*,*,#16427,.F.);
#22377=ORIENTED_EDGE('',*,*,#16428,.F.);
#22378=ORIENTED_EDGE('',*,*,#16427,.T.);
#22379=ORIENTED_EDGE('',*,*,#16429,.T.);
#22380=ORIENTED_EDGE('',*,*,#16430,.F.);
#22381=ORIENTED_EDGE('',*,*,#16429,.F.);
#22382=ORIENTED_EDGE('',*,*,#16426,.T.);
#22383=ORIENTED_EDGE('',*,*,#16431,.T.);
#22384=ORIENTED_EDGE('',*,*,#16432,.F.);
#22385=ORIENTED_EDGE('',*,*,#16431,.F.);
#22386=ORIENTED_EDGE('',*,*,#16425,.F.);
#22387=ORIENTED_EDGE('',*,*,#16433,.F.);
#22388=ORIENTED_EDGE('',*,*,#16434,.T.);
#22389=ORIENTED_EDGE('',*,*,#16435,.F.);
#22390=ORIENTED_EDGE('',*,*,#16436,.F.);
#22391=ORIENTED_EDGE('',*,*,#16437,.F.);
#22392=ORIENTED_EDGE('',*,*,#16436,.T.);
#22393=ORIENTED_EDGE('',*,*,#16438,.T.);
#22394=ORIENTED_EDGE('',*,*,#16439,.F.);
#22395=ORIENTED_EDGE('',*,*,#16438,.F.);
#22396=ORIENTED_EDGE('',*,*,#16435,.T.);
#22397=ORIENTED_EDGE('',*,*,#16440,.T.);
#22398=ORIENTED_EDGE('',*,*,#16441,.F.);
#22399=ORIENTED_EDGE('',*,*,#16440,.F.);
#22400=ORIENTED_EDGE('',*,*,#16434,.F.);
#22401=ORIENTED_EDGE('',*,*,#16442,.F.);
#22402=ORIENTED_EDGE('',*,*,#16443,.T.);
#22403=ORIENTED_EDGE('',*,*,#16444,.F.);
#22404=ORIENTED_EDGE('',*,*,#16445,.F.);
#22405=ORIENTED_EDGE('',*,*,#16446,.F.);
#22406=ORIENTED_EDGE('',*,*,#16445,.T.);
#22407=ORIENTED_EDGE('',*,*,#16447,.T.);
#22408=ORIENTED_EDGE('',*,*,#16448,.F.);
#22409=ORIENTED_EDGE('',*,*,#16447,.F.);
#22410=ORIENTED_EDGE('',*,*,#16444,.T.);
#22411=ORIENTED_EDGE('',*,*,#16449,.T.);
#22412=ORIENTED_EDGE('',*,*,#16450,.F.);
#22413=ORIENTED_EDGE('',*,*,#16449,.F.);
#22414=ORIENTED_EDGE('',*,*,#16443,.F.);
#22415=ORIENTED_EDGE('',*,*,#16451,.F.);
#22416=ORIENTED_EDGE('',*,*,#16452,.T.);
#22417=ORIENTED_EDGE('',*,*,#16453,.F.);
#22418=ORIENTED_EDGE('',*,*,#16454,.F.);
#22419=ORIENTED_EDGE('',*,*,#16455,.F.);
#22420=ORIENTED_EDGE('',*,*,#16454,.T.);
#22421=ORIENTED_EDGE('',*,*,#16456,.T.);
#22422=ORIENTED_EDGE('',*,*,#16457,.F.);
#22423=ORIENTED_EDGE('',*,*,#16456,.F.);
#22424=ORIENTED_EDGE('',*,*,#16453,.T.);
#22425=ORIENTED_EDGE('',*,*,#16458,.T.);
#22426=ORIENTED_EDGE('',*,*,#16459,.F.);
#22427=ORIENTED_EDGE('',*,*,#16458,.F.);
#22428=ORIENTED_EDGE('',*,*,#16452,.F.);
#22429=ORIENTED_EDGE('',*,*,#16460,.F.);
#22430=ORIENTED_EDGE('',*,*,#16461,.T.);
#22431=ORIENTED_EDGE('',*,*,#16462,.F.);
#22432=ORIENTED_EDGE('',*,*,#16463,.F.);
#22433=ORIENTED_EDGE('',*,*,#16464,.F.);
#22434=ORIENTED_EDGE('',*,*,#16463,.T.);
#22435=ORIENTED_EDGE('',*,*,#16465,.T.);
#22436=ORIENTED_EDGE('',*,*,#16466,.F.);
#22437=ORIENTED_EDGE('',*,*,#16465,.F.);
#22438=ORIENTED_EDGE('',*,*,#16462,.T.);
#22439=ORIENTED_EDGE('',*,*,#16467,.T.);
#22440=ORIENTED_EDGE('',*,*,#16468,.F.);
#22441=ORIENTED_EDGE('',*,*,#16467,.F.);
#22442=ORIENTED_EDGE('',*,*,#16461,.F.);
#22443=ORIENTED_EDGE('',*,*,#16469,.F.);
#22444=ORIENTED_EDGE('',*,*,#16470,.T.);
#22445=ORIENTED_EDGE('',*,*,#16471,.F.);
#22446=ORIENTED_EDGE('',*,*,#16472,.F.);
#22447=ORIENTED_EDGE('',*,*,#16473,.F.);
#22448=ORIENTED_EDGE('',*,*,#16472,.T.);
#22449=ORIENTED_EDGE('',*,*,#16474,.T.);
#22450=ORIENTED_EDGE('',*,*,#16475,.F.);
#22451=ORIENTED_EDGE('',*,*,#16474,.F.);
#22452=ORIENTED_EDGE('',*,*,#16471,.T.);
#22453=ORIENTED_EDGE('',*,*,#16476,.T.);
#22454=ORIENTED_EDGE('',*,*,#16477,.F.);
#22455=ORIENTED_EDGE('',*,*,#16476,.F.);
#22456=ORIENTED_EDGE('',*,*,#16470,.F.);
#22457=ORIENTED_EDGE('',*,*,#16478,.F.);
#22458=ORIENTED_EDGE('',*,*,#16479,.T.);
#22459=ORIENTED_EDGE('',*,*,#16480,.F.);
#22460=ORIENTED_EDGE('',*,*,#16481,.F.);
#22461=ORIENTED_EDGE('',*,*,#16482,.F.);
#22462=ORIENTED_EDGE('',*,*,#16481,.T.);
#22463=ORIENTED_EDGE('',*,*,#16483,.T.);
#22464=ORIENTED_EDGE('',*,*,#16484,.F.);
#22465=ORIENTED_EDGE('',*,*,#16483,.F.);
#22466=ORIENTED_EDGE('',*,*,#16480,.T.);
#22467=ORIENTED_EDGE('',*,*,#16485,.T.);
#22468=ORIENTED_EDGE('',*,*,#16486,.F.);
#22469=ORIENTED_EDGE('',*,*,#16485,.F.);
#22470=ORIENTED_EDGE('',*,*,#16479,.F.);
#22471=ORIENTED_EDGE('',*,*,#16487,.F.);
#22472=ORIENTED_EDGE('',*,*,#16488,.T.);
#22473=ORIENTED_EDGE('',*,*,#16489,.F.);
#22474=ORIENTED_EDGE('',*,*,#16490,.F.);
#22475=ORIENTED_EDGE('',*,*,#16491,.F.);
#22476=ORIENTED_EDGE('',*,*,#16490,.T.);
#22477=ORIENTED_EDGE('',*,*,#16492,.T.);
#22478=ORIENTED_EDGE('',*,*,#16493,.F.);
#22479=ORIENTED_EDGE('',*,*,#16492,.F.);
#22480=ORIENTED_EDGE('',*,*,#16489,.T.);
#22481=ORIENTED_EDGE('',*,*,#16494,.T.);
#22482=ORIENTED_EDGE('',*,*,#16495,.F.);
#22483=ORIENTED_EDGE('',*,*,#16494,.F.);
#22484=ORIENTED_EDGE('',*,*,#16488,.F.);
#22485=ORIENTED_EDGE('',*,*,#16496,.F.);
#22486=ORIENTED_EDGE('',*,*,#16497,.T.);
#22487=ORIENTED_EDGE('',*,*,#16498,.F.);
#22488=ORIENTED_EDGE('',*,*,#16499,.F.);
#22489=ORIENTED_EDGE('',*,*,#16500,.F.);
#22490=ORIENTED_EDGE('',*,*,#16499,.T.);
#22491=ORIENTED_EDGE('',*,*,#16501,.T.);
#22492=ORIENTED_EDGE('',*,*,#16502,.F.);
#22493=ORIENTED_EDGE('',*,*,#16501,.F.);
#22494=ORIENTED_EDGE('',*,*,#16498,.T.);
#22495=ORIENTED_EDGE('',*,*,#16503,.T.);
#22496=ORIENTED_EDGE('',*,*,#16504,.F.);
#22497=ORIENTED_EDGE('',*,*,#16503,.F.);
#22498=ORIENTED_EDGE('',*,*,#16497,.F.);
#22499=ORIENTED_EDGE('',*,*,#16505,.F.);
#22500=ORIENTED_EDGE('',*,*,#16506,.T.);
#22501=ORIENTED_EDGE('',*,*,#16507,.F.);
#22502=ORIENTED_EDGE('',*,*,#16508,.F.);
#22503=ORIENTED_EDGE('',*,*,#16509,.F.);
#22504=ORIENTED_EDGE('',*,*,#16508,.T.);
#22505=ORIENTED_EDGE('',*,*,#16510,.T.);
#22506=ORIENTED_EDGE('',*,*,#16511,.F.);
#22507=ORIENTED_EDGE('',*,*,#16510,.F.);
#22508=ORIENTED_EDGE('',*,*,#16507,.T.);
#22509=ORIENTED_EDGE('',*,*,#16512,.T.);
#22510=ORIENTED_EDGE('',*,*,#16513,.F.);
#22511=ORIENTED_EDGE('',*,*,#16512,.F.);
#22512=ORIENTED_EDGE('',*,*,#16506,.F.);
#22513=ORIENTED_EDGE('',*,*,#16514,.F.);
#22514=ORIENTED_EDGE('',*,*,#16515,.T.);
#22515=ORIENTED_EDGE('',*,*,#16516,.F.);
#22516=ORIENTED_EDGE('',*,*,#16517,.F.);
#22517=ORIENTED_EDGE('',*,*,#16518,.F.);
#22518=ORIENTED_EDGE('',*,*,#16517,.T.);
#22519=ORIENTED_EDGE('',*,*,#16519,.T.);
#22520=ORIENTED_EDGE('',*,*,#16520,.F.);
#22521=ORIENTED_EDGE('',*,*,#16519,.F.);
#22522=ORIENTED_EDGE('',*,*,#16516,.T.);
#22523=ORIENTED_EDGE('',*,*,#16521,.T.);
#22524=ORIENTED_EDGE('',*,*,#16522,.F.);
#22525=ORIENTED_EDGE('',*,*,#16521,.F.);
#22526=ORIENTED_EDGE('',*,*,#16515,.F.);
#22527=ORIENTED_EDGE('',*,*,#16523,.F.);
#22528=ORIENTED_EDGE('',*,*,#16524,.T.);
#22529=ORIENTED_EDGE('',*,*,#16525,.F.);
#22530=ORIENTED_EDGE('',*,*,#16526,.F.);
#22531=ORIENTED_EDGE('',*,*,#16527,.F.);
#22532=ORIENTED_EDGE('',*,*,#16526,.T.);
#22533=ORIENTED_EDGE('',*,*,#16528,.T.);
#22534=ORIENTED_EDGE('',*,*,#16529,.F.);
#22535=ORIENTED_EDGE('',*,*,#16530,.F.);
#22536=ORIENTED_EDGE('',*,*,#16528,.F.);
#22537=ORIENTED_EDGE('',*,*,#16525,.T.);
#22538=ORIENTED_EDGE('',*,*,#16531,.T.);
#22539=ORIENTED_EDGE('',*,*,#16532,.F.);
#22540=ORIENTED_EDGE('',*,*,#16531,.F.);
#22541=ORIENTED_EDGE('',*,*,#16524,.F.);
#22542=ORIENTED_EDGE('',*,*,#16533,.F.);
#22543=ORIENTED_EDGE('',*,*,#16534,.F.);
#22544=ORIENTED_EDGE('',*,*,#16535,.T.);
#22545=ORIENTED_EDGE('',*,*,#16536,.F.);
#22546=ORIENTED_EDGE('',*,*,#16537,.F.);
#22547=ORIENTED_EDGE('',*,*,#16538,.F.);
#22548=ORIENTED_EDGE('',*,*,#16537,.T.);
#22549=ORIENTED_EDGE('',*,*,#16539,.T.);
#22550=ORIENTED_EDGE('',*,*,#16540,.F.);
#22551=ORIENTED_EDGE('',*,*,#16539,.F.);
#22552=ORIENTED_EDGE('',*,*,#16536,.T.);
#22553=ORIENTED_EDGE('',*,*,#16541,.T.);
#22554=ORIENTED_EDGE('',*,*,#16542,.F.);
#22555=ORIENTED_EDGE('',*,*,#16541,.F.);
#22556=ORIENTED_EDGE('',*,*,#16535,.F.);
#22557=ORIENTED_EDGE('',*,*,#16543,.F.);
#22558=ORIENTED_EDGE('',*,*,#16544,.T.);
#22559=ORIENTED_EDGE('',*,*,#16545,.F.);
#22560=ORIENTED_EDGE('',*,*,#16546,.F.);
#22561=ORIENTED_EDGE('',*,*,#16547,.F.);
#22562=ORIENTED_EDGE('',*,*,#16546,.T.);
#22563=ORIENTED_EDGE('',*,*,#16548,.T.);
#22564=ORIENTED_EDGE('',*,*,#16549,.F.);
#22565=ORIENTED_EDGE('',*,*,#16548,.F.);
#22566=ORIENTED_EDGE('',*,*,#16545,.T.);
#22567=ORIENTED_EDGE('',*,*,#16550,.T.);
#22568=ORIENTED_EDGE('',*,*,#16551,.F.);
#22569=ORIENTED_EDGE('',*,*,#16550,.F.);
#22570=ORIENTED_EDGE('',*,*,#16544,.F.);
#22571=ORIENTED_EDGE('',*,*,#16552,.F.);
#22572=ORIENTED_EDGE('',*,*,#16553,.T.);
#22573=ORIENTED_EDGE('',*,*,#16554,.F.);
#22574=ORIENTED_EDGE('',*,*,#16555,.F.);
#22575=ORIENTED_EDGE('',*,*,#16556,.F.);
#22576=ORIENTED_EDGE('',*,*,#16555,.T.);
#22577=ORIENTED_EDGE('',*,*,#16557,.T.);
#22578=ORIENTED_EDGE('',*,*,#16558,.F.);
#22579=ORIENTED_EDGE('',*,*,#16557,.F.);
#22580=ORIENTED_EDGE('',*,*,#16554,.T.);
#22581=ORIENTED_EDGE('',*,*,#16559,.T.);
#22582=ORIENTED_EDGE('',*,*,#16560,.F.);
#22583=ORIENTED_EDGE('',*,*,#16559,.F.);
#22584=ORIENTED_EDGE('',*,*,#16553,.F.);
#22585=ORIENTED_EDGE('',*,*,#16561,.F.);
#22586=ORIENTED_EDGE('',*,*,#16562,.T.);
#22587=ORIENTED_EDGE('',*,*,#16563,.F.);
#22588=ORIENTED_EDGE('',*,*,#16564,.F.);
#22589=ORIENTED_EDGE('',*,*,#16565,.F.);
#22590=ORIENTED_EDGE('',*,*,#16564,.T.);
#22591=ORIENTED_EDGE('',*,*,#16566,.T.);
#22592=ORIENTED_EDGE('',*,*,#16567,.F.);
#22593=ORIENTED_EDGE('',*,*,#16566,.F.);
#22594=ORIENTED_EDGE('',*,*,#16563,.T.);
#22595=ORIENTED_EDGE('',*,*,#16568,.T.);
#22596=ORIENTED_EDGE('',*,*,#16569,.F.);
#22597=ORIENTED_EDGE('',*,*,#16568,.F.);
#22598=ORIENTED_EDGE('',*,*,#16562,.F.);
#22599=ORIENTED_EDGE('',*,*,#16570,.F.);
#22600=ORIENTED_EDGE('',*,*,#16571,.T.);
#22601=ORIENTED_EDGE('',*,*,#16572,.F.);
#22602=ORIENTED_EDGE('',*,*,#16573,.F.);
#22603=ORIENTED_EDGE('',*,*,#16574,.F.);
#22604=ORIENTED_EDGE('',*,*,#16573,.T.);
#22605=ORIENTED_EDGE('',*,*,#16575,.T.);
#22606=ORIENTED_EDGE('',*,*,#16576,.F.);
#22607=ORIENTED_EDGE('',*,*,#16575,.F.);
#22608=ORIENTED_EDGE('',*,*,#16572,.T.);
#22609=ORIENTED_EDGE('',*,*,#16577,.T.);
#22610=ORIENTED_EDGE('',*,*,#16578,.F.);
#22611=ORIENTED_EDGE('',*,*,#16577,.F.);
#22612=ORIENTED_EDGE('',*,*,#16571,.F.);
#22613=ORIENTED_EDGE('',*,*,#16579,.F.);
#22614=ORIENTED_EDGE('',*,*,#16580,.T.);
#22615=ORIENTED_EDGE('',*,*,#16581,.F.);
#22616=ORIENTED_EDGE('',*,*,#16582,.F.);
#22617=ORIENTED_EDGE('',*,*,#16583,.F.);
#22618=ORIENTED_EDGE('',*,*,#16582,.T.);
#22619=ORIENTED_EDGE('',*,*,#16584,.T.);
#22620=ORIENTED_EDGE('',*,*,#16585,.F.);
#22621=ORIENTED_EDGE('',*,*,#16584,.F.);
#22622=ORIENTED_EDGE('',*,*,#16581,.T.);
#22623=ORIENTED_EDGE('',*,*,#16586,.T.);
#22624=ORIENTED_EDGE('',*,*,#16587,.F.);
#22625=ORIENTED_EDGE('',*,*,#16586,.F.);
#22626=ORIENTED_EDGE('',*,*,#16580,.F.);
#22627=ORIENTED_EDGE('',*,*,#16588,.F.);
#22628=ORIENTED_EDGE('',*,*,#16589,.T.);
#22629=ORIENTED_EDGE('',*,*,#16590,.F.);
#22630=ORIENTED_EDGE('',*,*,#16591,.F.);
#22631=ORIENTED_EDGE('',*,*,#16592,.F.);
#22632=ORIENTED_EDGE('',*,*,#16591,.T.);
#22633=ORIENTED_EDGE('',*,*,#16593,.T.);
#22634=ORIENTED_EDGE('',*,*,#16594,.F.);
#22635=ORIENTED_EDGE('',*,*,#16593,.F.);
#22636=ORIENTED_EDGE('',*,*,#16590,.T.);
#22637=ORIENTED_EDGE('',*,*,#16595,.T.);
#22638=ORIENTED_EDGE('',*,*,#16596,.F.);
#22639=ORIENTED_EDGE('',*,*,#16595,.F.);
#22640=ORIENTED_EDGE('',*,*,#16589,.F.);
#22641=ORIENTED_EDGE('',*,*,#16597,.F.);
#22642=ORIENTED_EDGE('',*,*,#16598,.T.);
#22643=ORIENTED_EDGE('',*,*,#16599,.F.);
#22644=ORIENTED_EDGE('',*,*,#16600,.F.);
#22645=ORIENTED_EDGE('',*,*,#16601,.F.);
#22646=ORIENTED_EDGE('',*,*,#16600,.T.);
#22647=ORIENTED_EDGE('',*,*,#16602,.T.);
#22648=ORIENTED_EDGE('',*,*,#16603,.F.);
#22649=ORIENTED_EDGE('',*,*,#16602,.F.);
#22650=ORIENTED_EDGE('',*,*,#16599,.T.);
#22651=ORIENTED_EDGE('',*,*,#16604,.T.);
#22652=ORIENTED_EDGE('',*,*,#16605,.F.);
#22653=ORIENTED_EDGE('',*,*,#16604,.F.);
#22654=ORIENTED_EDGE('',*,*,#16598,.F.);
#22655=ORIENTED_EDGE('',*,*,#16606,.F.);
#22656=ORIENTED_EDGE('',*,*,#16607,.T.);
#22657=ORIENTED_EDGE('',*,*,#16608,.F.);
#22658=ORIENTED_EDGE('',*,*,#16609,.F.);
#22659=ORIENTED_EDGE('',*,*,#16610,.F.);
#22660=ORIENTED_EDGE('',*,*,#16609,.T.);
#22661=ORIENTED_EDGE('',*,*,#16611,.T.);
#22662=ORIENTED_EDGE('',*,*,#16612,.F.);
#22663=ORIENTED_EDGE('',*,*,#16611,.F.);
#22664=ORIENTED_EDGE('',*,*,#16608,.T.);
#22665=ORIENTED_EDGE('',*,*,#16613,.T.);
#22666=ORIENTED_EDGE('',*,*,#16614,.F.);
#22667=ORIENTED_EDGE('',*,*,#16613,.F.);
#22668=ORIENTED_EDGE('',*,*,#16607,.F.);
#22669=ORIENTED_EDGE('',*,*,#16615,.F.);
#22670=ORIENTED_EDGE('',*,*,#16616,.T.);
#22671=ORIENTED_EDGE('',*,*,#16617,.F.);
#22672=ORIENTED_EDGE('',*,*,#16618,.F.);
#22673=ORIENTED_EDGE('',*,*,#16619,.F.);
#22674=ORIENTED_EDGE('',*,*,#16618,.T.);
#22675=ORIENTED_EDGE('',*,*,#16620,.T.);
#22676=ORIENTED_EDGE('',*,*,#16621,.F.);
#22677=ORIENTED_EDGE('',*,*,#16620,.F.);
#22678=ORIENTED_EDGE('',*,*,#16617,.T.);
#22679=ORIENTED_EDGE('',*,*,#16622,.T.);
#22680=ORIENTED_EDGE('',*,*,#16623,.F.);
#22681=ORIENTED_EDGE('',*,*,#16622,.F.);
#22682=ORIENTED_EDGE('',*,*,#16616,.F.);
#22683=ORIENTED_EDGE('',*,*,#16624,.F.);
#22684=ORIENTED_EDGE('',*,*,#16625,.T.);
#22685=ORIENTED_EDGE('',*,*,#16626,.F.);
#22686=ORIENTED_EDGE('',*,*,#16627,.F.);
#22687=ORIENTED_EDGE('',*,*,#16628,.F.);
#22688=ORIENTED_EDGE('',*,*,#16627,.T.);
#22689=ORIENTED_EDGE('',*,*,#16629,.T.);
#22690=ORIENTED_EDGE('',*,*,#16630,.F.);
#22691=ORIENTED_EDGE('',*,*,#16629,.F.);
#22692=ORIENTED_EDGE('',*,*,#16626,.T.);
#22693=ORIENTED_EDGE('',*,*,#16631,.T.);
#22694=ORIENTED_EDGE('',*,*,#16632,.F.);
#22695=ORIENTED_EDGE('',*,*,#16631,.F.);
#22696=ORIENTED_EDGE('',*,*,#16625,.F.);
#22697=ORIENTED_EDGE('',*,*,#16633,.F.);
#22698=ORIENTED_EDGE('',*,*,#16634,.T.);
#22699=ORIENTED_EDGE('',*,*,#16635,.F.);
#22700=ORIENTED_EDGE('',*,*,#16636,.F.);
#22701=ORIENTED_EDGE('',*,*,#16637,.F.);
#22702=ORIENTED_EDGE('',*,*,#16636,.T.);
#22703=ORIENTED_EDGE('',*,*,#16638,.T.);
#22704=ORIENTED_EDGE('',*,*,#16639,.F.);
#22705=ORIENTED_EDGE('',*,*,#16638,.F.);
#22706=ORIENTED_EDGE('',*,*,#16635,.T.);
#22707=ORIENTED_EDGE('',*,*,#16640,.T.);
#22708=ORIENTED_EDGE('',*,*,#16641,.F.);
#22709=ORIENTED_EDGE('',*,*,#16640,.F.);
#22710=ORIENTED_EDGE('',*,*,#16634,.F.);
#22711=ORIENTED_EDGE('',*,*,#16642,.F.);
#22712=ORIENTED_EDGE('',*,*,#16643,.T.);
#22713=ORIENTED_EDGE('',*,*,#16644,.F.);
#22714=ORIENTED_EDGE('',*,*,#16645,.F.);
#22715=ORIENTED_EDGE('',*,*,#16646,.F.);
#22716=ORIENTED_EDGE('',*,*,#16645,.T.);
#22717=ORIENTED_EDGE('',*,*,#16647,.T.);
#22718=ORIENTED_EDGE('',*,*,#16648,.F.);
#22719=ORIENTED_EDGE('',*,*,#16647,.F.);
#22720=ORIENTED_EDGE('',*,*,#16644,.T.);
#22721=ORIENTED_EDGE('',*,*,#16649,.T.);
#22722=ORIENTED_EDGE('',*,*,#16650,.F.);
#22723=ORIENTED_EDGE('',*,*,#16649,.F.);
#22724=ORIENTED_EDGE('',*,*,#16643,.F.);
#22725=ORIENTED_EDGE('',*,*,#16651,.F.);
#22726=ORIENTED_EDGE('',*,*,#16652,.T.);
#22727=ORIENTED_EDGE('',*,*,#16653,.F.);
#22728=ORIENTED_EDGE('',*,*,#16654,.F.);
#22729=ORIENTED_EDGE('',*,*,#16655,.F.);
#22730=ORIENTED_EDGE('',*,*,#16654,.T.);
#22731=ORIENTED_EDGE('',*,*,#16656,.T.);
#22732=ORIENTED_EDGE('',*,*,#16657,.F.);
#22733=ORIENTED_EDGE('',*,*,#16656,.F.);
#22734=ORIENTED_EDGE('',*,*,#16653,.T.);
#22735=ORIENTED_EDGE('',*,*,#16658,.T.);
#22736=ORIENTED_EDGE('',*,*,#16659,.F.);
#22737=ORIENTED_EDGE('',*,*,#16658,.F.);
#22738=ORIENTED_EDGE('',*,*,#16652,.F.);
#22739=ORIENTED_EDGE('',*,*,#16660,.F.);
#22740=ORIENTED_EDGE('',*,*,#16661,.T.);
#22741=ORIENTED_EDGE('',*,*,#16662,.F.);
#22742=ORIENTED_EDGE('',*,*,#16663,.F.);
#22743=ORIENTED_EDGE('',*,*,#16664,.F.);
#22744=ORIENTED_EDGE('',*,*,#16663,.T.);
#22745=ORIENTED_EDGE('',*,*,#16665,.T.);
#22746=ORIENTED_EDGE('',*,*,#16666,.F.);
#22747=ORIENTED_EDGE('',*,*,#16665,.F.);
#22748=ORIENTED_EDGE('',*,*,#16662,.T.);
#22749=ORIENTED_EDGE('',*,*,#16667,.T.);
#22750=ORIENTED_EDGE('',*,*,#16668,.F.);
#22751=ORIENTED_EDGE('',*,*,#16667,.F.);
#22752=ORIENTED_EDGE('',*,*,#16661,.F.);
#22753=ORIENTED_EDGE('',*,*,#16669,.F.);
#22754=ORIENTED_EDGE('',*,*,#16670,.T.);
#22755=ORIENTED_EDGE('',*,*,#16671,.F.);
#22756=ORIENTED_EDGE('',*,*,#16672,.F.);
#22757=ORIENTED_EDGE('',*,*,#16673,.F.);
#22758=ORIENTED_EDGE('',*,*,#16672,.T.);
#22759=ORIENTED_EDGE('',*,*,#16674,.T.);
#22760=ORIENTED_EDGE('',*,*,#16675,.F.);
#22761=ORIENTED_EDGE('',*,*,#16674,.F.);
#22762=ORIENTED_EDGE('',*,*,#16671,.T.);
#22763=ORIENTED_EDGE('',*,*,#16676,.T.);
#22764=ORIENTED_EDGE('',*,*,#16677,.F.);
#22765=ORIENTED_EDGE('',*,*,#16676,.F.);
#22766=ORIENTED_EDGE('',*,*,#16670,.F.);
#22767=ORIENTED_EDGE('',*,*,#16678,.F.);
#22768=ORIENTED_EDGE('',*,*,#16679,.T.);
#22769=ORIENTED_EDGE('',*,*,#16680,.F.);
#22770=ORIENTED_EDGE('',*,*,#16681,.F.);
#22771=ORIENTED_EDGE('',*,*,#16682,.F.);
#22772=ORIENTED_EDGE('',*,*,#16681,.T.);
#22773=ORIENTED_EDGE('',*,*,#16683,.T.);
#22774=ORIENTED_EDGE('',*,*,#16684,.F.);
#22775=ORIENTED_EDGE('',*,*,#16683,.F.);
#22776=ORIENTED_EDGE('',*,*,#16680,.T.);
#22777=ORIENTED_EDGE('',*,*,#16685,.T.);
#22778=ORIENTED_EDGE('',*,*,#16686,.F.);
#22779=ORIENTED_EDGE('',*,*,#16685,.F.);
#22780=ORIENTED_EDGE('',*,*,#16679,.F.);
#22781=ORIENTED_EDGE('',*,*,#16687,.F.);
#22782=ORIENTED_EDGE('',*,*,#16688,.T.);
#22783=ORIENTED_EDGE('',*,*,#16689,.F.);
#22784=ORIENTED_EDGE('',*,*,#16690,.F.);
#22785=ORIENTED_EDGE('',*,*,#16691,.F.);
#22786=ORIENTED_EDGE('',*,*,#16690,.T.);
#22787=ORIENTED_EDGE('',*,*,#16692,.T.);
#22788=ORIENTED_EDGE('',*,*,#16693,.F.);
#22789=ORIENTED_EDGE('',*,*,#16692,.F.);
#22790=ORIENTED_EDGE('',*,*,#16689,.T.);
#22791=ORIENTED_EDGE('',*,*,#16694,.T.);
#22792=ORIENTED_EDGE('',*,*,#16695,.F.);
#22793=ORIENTED_EDGE('',*,*,#16694,.F.);
#22794=ORIENTED_EDGE('',*,*,#16688,.F.);
#22795=ORIENTED_EDGE('',*,*,#16696,.T.);
#22796=ORIENTED_EDGE('',*,*,#16697,.F.);
#22797=ORIENTED_EDGE('',*,*,#16696,.F.);
#22798=ORIENTED_EDGE('',*,*,#16698,.F.);
#22799=ORIENTED_EDGE('',*,*,#16699,.T.);
#22800=ORIENTED_EDGE('',*,*,#16700,.T.);
#22801=ORIENTED_EDGE('',*,*,#16701,.F.);
#22802=ORIENTED_EDGE('',*,*,#16702,.F.);
#22803=ORIENTED_EDGE('',*,*,#16703,.T.);
#22804=ORIENTED_EDGE('',*,*,#16704,.T.);
#22805=ORIENTED_EDGE('',*,*,#16699,.F.);
#22806=ORIENTED_EDGE('',*,*,#16705,.F.);
#22807=ORIENTED_EDGE('',*,*,#16706,.T.);
#22808=ORIENTED_EDGE('',*,*,#16707,.T.);
#22809=ORIENTED_EDGE('',*,*,#16703,.F.);
#22810=ORIENTED_EDGE('',*,*,#16708,.F.);
#22811=ORIENTED_EDGE('',*,*,#16709,.T.);
#22812=ORIENTED_EDGE('',*,*,#16710,.T.);
#22813=ORIENTED_EDGE('',*,*,#16706,.F.);
#22814=ORIENTED_EDGE('',*,*,#16711,.F.);
#22815=ORIENTED_EDGE('',*,*,#16712,.T.);
#22816=ORIENTED_EDGE('',*,*,#16713,.T.);
#22817=ORIENTED_EDGE('',*,*,#16709,.F.);
#22818=ORIENTED_EDGE('',*,*,#16714,.F.);
#22819=ORIENTED_EDGE('',*,*,#16701,.T.);
#22820=ORIENTED_EDGE('',*,*,#16715,.T.);
#22821=ORIENTED_EDGE('',*,*,#16712,.F.);
#22822=ORIENTED_EDGE('',*,*,#16715,.F.);
#22823=ORIENTED_EDGE('',*,*,#16700,.F.);
#22824=ORIENTED_EDGE('',*,*,#16704,.F.);
#22825=ORIENTED_EDGE('',*,*,#16707,.F.);
#22826=ORIENTED_EDGE('',*,*,#16710,.F.);
#22827=ORIENTED_EDGE('',*,*,#16713,.F.);
#22828=ORIENTED_EDGE('',*,*,#16697,.T.);
#22829=ORIENTED_EDGE('',*,*,#16716,.T.);
#22830=ORIENTED_EDGE('',*,*,#16717,.T.);
#22831=ORIENTED_EDGE('',*,*,#16718,.T.);
#22832=ORIENTED_EDGE('',*,*,#16717,.F.);
#22833=ORIENTED_EDGE('',*,*,#16719,.T.);
#22834=ORIENTED_EDGE('',*,*,#16716,.F.);
#22835=ORIENTED_EDGE('',*,*,#16720,.T.);
#22836=ORIENTED_EDGE('',*,*,#16721,.T.);
#22837=ORIENTED_EDGE('',*,*,#16720,.F.);
#22838=ORIENTED_EDGE('',*,*,#16719,.F.);
#22839=ORIENTED_EDGE('',*,*,#16722,.F.);
#22840=ORIENTED_EDGE('',*,*,#16718,.F.);
#22841=ORIENTED_EDGE('',*,*,#16723,.F.);
#22842=ORIENTED_EDGE('',*,*,#16364,.F.);
#22843=ORIENTED_EDGE('',*,*,#16297,.F.);
#22844=ORIENTED_EDGE('',*,*,#16365,.F.);
#22845=ORIENTED_EDGE('',*,*,#16724,.T.);
#22846=ORIENTED_EDGE('',*,*,#16723,.T.);
#22847=ORIENTED_EDGE('',*,*,#16724,.F.);
#22848=ORIENTED_EDGE('',*,*,#16323,.T.);
#22849=ORIENTED_EDGE('',*,*,#16361,.T.);
#22850=ORIENTED_EDGE('',*,*,#16725,.F.);
#22851=ORIENTED_EDGE('',*,*,#16369,.T.);
#22852=ORIENTED_EDGE('',*,*,#16726,.F.);
#22853=ORIENTED_EDGE('',*,*,#16727,.T.);
#22854=ORIENTED_EDGE('',*,*,#16358,.T.);
#22855=ORIENTED_EDGE('',*,*,#16725,.T.);
#22856=ORIENTED_EDGE('',*,*,#16359,.T.);
#22857=ORIENTED_EDGE('',*,*,#16727,.F.);
#22858=ORIENTED_EDGE('',*,*,#16728,.F.);
#22859=ORIENTED_EDGE('',*,*,#16729,.T.);
#22860=ORIENTED_EDGE('',*,*,#16726,.T.);
#22861=ORIENTED_EDGE('',*,*,#16729,.F.);
#22862=ORIENTED_EDGE('',*,*,#16721,.F.);
#22863=ORIENTED_EDGE('',*,*,#16728,.T.);
#22864=ORIENTED_EDGE('',*,*,#16730,.F.);
#22865=ORIENTED_EDGE('',*,*,#16731,.T.);
#22866=ORIENTED_EDGE('',*,*,#16533,.T.);
#22867=ORIENTED_EDGE('',*,*,#16523,.T.);
#22868=ORIENTED_EDGE('',*,*,#16527,.T.);
#22869=ORIENTED_EDGE('',*,*,#16732,.T.);
#22870=ORIENTED_EDGE('',*,*,#16722,.T.);
#22871=ORIENTED_EDGE('',*,*,#16732,.F.);
#22872=ORIENTED_EDGE('',*,*,#16529,.T.);
#22873=ORIENTED_EDGE('',*,*,#16530,.T.);
#22874=ORIENTED_EDGE('',*,*,#16532,.T.);
#22875=ORIENTED_EDGE('',*,*,#16731,.F.);
#22876=ORIENTED_EDGE('',*,*,#16376,.T.);
#22877=ORIENTED_EDGE('',*,*,#16378,.T.);
#22878=ORIENTED_EDGE('',*,*,#16370,.T.);
#22879=ORIENTED_EDGE('',*,*,#16374,.T.);
#22880=ORIENTED_EDGE('',*,*,#16385,.T.);
#22881=ORIENTED_EDGE('',*,*,#16387,.T.);
#22882=ORIENTED_EDGE('',*,*,#16379,.T.);
#22883=ORIENTED_EDGE('',*,*,#16383,.T.);
#22884=ORIENTED_EDGE('',*,*,#16394,.T.);
#22885=ORIENTED_EDGE('',*,*,#16396,.T.);
#22886=ORIENTED_EDGE('',*,*,#16388,.T.);
#22887=ORIENTED_EDGE('',*,*,#16392,.T.);
#22888=ORIENTED_EDGE('',*,*,#16403,.T.);
#22889=ORIENTED_EDGE('',*,*,#16405,.T.);
#22890=ORIENTED_EDGE('',*,*,#16397,.T.);
#22891=ORIENTED_EDGE('',*,*,#16401,.T.);
#22892=ORIENTED_EDGE('',*,*,#16412,.T.);
#22893=ORIENTED_EDGE('',*,*,#16414,.T.);
#22894=ORIENTED_EDGE('',*,*,#16406,.T.);
#22895=ORIENTED_EDGE('',*,*,#16410,.T.);
#22896=ORIENTED_EDGE('',*,*,#16421,.T.);
#22897=ORIENTED_EDGE('',*,*,#16423,.T.);
#22898=ORIENTED_EDGE('',*,*,#16415,.T.);
#22899=ORIENTED_EDGE('',*,*,#16419,.T.);
#22900=ORIENTED_EDGE('',*,*,#16430,.T.);
#22901=ORIENTED_EDGE('',*,*,#16432,.T.);
#22902=ORIENTED_EDGE('',*,*,#16424,.T.);
#22903=ORIENTED_EDGE('',*,*,#16428,.T.);
#22904=ORIENTED_EDGE('',*,*,#16439,.T.);
#22905=ORIENTED_EDGE('',*,*,#16441,.T.);
#22906=ORIENTED_EDGE('',*,*,#16433,.T.);
#22907=ORIENTED_EDGE('',*,*,#16437,.T.);
#22908=ORIENTED_EDGE('',*,*,#16448,.T.);
#22909=ORIENTED_EDGE('',*,*,#16450,.T.);
#22910=ORIENTED_EDGE('',*,*,#16442,.T.);
#22911=ORIENTED_EDGE('',*,*,#16446,.T.);
#22912=ORIENTED_EDGE('',*,*,#16457,.T.);
#22913=ORIENTED_EDGE('',*,*,#16459,.T.);
#22914=ORIENTED_EDGE('',*,*,#16451,.T.);
#22915=ORIENTED_EDGE('',*,*,#16455,.T.);
#22916=ORIENTED_EDGE('',*,*,#16466,.T.);
#22917=ORIENTED_EDGE('',*,*,#16468,.T.);
#22918=ORIENTED_EDGE('',*,*,#16460,.T.);
#22919=ORIENTED_EDGE('',*,*,#16464,.T.);
#22920=ORIENTED_EDGE('',*,*,#16475,.T.);
#22921=ORIENTED_EDGE('',*,*,#16477,.T.);
#22922=ORIENTED_EDGE('',*,*,#16469,.T.);
#22923=ORIENTED_EDGE('',*,*,#16473,.T.);
#22924=ORIENTED_EDGE('',*,*,#16484,.T.);
#22925=ORIENTED_EDGE('',*,*,#16486,.T.);
#22926=ORIENTED_EDGE('',*,*,#16478,.T.);
#22927=ORIENTED_EDGE('',*,*,#16482,.T.);
#22928=ORIENTED_EDGE('',*,*,#16493,.T.);
#22929=ORIENTED_EDGE('',*,*,#16495,.T.);
#22930=ORIENTED_EDGE('',*,*,#16487,.T.);
#22931=ORIENTED_EDGE('',*,*,#16491,.T.);
#22932=ORIENTED_EDGE('',*,*,#16502,.T.);
#22933=ORIENTED_EDGE('',*,*,#16504,.T.);
#22934=ORIENTED_EDGE('',*,*,#16496,.T.);
#22935=ORIENTED_EDGE('',*,*,#16500,.T.);
#22936=ORIENTED_EDGE('',*,*,#16511,.T.);
#22937=ORIENTED_EDGE('',*,*,#16513,.T.);
#22938=ORIENTED_EDGE('',*,*,#16505,.T.);
#22939=ORIENTED_EDGE('',*,*,#16509,.T.);
#22940=ORIENTED_EDGE('',*,*,#16520,.T.);
#22941=ORIENTED_EDGE('',*,*,#16522,.T.);
#22942=ORIENTED_EDGE('',*,*,#16514,.T.);
#22943=ORIENTED_EDGE('',*,*,#16518,.T.);
#22944=ORIENTED_EDGE('',*,*,#16540,.T.);
#22945=ORIENTED_EDGE('',*,*,#16542,.T.);
#22946=ORIENTED_EDGE('',*,*,#16534,.T.);
#22947=ORIENTED_EDGE('',*,*,#16538,.T.);
#22948=ORIENTED_EDGE('',*,*,#16549,.T.);
#22949=ORIENTED_EDGE('',*,*,#16551,.T.);
#22950=ORIENTED_EDGE('',*,*,#16543,.T.);
#22951=ORIENTED_EDGE('',*,*,#16547,.T.);
#22952=ORIENTED_EDGE('',*,*,#16558,.T.);
#22953=ORIENTED_EDGE('',*,*,#16560,.T.);
#22954=ORIENTED_EDGE('',*,*,#16552,.T.);
#22955=ORIENTED_EDGE('',*,*,#16556,.T.);
#22956=ORIENTED_EDGE('',*,*,#16567,.T.);
#22957=ORIENTED_EDGE('',*,*,#16569,.T.);
#22958=ORIENTED_EDGE('',*,*,#16561,.T.);
#22959=ORIENTED_EDGE('',*,*,#16565,.T.);
#22960=ORIENTED_EDGE('',*,*,#16576,.T.);
#22961=ORIENTED_EDGE('',*,*,#16578,.T.);
#22962=ORIENTED_EDGE('',*,*,#16570,.T.);
#22963=ORIENTED_EDGE('',*,*,#16574,.T.);
#22964=ORIENTED_EDGE('',*,*,#16585,.T.);
#22965=ORIENTED_EDGE('',*,*,#16587,.T.);
#22966=ORIENTED_EDGE('',*,*,#16579,.T.);
#22967=ORIENTED_EDGE('',*,*,#16583,.T.);
#22968=ORIENTED_EDGE('',*,*,#16594,.T.);
#22969=ORIENTED_EDGE('',*,*,#16596,.T.);
#22970=ORIENTED_EDGE('',*,*,#16588,.T.);
#22971=ORIENTED_EDGE('',*,*,#16592,.T.);
#22972=ORIENTED_EDGE('',*,*,#16603,.T.);
#22973=ORIENTED_EDGE('',*,*,#16605,.T.);
#22974=ORIENTED_EDGE('',*,*,#16597,.T.);
#22975=ORIENTED_EDGE('',*,*,#16601,.T.);
#22976=ORIENTED_EDGE('',*,*,#16612,.T.);
#22977=ORIENTED_EDGE('',*,*,#16614,.T.);
#22978=ORIENTED_EDGE('',*,*,#16606,.T.);
#22979=ORIENTED_EDGE('',*,*,#16610,.T.);
#22980=ORIENTED_EDGE('',*,*,#16621,.T.);
#22981=ORIENTED_EDGE('',*,*,#16623,.T.);
#22982=ORIENTED_EDGE('',*,*,#16615,.T.);
#22983=ORIENTED_EDGE('',*,*,#16619,.T.);
#22984=ORIENTED_EDGE('',*,*,#16630,.T.);
#22985=ORIENTED_EDGE('',*,*,#16632,.T.);
#22986=ORIENTED_EDGE('',*,*,#16624,.T.);
#22987=ORIENTED_EDGE('',*,*,#16628,.T.);
#22988=ORIENTED_EDGE('',*,*,#16639,.T.);
#22989=ORIENTED_EDGE('',*,*,#16641,.T.);
#22990=ORIENTED_EDGE('',*,*,#16633,.T.);
#22991=ORIENTED_EDGE('',*,*,#16637,.T.);
#22992=ORIENTED_EDGE('',*,*,#16648,.T.);
#22993=ORIENTED_EDGE('',*,*,#16650,.T.);
#22994=ORIENTED_EDGE('',*,*,#16642,.T.);
#22995=ORIENTED_EDGE('',*,*,#16646,.T.);
#22996=ORIENTED_EDGE('',*,*,#16657,.T.);
#22997=ORIENTED_EDGE('',*,*,#16659,.T.);
#22998=ORIENTED_EDGE('',*,*,#16651,.T.);
#22999=ORIENTED_EDGE('',*,*,#16655,.T.);
#23000=ORIENTED_EDGE('',*,*,#16666,.T.);
#23001=ORIENTED_EDGE('',*,*,#16668,.T.);
#23002=ORIENTED_EDGE('',*,*,#16660,.T.);
#23003=ORIENTED_EDGE('',*,*,#16664,.T.);
#23004=ORIENTED_EDGE('',*,*,#16675,.T.);
#23005=ORIENTED_EDGE('',*,*,#16677,.T.);
#23006=ORIENTED_EDGE('',*,*,#16669,.T.);
#23007=ORIENTED_EDGE('',*,*,#16673,.T.);
#23008=ORIENTED_EDGE('',*,*,#16684,.T.);
#23009=ORIENTED_EDGE('',*,*,#16686,.T.);
#23010=ORIENTED_EDGE('',*,*,#16678,.T.);
#23011=ORIENTED_EDGE('',*,*,#16682,.T.);
#23012=ORIENTED_EDGE('',*,*,#16693,.T.);
#23013=ORIENTED_EDGE('',*,*,#16695,.T.);
#23014=ORIENTED_EDGE('',*,*,#16687,.T.);
#23015=ORIENTED_EDGE('',*,*,#16691,.T.);
#23016=ORIENTED_EDGE('',*,*,#16733,.F.);
#23017=ORIENTED_EDGE('',*,*,#16734,.T.);
#23018=ORIENTED_EDGE('',*,*,#16730,.T.);
#23019=ORIENTED_EDGE('',*,*,#16734,.F.);
#23020=ORIENTED_EDGE('',*,*,#16733,.T.);
#23021=ORIENTED_EDGE('',*,*,#16698,.T.);
#23022=ORIENTED_EDGE('',*,*,#16714,.T.);
#23023=ORIENTED_EDGE('',*,*,#16711,.T.);
#23024=ORIENTED_EDGE('',*,*,#16708,.T.);
#23025=ORIENTED_EDGE('',*,*,#16705,.T.);
#23026=ORIENTED_EDGE('',*,*,#16702,.T.);
#28313=PLANE('',#31807);
#28314=PLANE('',#31810);
#28315=PLANE('',#31815);
#28316=PLANE('',#31816);
#28317=PLANE('',#31818);
#28318=PLANE('',#31819);
#28319=PLANE('',#31821);
#28320=PLANE('',#31822);
#28321=PLANE('',#31824);
#28322=PLANE('',#31825);
#28323=PLANE('',#31827);
#28324=PLANE('',#31828);
#28325=PLANE('',#31830);
#28326=PLANE('',#31831);
#28327=PLANE('',#31833);
#28328=PLANE('',#31834);
#28329=PLANE('',#31836);
#28330=PLANE('',#31837);
#28331=PLANE('',#31839);
#28332=PLANE('',#31840);
#28333=PLANE('',#31842);
#28334=PLANE('',#31843);
#28335=PLANE('',#31845);
#28336=PLANE('',#31846);
#28337=PLANE('',#31848);
#28338=PLANE('',#31849);
#28339=PLANE('',#31851);
#28340=PLANE('',#31852);
#28341=PLANE('',#31854);
#28342=PLANE('',#31855);
#28343=PLANE('',#31857);
#28344=PLANE('',#31858);
#28345=PLANE('',#31860);
#28346=PLANE('',#31861);
#28347=PLANE('',#31863);
#28348=PLANE('',#31864);
#28349=PLANE('',#31866);
#28350=PLANE('',#31867);
#28351=PLANE('',#31869);
#28352=PLANE('',#31870);
#28353=PLANE('',#31872);
#28354=PLANE('',#31873);
#28355=PLANE('',#31875);
#28356=PLANE('',#31876);
#28357=PLANE('',#31878);
#28358=PLANE('',#31879);
#28359=PLANE('',#31881);
#28360=PLANE('',#31882);
#28361=PLANE('',#31884);
#28362=PLANE('',#31885);
#28363=PLANE('',#31887);
#28364=PLANE('',#31888);
#28365=PLANE('',#31890);
#28366=PLANE('',#31891);
#28367=PLANE('',#31893);
#28368=PLANE('',#31894);
#28369=PLANE('',#31896);
#28370=PLANE('',#31897);
#28371=PLANE('',#31899);
#28372=PLANE('',#31900);
#28373=PLANE('',#31902);
#28374=PLANE('',#31903);
#28375=PLANE('',#31905);
#28376=PLANE('',#31906);
#28377=PLANE('',#31908);
#28378=PLANE('',#31909);
#28379=PLANE('',#31911);
#28380=PLANE('',#31912);
#28381=PLANE('',#31914);
#28382=PLANE('',#31915);
#28383=PLANE('',#31917);
#28384=PLANE('',#31918);
#28385=PLANE('',#31921);
#28386=PLANE('',#31922);
#28387=PLANE('',#31925);
#28388=PLANE('',#31926);
#28389=PLANE('',#31928);
#28390=PLANE('',#31929);
#28391=PLANE('',#31931);
#28392=PLANE('',#31932);
#28393=PLANE('',#31934);
#28394=PLANE('',#31935);
#28395=PLANE('',#31937);
#28396=PLANE('',#31938);
#28397=PLANE('',#31940);
#28398=PLANE('',#31941);
#28399=PLANE('',#31943);
#28400=PLANE('',#31944);
#28401=PLANE('',#31946);
#28402=PLANE('',#31947);
#28403=PLANE('',#31949);
#28404=PLANE('',#31950);
#28405=PLANE('',#31952);
#28406=PLANE('',#31953);
#28407=PLANE('',#31955);
#28408=PLANE('',#31956);
#28409=PLANE('',#31958);
#28410=PLANE('',#31959);
#28411=PLANE('',#31961);
#28412=PLANE('',#31962);
#28413=PLANE('',#31964);
#28414=PLANE('',#31965);
#28415=PLANE('',#31967);
#28416=PLANE('',#31968);
#28417=PLANE('',#31970);
#28418=PLANE('',#31971);
#28419=PLANE('',#31973);
#28420=PLANE('',#31974);
#28421=PLANE('',#31976);
#28422=PLANE('',#31977);
#28423=PLANE('',#31979);
#28424=PLANE('',#31980);
#28425=PLANE('',#31982);
#28426=PLANE('',#31983);
#28427=PLANE('',#31985);
#28428=PLANE('',#31986);
#28429=PLANE('',#31988);
#28430=PLANE('',#31989);
#28431=PLANE('',#31991);
#28432=PLANE('',#31992);
#28433=PLANE('',#31994);
#28434=PLANE('',#31995);
#28435=PLANE('',#31997);
#28436=PLANE('',#31998);
#28437=PLANE('',#32000);
#28438=PLANE('',#32001);
#28439=PLANE('',#32003);
#28440=PLANE('',#32004);
#28441=PLANE('',#32006);
#28442=PLANE('',#32007);
#28443=PLANE('',#32009);
#28444=PLANE('',#32010);
#28445=PLANE('',#32012);
#28446=PLANE('',#32013);
#28447=PLANE('',#32015);
#28448=PLANE('',#32016);
#28449=PLANE('',#32018);
#28450=PLANE('',#32019);
#28451=PLANE('',#32021);
#28452=PLANE('',#32022);
#28453=PLANE('',#32024);
#28454=PLANE('',#32025);
#28455=PLANE('',#32027);
#28456=PLANE('',#32028);
#28457=PLANE('',#32030);
#28458=PLANE('',#32031);
#28459=PLANE('',#32035);
#28460=PLANE('',#32036);
#28461=PLANE('',#32037);
#28462=PLANE('',#32038);
#28463=PLANE('',#32039);
#28464=PLANE('',#32040);
#28465=PLANE('',#32041);
#28466=PLANE('',#32049);
#28467=PLANE('',#32051);
#28468=PLANE('',#32060);
#28469=PLANE('',#32065);
#29510=ADVANCED_FACE('',(#4182),#548,.T.);
#29511=ADVANCED_FACE('',(#4183),#549,.T.);
#29512=ADVANCED_FACE('',(#4184),#550,.T.);
#29513=ADVANCED_FACE('',(#4185),#551,.T.);
#29514=ADVANCED_FACE('',(#4186),#552,.T.);
#29515=ADVANCED_FACE('',(#4187),#553,.T.);
#29516=ADVANCED_FACE('',(#4188),#554,.T.);
#29517=ADVANCED_FACE('',(#4189),#555,.T.);
#29518=ADVANCED_FACE('',(#4190),#556,.T.);
#29519=ADVANCED_FACE('',(#4191),#557,.T.);
#29520=ADVANCED_FACE('',(#4192),#558,.T.);
#29521=ADVANCED_FACE('',(#4193),#559,.T.);
#29522=ADVANCED_FACE('',(#4194),#560,.T.);
#29523=ADVANCED_FACE('',(#4195),#561,.T.);
#29524=ADVANCED_FACE('',(#4196),#562,.T.);
#29525=ADVANCED_FACE('',(#4197),#563,.T.);
#29526=ADVANCED_FACE('',(#4198),#564,.T.);
#29527=ADVANCED_FACE('',(#4199),#565,.T.);
#29528=ADVANCED_FACE('',(#4200),#566,.T.);
#29529=ADVANCED_FACE('',(#4201),#567,.T.);
#29530=ADVANCED_FACE('',(#4202),#28313,.F.);
#29531=ADVANCED_FACE('',(#4203),#419,.F.);
#29532=ADVANCED_FACE('',(#4204),#28314,.T.);
#29533=ADVANCED_FACE('',(#4205),#568,.T.);
#29534=ADVANCED_FACE('',(#4206),#420,.F.);
#29535=ADVANCED_FACE('',(#4207),#28315,.F.);
#29536=ADVANCED_FACE('',(#4208),#28316,.T.);
#29537=ADVANCED_FACE('',(#4209),#28317,.F.);
#29538=ADVANCED_FACE('',(#4210),#28318,.F.);
#29539=ADVANCED_FACE('',(#4211),#28319,.F.);
#29540=ADVANCED_FACE('',(#4212),#28320,.T.);
#29541=ADVANCED_FACE('',(#4213),#28321,.F.);
#29542=ADVANCED_FACE('',(#4214),#28322,.F.);
#29543=ADVANCED_FACE('',(#4215),#28323,.F.);
#29544=ADVANCED_FACE('',(#4216),#28324,.T.);
#29545=ADVANCED_FACE('',(#4217),#28325,.F.);
#29546=ADVANCED_FACE('',(#4218),#28326,.F.);
#29547=ADVANCED_FACE('',(#4219),#28327,.F.);
#29548=ADVANCED_FACE('',(#4220),#28328,.T.);
#29549=ADVANCED_FACE('',(#4221),#28329,.F.);
#29550=ADVANCED_FACE('',(#4222),#28330,.F.);
#29551=ADVANCED_FACE('',(#4223),#28331,.F.);
#29552=ADVANCED_FACE('',(#4224),#28332,.T.);
#29553=ADVANCED_FACE('',(#4225),#28333,.F.);
#29554=ADVANCED_FACE('',(#4226),#28334,.F.);
#29555=ADVANCED_FACE('',(#4227),#28335,.F.);
#29556=ADVANCED_FACE('',(#4228),#28336,.T.);
#29557=ADVANCED_FACE('',(#4229),#28337,.F.);
#29558=ADVANCED_FACE('',(#4230),#28338,.F.);
#29559=ADVANCED_FACE('',(#4231),#28339,.F.);
#29560=ADVANCED_FACE('',(#4232),#28340,.T.);
#29561=ADVANCED_FACE('',(#4233),#28341,.F.);
#29562=ADVANCED_FACE('',(#4234),#28342,.F.);
#29563=ADVANCED_FACE('',(#4235),#28343,.F.);
#29564=ADVANCED_FACE('',(#4236),#28344,.T.);
#29565=ADVANCED_FACE('',(#4237),#28345,.F.);
#29566=ADVANCED_FACE('',(#4238),#28346,.F.);
#29567=ADVANCED_FACE('',(#4239),#28347,.F.);
#29568=ADVANCED_FACE('',(#4240),#28348,.T.);
#29569=ADVANCED_FACE('',(#4241),#28349,.F.);
#29570=ADVANCED_FACE('',(#4242),#28350,.F.);
#29571=ADVANCED_FACE('',(#4243),#28351,.F.);
#29572=ADVANCED_FACE('',(#4244),#28352,.T.);
#29573=ADVANCED_FACE('',(#4245),#28353,.F.);
#29574=ADVANCED_FACE('',(#4246),#28354,.F.);
#29575=ADVANCED_FACE('',(#4247),#28355,.F.);
#29576=ADVANCED_FACE('',(#4248),#28356,.T.);
#29577=ADVANCED_FACE('',(#4249),#28357,.F.);
#29578=ADVANCED_FACE('',(#4250),#28358,.F.);
#29579=ADVANCED_FACE('',(#4251),#28359,.F.);
#29580=ADVANCED_FACE('',(#4252),#28360,.T.);
#29581=ADVANCED_FACE('',(#4253),#28361,.F.);
#29582=ADVANCED_FACE('',(#4254),#28362,.F.);
#29583=ADVANCED_FACE('',(#4255),#28363,.F.);
#29584=ADVANCED_FACE('',(#4256),#28364,.T.);
#29585=ADVANCED_FACE('',(#4257),#28365,.F.);
#29586=ADVANCED_FACE('',(#4258),#28366,.F.);
#29587=ADVANCED_FACE('',(#4259),#28367,.F.);
#29588=ADVANCED_FACE('',(#4260),#28368,.T.);
#29589=ADVANCED_FACE('',(#4261),#28369,.F.);
#29590=ADVANCED_FACE('',(#4262),#28370,.F.);
#29591=ADVANCED_FACE('',(#4263),#28371,.F.);
#29592=ADVANCED_FACE('',(#4264),#28372,.T.);
#29593=ADVANCED_FACE('',(#4265),#28373,.F.);
#29594=ADVANCED_FACE('',(#4266),#28374,.F.);
#29595=ADVANCED_FACE('',(#4267),#28375,.F.);
#29596=ADVANCED_FACE('',(#4268),#28376,.T.);
#29597=ADVANCED_FACE('',(#4269),#28377,.F.);
#29598=ADVANCED_FACE('',(#4270),#28378,.F.);
#29599=ADVANCED_FACE('',(#4271),#28379,.F.);
#29600=ADVANCED_FACE('',(#4272),#28380,.T.);
#29601=ADVANCED_FACE('',(#4273),#28381,.F.);
#29602=ADVANCED_FACE('',(#4274),#28382,.F.);
#29603=ADVANCED_FACE('',(#4275),#28383,.F.);
#29604=ADVANCED_FACE('',(#4276),#28384,.T.);
#29605=ADVANCED_FACE('',(#4277),#28385,.F.);
#29606=ADVANCED_FACE('',(#4278),#28386,.F.);
#29607=ADVANCED_FACE('',(#4279),#28387,.F.);
#29608=ADVANCED_FACE('',(#4280),#28388,.T.);
#29609=ADVANCED_FACE('',(#4281),#28389,.F.);
#29610=ADVANCED_FACE('',(#4282),#28390,.F.);
#29611=ADVANCED_FACE('',(#4283),#28391,.F.);
#29612=ADVANCED_FACE('',(#4284),#28392,.T.);
#29613=ADVANCED_FACE('',(#4285),#28393,.F.);
#29614=ADVANCED_FACE('',(#4286),#28394,.F.);
#29615=ADVANCED_FACE('',(#4287),#28395,.F.);
#29616=ADVANCED_FACE('',(#4288),#28396,.T.);
#29617=ADVANCED_FACE('',(#4289),#28397,.F.);
#29618=ADVANCED_FACE('',(#4290),#28398,.F.);
#29619=ADVANCED_FACE('',(#4291),#28399,.F.);
#29620=ADVANCED_FACE('',(#4292),#28400,.T.);
#29621=ADVANCED_FACE('',(#4293),#28401,.F.);
#29622=ADVANCED_FACE('',(#4294),#28402,.F.);
#29623=ADVANCED_FACE('',(#4295),#28403,.F.);
#29624=ADVANCED_FACE('',(#4296),#28404,.T.);
#29625=ADVANCED_FACE('',(#4297),#28405,.F.);
#29626=ADVANCED_FACE('',(#4298),#28406,.F.);
#29627=ADVANCED_FACE('',(#4299),#28407,.F.);
#29628=ADVANCED_FACE('',(#4300),#28408,.T.);
#29629=ADVANCED_FACE('',(#4301),#28409,.F.);
#29630=ADVANCED_FACE('',(#4302),#28410,.F.);
#29631=ADVANCED_FACE('',(#4303),#28411,.F.);
#29632=ADVANCED_FACE('',(#4304),#28412,.T.);
#29633=ADVANCED_FACE('',(#4305),#28413,.F.);
#29634=ADVANCED_FACE('',(#4306),#28414,.F.);
#29635=ADVANCED_FACE('',(#4307),#28415,.F.);
#29636=ADVANCED_FACE('',(#4308),#28416,.T.);
#29637=ADVANCED_FACE('',(#4309),#28417,.F.);
#29638=ADVANCED_FACE('',(#4310),#28418,.F.);
#29639=ADVANCED_FACE('',(#4311),#28419,.F.);
#29640=ADVANCED_FACE('',(#4312),#28420,.T.);
#29641=ADVANCED_FACE('',(#4313),#28421,.F.);
#29642=ADVANCED_FACE('',(#4314),#28422,.F.);
#29643=ADVANCED_FACE('',(#4315),#28423,.F.);
#29644=ADVANCED_FACE('',(#4316),#28424,.T.);
#29645=ADVANCED_FACE('',(#4317),#28425,.F.);
#29646=ADVANCED_FACE('',(#4318),#28426,.F.);
#29647=ADVANCED_FACE('',(#4319),#28427,.F.);
#29648=ADVANCED_FACE('',(#4320),#28428,.T.);
#29649=ADVANCED_FACE('',(#4321),#28429,.F.);
#29650=ADVANCED_FACE('',(#4322),#28430,.F.);
#29651=ADVANCED_FACE('',(#4323),#28431,.F.);
#29652=ADVANCED_FACE('',(#4324),#28432,.T.);
#29653=ADVANCED_FACE('',(#4325),#28433,.F.);
#29654=ADVANCED_FACE('',(#4326),#28434,.F.);
#29655=ADVANCED_FACE('',(#4327),#28435,.F.);
#29656=ADVANCED_FACE('',(#4328),#28436,.T.);
#29657=ADVANCED_FACE('',(#4329),#28437,.F.);
#29658=ADVANCED_FACE('',(#4330),#28438,.F.);
#29659=ADVANCED_FACE('',(#4331),#28439,.F.);
#29660=ADVANCED_FACE('',(#4332),#28440,.T.);
#29661=ADVANCED_FACE('',(#4333),#28441,.F.);
#29662=ADVANCED_FACE('',(#4334),#28442,.F.);
#29663=ADVANCED_FACE('',(#4335),#28443,.F.);
#29664=ADVANCED_FACE('',(#4336),#28444,.T.);
#29665=ADVANCED_FACE('',(#4337),#28445,.F.);
#29666=ADVANCED_FACE('',(#4338),#28446,.F.);
#29667=ADVANCED_FACE('',(#4339),#28447,.F.);
#29668=ADVANCED_FACE('',(#4340),#28448,.T.);
#29669=ADVANCED_FACE('',(#4341),#28449,.F.);
#29670=ADVANCED_FACE('',(#4342),#28450,.F.);
#29671=ADVANCED_FACE('',(#4343),#28451,.F.);
#29672=ADVANCED_FACE('',(#4344),#28452,.T.);
#29673=ADVANCED_FACE('',(#4345),#28453,.F.);
#29674=ADVANCED_FACE('',(#4346),#28454,.F.);
#29675=ADVANCED_FACE('',(#4347),#28455,.F.);
#29676=ADVANCED_FACE('',(#4348),#28456,.T.);
#29677=ADVANCED_FACE('',(#4349),#28457,.F.);
#29678=ADVANCED_FACE('',(#4350),#28458,.F.);
#29679=ADVANCED_FACE('',(#4351),#2031,.F.);
#29680=ADVANCED_FACE('',(#4352),#28459,.F.);
#29681=ADVANCED_FACE('',(#4353),#28460,.F.);
#29682=ADVANCED_FACE('',(#4354),#28461,.F.);
#29683=ADVANCED_FACE('',(#4355),#28462,.F.);
#29684=ADVANCED_FACE('',(#4356),#28463,.F.);
#29685=ADVANCED_FACE('',(#4357),#28464,.F.);
#29686=ADVANCED_FACE('',(#4358,#3445),#28465,.F.);
#29687=ADVANCED_FACE('',(#4359),#159,.F.);
#29688=ADVANCED_FACE('',(#4360),#569,.T.);
#29689=ADVANCED_FACE('',(#4361,#3446),#28466,.T.);
#29690=ADVANCED_FACE('',(#4362),#28467,.T.);
#29691=ADVANCED_FACE('',(#4363),#2032,.T.);
#29692=ADVANCED_FACE('',(#4364),#570,.T.);
#29693=ADVANCED_FACE('',(#4365),#2033,.T.);
#29694=ADVANCED_FACE('',(#4366),#571,.T.);
#29695=ADVANCED_FACE('',(#4367,#3447),#28468,.T.);
#29696=ADVANCED_FACE('',(#4368,#3448,#3449,#3450,#3451,#3452,#3453,#3454,
#3455,#3456,#3457,#3458,#3459,#3460,#3461,#3462,#3463,#3464,#3465,#3466,
#3467,#3468,#3469,#3470,#3471,#3472,#3473,#3474,#3475,#3476,#3477,#3478,
#3479,#3480,#3481,#3482),#572,.T.);
#29697=ADVANCED_FACE('',(#4369),#2034,.T.);
#29698=ADVANCED_FACE('',(#4370,#3483),#28469,.T.);
#30666=CLOSED_SHELL('',(#29510,#29511,#29512,#29513,#29514,#29515,#29516,
#29517,#29518,#29519,#29520,#29521,#29522,#29523,#29524,#29525,#29526,#29527,
#29528,#29529,#29530,#29531,#29532,#29533,#29534,#29535,#29536,#29537,#29538,
#29539,#29540,#29541,#29542,#29543,#29544,#29545,#29546,#29547,#29548,#29549,
#29550,#29551,#29552,#29553,#29554,#29555,#29556,#29557,#29558,#29559,#29560,
#29561,#29562,#29563,#29564,#29565,#29566,#29567,#29568,#29569,#29570,#29571,
#29572,#29573,#29574,#29575,#29576,#29577,#29578,#29579,#29580,#29581,#29582,
#29583,#29584,#29585,#29586,#29587,#29588,#29589,#29590,#29591,#29592,#29593,
#29594,#29595,#29596,#29597,#29598,#29599,#29600,#29601,#29602,#29603,#29604,
#29605,#29606,#29607,#29608,#29609,#29610,#29611,#29612,#29613,#29614,#29615,
#29616,#29617,#29618,#29619,#29620,#29621,#29622,#29623,#29624,#29625,#29626,
#29627,#29628,#29629,#29630,#29631,#29632,#29633,#29634,#29635,#29636,#29637,
#29638,#29639,#29640,#29641,#29642,#29643,#29644,#29645,#29646,#29647,#29648,
#29649,#29650,#29651,#29652,#29653,#29654,#29655,#29656,#29657,#29658,#29659,
#29660,#29661,#29662,#29663,#29664,#29665,#29666,#29667,#29668,#29669,#29670,
#29671,#29672,#29673,#29674,#29675,#29676,#29677,#29678,#29679,#29680,#29681,
#29682,#29683,#29684,#29685,#29686,#29687,#29688,#29689,#29690,#29691,#29692,
#29693,#29694,#29695,#29696,#29697,#29698));
#31784=AXIS2_PLACEMENT_3D('',#46413,#35995,#35996);
#31785=AXIS2_PLACEMENT_3D('',#46414,#35997,#35998);
#31786=AXIS2_PLACEMENT_3D('',#46430,#36000,#36001);
#31787=AXIS2_PLACEMENT_3D('',#46438,#36002,#36003);
#31788=AXIS2_PLACEMENT_3D('',#46486,#36005,#36006);
#31789=AXIS2_PLACEMENT_3D('',#46534,#36008,#36009);
#31790=AXIS2_PLACEMENT_3D('',#46582,#36011,#36012);
#31791=AXIS2_PLACEMENT_3D('',#46636,#36014,#36015);
#31792=AXIS2_PLACEMENT_3D('',#46684,#36017,#36018);
#31793=AXIS2_PLACEMENT_3D('',#46732,#36020,#36021);
#31794=AXIS2_PLACEMENT_3D('',#46786,#36023,#36024);
#31795=AXIS2_PLACEMENT_3D('',#46834,#36026,#36027);
#31796=AXIS2_PLACEMENT_3D('',#46882,#36029,#36030);
#31797=AXIS2_PLACEMENT_3D('',#46893,#36032,#36033);
#31798=AXIS2_PLACEMENT_3D('',#46898,#36034,#36035);
#31799=AXIS2_PLACEMENT_3D('',#46922,#36037,#36038);
#31800=AXIS2_PLACEMENT_3D('',#46946,#36040,#36041);
#31801=AXIS2_PLACEMENT_3D('',#46971,#36043,#36044);
#31802=AXIS2_PLACEMENT_3D('',#46996,#36046,#36047);
#31803=AXIS2_PLACEMENT_3D('',#47020,#36049,#36050);
#31804=AXIS2_PLACEMENT_3D('',#47045,#36052,#36053);
#31805=AXIS2_PLACEMENT_3D('',#47070,#36055,#36056);
#31806=AXIS2_PLACEMENT_3D('',#47094,#36058,#36059);
#31807=AXIS2_PLACEMENT_3D('',#47118,#36061,#36062);
#31808=AXIS2_PLACEMENT_3D('',#47218,#36063,#36064);
#31809=AXIS2_PLACEMENT_3D('',#47220,#36065,#36066);
#31810=AXIS2_PLACEMENT_3D('',#47709,#36067,#36068);
#31811=AXIS2_PLACEMENT_3D('',#47711,#36069,#36070);
#31812=AXIS2_PLACEMENT_3D('',#47712,#36071,#36072);
#31813=AXIS2_PLACEMENT_3D('',#47811,#36073,#36074);
#31814=AXIS2_PLACEMENT_3D('',#47812,#36075,#36076);
#31815=AXIS2_PLACEMENT_3D('',#48102,#36077,#36078);
#31816=AXIS2_PLACEMENT_3D('',#48111,#36083,#36084);
#31817=AXIS2_PLACEMENT_3D('',#48113,#36085,#36086);
#31818=AXIS2_PLACEMENT_3D('',#48115,#36088,#36089);
#31819=AXIS2_PLACEMENT_3D('',#48119,#36092,#36093);
#31820=AXIS2_PLACEMENT_3D('',#48120,#36094,#36095);
#31821=AXIS2_PLACEMENT_3D('',#48121,#36096,#36097);
#31822=AXIS2_PLACEMENT_3D('',#48130,#36102,#36103);
#31823=AXIS2_PLACEMENT_3D('',#48132,#36104,#36105);
#31824=AXIS2_PLACEMENT_3D('',#48134,#36107,#36108);
#31825=AXIS2_PLACEMENT_3D('',#48138,#36111,#36112);
#31826=AXIS2_PLACEMENT_3D('',#48139,#36113,#36114);
#31827=AXIS2_PLACEMENT_3D('',#48140,#36115,#36116);
#31828=AXIS2_PLACEMENT_3D('',#48149,#36121,#36122);
#31829=AXIS2_PLACEMENT_3D('',#48151,#36123,#36124);
#31830=AXIS2_PLACEMENT_3D('',#48153,#36126,#36127);
#31831=AXIS2_PLACEMENT_3D('',#48157,#36130,#36131);
#31832=AXIS2_PLACEMENT_3D('',#48158,#36132,#36133);
#31833=AXIS2_PLACEMENT_3D('',#48159,#36134,#36135);
#31834=AXIS2_PLACEMENT_3D('',#48168,#36140,#36141);
#31835=AXIS2_PLACEMENT_3D('',#48170,#36142,#36143);
#31836=AXIS2_PLACEMENT_3D('',#48172,#36145,#36146);
#31837=AXIS2_PLACEMENT_3D('',#48176,#36149,#36150);
#31838=AXIS2_PLACEMENT_3D('',#48177,#36151,#36152);
#31839=AXIS2_PLACEMENT_3D('',#48178,#36153,#36154);
#31840=AXIS2_PLACEMENT_3D('',#48187,#36159,#36160);
#31841=AXIS2_PLACEMENT_3D('',#48189,#36161,#36162);
#31842=AXIS2_PLACEMENT_3D('',#48191,#36164,#36165);
#31843=AXIS2_PLACEMENT_3D('',#48195,#36168,#36169);
#31844=AXIS2_PLACEMENT_3D('',#48196,#36170,#36171);
#31845=AXIS2_PLACEMENT_3D('',#48197,#36172,#36173);
#31846=AXIS2_PLACEMENT_3D('',#48206,#36178,#36179);
#31847=AXIS2_PLACEMENT_3D('',#48208,#36180,#36181);
#31848=AXIS2_PLACEMENT_3D('',#48210,#36183,#36184);
#31849=AXIS2_PLACEMENT_3D('',#48214,#36187,#36188);
#31850=AXIS2_PLACEMENT_3D('',#48215,#36189,#36190);
#31851=AXIS2_PLACEMENT_3D('',#48216,#36191,#36192);
#31852=AXIS2_PLACEMENT_3D('',#48225,#36197,#36198);
#31853=AXIS2_PLACEMENT_3D('',#48227,#36199,#36200);
#31854=AXIS2_PLACEMENT_3D('',#48229,#36202,#36203);
#31855=AXIS2_PLACEMENT_3D('',#48233,#36206,#36207);
#31856=AXIS2_PLACEMENT_3D('',#48234,#36208,#36209);
#31857=AXIS2_PLACEMENT_3D('',#48235,#36210,#36211);
#31858=AXIS2_PLACEMENT_3D('',#48244,#36216,#36217);
#31859=AXIS2_PLACEMENT_3D('',#48246,#36218,#36219);
#31860=AXIS2_PLACEMENT_3D('',#48248,#36221,#36222);
#31861=AXIS2_PLACEMENT_3D('',#48252,#36225,#36226);
#31862=AXIS2_PLACEMENT_3D('',#48253,#36227,#36228);
#31863=AXIS2_PLACEMENT_3D('',#48254,#36229,#36230);
#31864=AXIS2_PLACEMENT_3D('',#48263,#36235,#36236);
#31865=AXIS2_PLACEMENT_3D('',#48265,#36237,#36238);
#31866=AXIS2_PLACEMENT_3D('',#48267,#36240,#36241);
#31867=AXIS2_PLACEMENT_3D('',#48271,#36244,#36245);
#31868=AXIS2_PLACEMENT_3D('',#48272,#36246,#36247);
#31869=AXIS2_PLACEMENT_3D('',#48273,#36248,#36249);
#31870=AXIS2_PLACEMENT_3D('',#48282,#36254,#36255);
#31871=AXIS2_PLACEMENT_3D('',#48284,#36256,#36257);
#31872=AXIS2_PLACEMENT_3D('',#48286,#36259,#36260);
#31873=AXIS2_PLACEMENT_3D('',#48290,#36263,#36264);
#31874=AXIS2_PLACEMENT_3D('',#48291,#36265,#36266);
#31875=AXIS2_PLACEMENT_3D('',#48292,#36267,#36268);
#31876=AXIS2_PLACEMENT_3D('',#48301,#36273,#36274);
#31877=AXIS2_PLACEMENT_3D('',#48303,#36275,#36276);
#31878=AXIS2_PLACEMENT_3D('',#48305,#36278,#36279);
#31879=AXIS2_PLACEMENT_3D('',#48309,#36282,#36283);
#31880=AXIS2_PLACEMENT_3D('',#48310,#36284,#36285);
#31881=AXIS2_PLACEMENT_3D('',#48311,#36286,#36287);
#31882=AXIS2_PLACEMENT_3D('',#48320,#36292,#36293);
#31883=AXIS2_PLACEMENT_3D('',#48322,#36294,#36295);
#31884=AXIS2_PLACEMENT_3D('',#48324,#36297,#36298);
#31885=AXIS2_PLACEMENT_3D('',#48328,#36301,#36302);
#31886=AXIS2_PLACEMENT_3D('',#48329,#36303,#36304);
#31887=AXIS2_PLACEMENT_3D('',#48330,#36305,#36306);
#31888=AXIS2_PLACEMENT_3D('',#48339,#36311,#36312);
#31889=AXIS2_PLACEMENT_3D('',#48341,#36313,#36314);
#31890=AXIS2_PLACEMENT_3D('',#48343,#36316,#36317);
#31891=AXIS2_PLACEMENT_3D('',#48347,#36320,#36321);
#31892=AXIS2_PLACEMENT_3D('',#48348,#36322,#36323);
#31893=AXIS2_PLACEMENT_3D('',#48349,#36324,#36325);
#31894=AXIS2_PLACEMENT_3D('',#48358,#36330,#36331);
#31895=AXIS2_PLACEMENT_3D('',#48360,#36332,#36333);
#31896=AXIS2_PLACEMENT_3D('',#48362,#36335,#36336);
#31897=AXIS2_PLACEMENT_3D('',#48366,#36339,#36340);
#31898=AXIS2_PLACEMENT_3D('',#48367,#36341,#36342);
#31899=AXIS2_PLACEMENT_3D('',#48368,#36343,#36344);
#31900=AXIS2_PLACEMENT_3D('',#48377,#36349,#36350);
#31901=AXIS2_PLACEMENT_3D('',#48379,#36351,#36352);
#31902=AXIS2_PLACEMENT_3D('',#48381,#36354,#36355);
#31903=AXIS2_PLACEMENT_3D('',#48385,#36358,#36359);
#31904=AXIS2_PLACEMENT_3D('',#48386,#36360,#36361);
#31905=AXIS2_PLACEMENT_3D('',#48387,#36362,#36363);
#31906=AXIS2_PLACEMENT_3D('',#48396,#36368,#36369);
#31907=AXIS2_PLACEMENT_3D('',#48398,#36370,#36371);
#31908=AXIS2_PLACEMENT_3D('',#48400,#36373,#36374);
#31909=AXIS2_PLACEMENT_3D('',#48404,#36377,#36378);
#31910=AXIS2_PLACEMENT_3D('',#48405,#36379,#36380);
#31911=AXIS2_PLACEMENT_3D('',#48406,#36381,#36382);
#31912=AXIS2_PLACEMENT_3D('',#48415,#36387,#36388);
#31913=AXIS2_PLACEMENT_3D('',#48417,#36389,#36390);
#31914=AXIS2_PLACEMENT_3D('',#48419,#36392,#36393);
#31915=AXIS2_PLACEMENT_3D('',#48423,#36396,#36397);
#31916=AXIS2_PLACEMENT_3D('',#48424,#36398,#36399);
#31917=AXIS2_PLACEMENT_3D('',#48425,#36400,#36401);
#31918=AXIS2_PLACEMENT_3D('',#48434,#36406,#36407);
#31919=AXIS2_PLACEMENT_3D('',#48436,#36408,#36409);
#31920=AXIS2_PLACEMENT_3D('',#48439,#36411,#36412);
#31921=AXIS2_PLACEMENT_3D('',#48440,#36413,#36414);
#31922=AXIS2_PLACEMENT_3D('',#48444,#36417,#36418);
#31923=AXIS2_PLACEMENT_3D('',#48446,#36419,#36420);
#31924=AXIS2_PLACEMENT_3D('',#48447,#36421,#36422);
#31925=AXIS2_PLACEMENT_3D('',#48448,#36423,#36424);
#31926=AXIS2_PLACEMENT_3D('',#48457,#36429,#36430);
#31927=AXIS2_PLACEMENT_3D('',#48459,#36431,#36432);
#31928=AXIS2_PLACEMENT_3D('',#48461,#36434,#36435);
#31929=AXIS2_PLACEMENT_3D('',#48465,#36438,#36439);
#31930=AXIS2_PLACEMENT_3D('',#48466,#36440,#36441);
#31931=AXIS2_PLACEMENT_3D('',#48467,#36442,#36443);
#31932=AXIS2_PLACEMENT_3D('',#48476,#36448,#36449);
#31933=AXIS2_PLACEMENT_3D('',#48478,#36450,#36451);
#31934=AXIS2_PLACEMENT_3D('',#48480,#36453,#36454);
#31935=AXIS2_PLACEMENT_3D('',#48484,#36457,#36458);
#31936=AXIS2_PLACEMENT_3D('',#48485,#36459,#36460);
#31937=AXIS2_PLACEMENT_3D('',#48486,#36461,#36462);
#31938=AXIS2_PLACEMENT_3D('',#48495,#36467,#36468);
#31939=AXIS2_PLACEMENT_3D('',#48497,#36469,#36470);
#31940=AXIS2_PLACEMENT_3D('',#48499,#36472,#36473);
#31941=AXIS2_PLACEMENT_3D('',#48503,#36476,#36477);
#31942=AXIS2_PLACEMENT_3D('',#48504,#36478,#36479);
#31943=AXIS2_PLACEMENT_3D('',#48505,#36480,#36481);
#31944=AXIS2_PLACEMENT_3D('',#48514,#36486,#36487);
#31945=AXIS2_PLACEMENT_3D('',#48516,#36488,#36489);
#31946=AXIS2_PLACEMENT_3D('',#48518,#36491,#36492);
#31947=AXIS2_PLACEMENT_3D('',#48522,#36495,#36496);
#31948=AXIS2_PLACEMENT_3D('',#48523,#36497,#36498);
#31949=AXIS2_PLACEMENT_3D('',#48524,#36499,#36500);
#31950=AXIS2_PLACEMENT_3D('',#48533,#36505,#36506);
#31951=AXIS2_PLACEMENT_3D('',#48535,#36507,#36508);
#31952=AXIS2_PLACEMENT_3D('',#48537,#36510,#36511);
#31953=AXIS2_PLACEMENT_3D('',#48541,#36514,#36515);
#31954=AXIS2_PLACEMENT_3D('',#48542,#36516,#36517);
#31955=AXIS2_PLACEMENT_3D('',#48543,#36518,#36519);
#31956=AXIS2_PLACEMENT_3D('',#48552,#36524,#36525);
#31957=AXIS2_PLACEMENT_3D('',#48554,#36526,#36527);
#31958=AXIS2_PLACEMENT_3D('',#48556,#36529,#36530);
#31959=AXIS2_PLACEMENT_3D('',#48560,#36533,#36534);
#31960=AXIS2_PLACEMENT_3D('',#48561,#36535,#36536);
#31961=AXIS2_PLACEMENT_3D('',#48562,#36537,#36538);
#31962=AXIS2_PLACEMENT_3D('',#48571,#36543,#36544);
#31963=AXIS2_PLACEMENT_3D('',#48573,#36545,#36546);
#31964=AXIS2_PLACEMENT_3D('',#48575,#36548,#36549);
#31965=AXIS2_PLACEMENT_3D('',#48579,#36552,#36553);
#31966=AXIS2_PLACEMENT_3D('',#48580,#36554,#36555);
#31967=AXIS2_PLACEMENT_3D('',#48581,#36556,#36557);
#31968=AXIS2_PLACEMENT_3D('',#48590,#36562,#36563);
#31969=AXIS2_PLACEMENT_3D('',#48592,#36564,#36565);
#31970=AXIS2_PLACEMENT_3D('',#48594,#36567,#36568);
#31971=AXIS2_PLACEMENT_3D('',#48598,#36571,#36572);
#31972=AXIS2_PLACEMENT_3D('',#48599,#36573,#36574);
#31973=AXIS2_PLACEMENT_3D('',#48600,#36575,#36576);
#31974=AXIS2_PLACEMENT_3D('',#48609,#36581,#36582);
#31975=AXIS2_PLACEMENT_3D('',#48611,#36583,#36584);
#31976=AXIS2_PLACEMENT_3D('',#48613,#36586,#36587);
#31977=AXIS2_PLACEMENT_3D('',#48617,#36590,#36591);
#31978=AXIS2_PLACEMENT_3D('',#48618,#36592,#36593);
#31979=AXIS2_PLACEMENT_3D('',#48619,#36594,#36595);
#31980=AXIS2_PLACEMENT_3D('',#48628,#36600,#36601);
#31981=AXIS2_PLACEMENT_3D('',#48630,#36602,#36603);
#31982=AXIS2_PLACEMENT_3D('',#48632,#36605,#36606);
#31983=AXIS2_PLACEMENT_3D('',#48636,#36609,#36610);
#31984=AXIS2_PLACEMENT_3D('',#48637,#36611,#36612);
#31985=AXIS2_PLACEMENT_3D('',#48638,#36613,#36614);
#31986=AXIS2_PLACEMENT_3D('',#48647,#36619,#36620);
#31987=AXIS2_PLACEMENT_3D('',#48649,#36621,#36622);
#31988=AXIS2_PLACEMENT_3D('',#48651,#36624,#36625);
#31989=AXIS2_PLACEMENT_3D('',#48655,#36628,#36629);
#31990=AXIS2_PLACEMENT_3D('',#48656,#36630,#36631);
#31991=AXIS2_PLACEMENT_3D('',#48657,#36632,#36633);
#31992=AXIS2_PLACEMENT_3D('',#48666,#36638,#36639);
#31993=AXIS2_PLACEMENT_3D('',#48668,#36640,#36641);
#31994=AXIS2_PLACEMENT_3D('',#48670,#36643,#36644);
#31995=AXIS2_PLACEMENT_3D('',#48674,#36647,#36648);
#31996=AXIS2_PLACEMENT_3D('',#48675,#36649,#36650);
#31997=AXIS2_PLACEMENT_3D('',#48676,#36651,#36652);
#31998=AXIS2_PLACEMENT_3D('',#48685,#36657,#36658);
#31999=AXIS2_PLACEMENT_3D('',#48687,#36659,#36660);
#32000=AXIS2_PLACEMENT_3D('',#48689,#36662,#36663);
#32001=AXIS2_PLACEMENT_3D('',#48693,#36666,#36667);
#32002=AXIS2_PLACEMENT_3D('',#48694,#36668,#36669);
#32003=AXIS2_PLACEMENT_3D('',#48695,#36670,#36671);
#32004=AXIS2_PLACEMENT_3D('',#48704,#36676,#36677);
#32005=AXIS2_PLACEMENT_3D('',#48706,#36678,#36679);
#32006=AXIS2_PLACEMENT_3D('',#48708,#36681,#36682);
#32007=AXIS2_PLACEMENT_3D('',#48712,#36685,#36686);
#32008=AXIS2_PLACEMENT_3D('',#48713,#36687,#36688);
#32009=AXIS2_PLACEMENT_3D('',#48714,#36689,#36690);
#32010=AXIS2_PLACEMENT_3D('',#48723,#36695,#36696);
#32011=AXIS2_PLACEMENT_3D('',#48725,#36697,#36698);
#32012=AXIS2_PLACEMENT_3D('',#48727,#36700,#36701);
#32013=AXIS2_PLACEMENT_3D('',#48731,#36704,#36705);
#32014=AXIS2_PLACEMENT_3D('',#48732,#36706,#36707);
#32015=AXIS2_PLACEMENT_3D('',#48733,#36708,#36709);
#32016=AXIS2_PLACEMENT_3D('',#48742,#36714,#36715);
#32017=AXIS2_PLACEMENT_3D('',#48744,#36716,#36717);
#32018=AXIS2_PLACEMENT_3D('',#48746,#36719,#36720);
#32019=AXIS2_PLACEMENT_3D('',#48750,#36723,#36724);
#32020=AXIS2_PLACEMENT_3D('',#48751,#36725,#36726);
#32021=AXIS2_PLACEMENT_3D('',#48752,#36727,#36728);
#32022=AXIS2_PLACEMENT_3D('',#48761,#36733,#36734);
#32023=AXIS2_PLACEMENT_3D('',#48763,#36735,#36736);
#32024=AXIS2_PLACEMENT_3D('',#48765,#36738,#36739);
#32025=AXIS2_PLACEMENT_3D('',#48769,#36742,#36743);
#32026=AXIS2_PLACEMENT_3D('',#48770,#36744,#36745);
#32027=AXIS2_PLACEMENT_3D('',#48771,#36746,#36747);
#32028=AXIS2_PLACEMENT_3D('',#48780,#36752,#36753);
#32029=AXIS2_PLACEMENT_3D('',#48782,#36754,#36755);
#32030=AXIS2_PLACEMENT_3D('',#48784,#36757,#36758);
#32031=AXIS2_PLACEMENT_3D('',#48788,#36761,#36762);
#32032=AXIS2_PLACEMENT_3D('',#48789,#36763,#36764);
#32033=AXIS2_PLACEMENT_3D('',#48790,#36765,#36766);
#32034=AXIS2_PLACEMENT_3D('',#48794,#36768,#36769);
#32035=AXIS2_PLACEMENT_3D('',#48795,#36770,#36771);
#32036=AXIS2_PLACEMENT_3D('',#48804,#36776,#36777);
#32037=AXIS2_PLACEMENT_3D('',#48810,#36781,#36782);
#32038=AXIS2_PLACEMENT_3D('',#48816,#36786,#36787);
#32039=AXIS2_PLACEMENT_3D('',#48822,#36791,#36792);
#32040=AXIS2_PLACEMENT_3D('',#48828,#36796,#36797);
#32041=AXIS2_PLACEMENT_3D('',#48831,#36800,#36801);
#32042=AXIS2_PLACEMENT_3D('',#48832,#36802,#36803);
#32043=AXIS2_PLACEMENT_3D('',#48835,#36804,#36805);
#32044=AXIS2_PLACEMENT_3D('',#48837,#36806,#36807);
#32045=AXIS2_PLACEMENT_3D('',#48838,#36808,#36809);
#32046=AXIS2_PLACEMENT_3D('',#48839,#36810,#36811);
#32047=AXIS2_PLACEMENT_3D('',#48840,#36812,#36813);
#32048=AXIS2_PLACEMENT_3D('',#48843,#36815,#36816);
#32049=AXIS2_PLACEMENT_3D('',#48844,#36817,#36818);
#32050=AXIS2_PLACEMENT_3D('',#48846,#36819,#36820);
#32051=AXIS2_PLACEMENT_3D('',#48847,#36821,#36822);
#32052=AXIS2_PLACEMENT_3D('',#48849,#36823,#36824);
#32053=AXIS2_PLACEMENT_3D('',#48850,#36825,#36826);
#32054=AXIS2_PLACEMENT_3D('',#48852,#36828,#36829);
#32055=AXIS2_PLACEMENT_3D('',#48853,#36830,#36831);
#32056=AXIS2_PLACEMENT_3D('',#48854,#36832,#36833);
#32057=AXIS2_PLACEMENT_3D('',#48856,#36834,#36835);
#32058=AXIS2_PLACEMENT_3D('',#48858,#36837,#36838);
#32059=AXIS2_PLACEMENT_3D('',#48860,#36839,#36840);
#32060=AXIS2_PLACEMENT_3D('',#48862,#36842,#36843);
#32061=AXIS2_PLACEMENT_3D('',#48863,#36844,#36845);
#32062=AXIS2_PLACEMENT_3D('',#48865,#36846,#36847);
#32063=AXIS2_PLACEMENT_3D('',#48868,#36850,#36851);
#32064=AXIS2_PLACEMENT_3D('',#48870,#36852,#36853);
#32065=AXIS2_PLACEMENT_3D('',#48872,#36855,#36856);
#35995=DIRECTION('axis',(0.,0.,1.));
#35996=DIRECTION('refdir',(1.,0.,0.));
#35997=DIRECTION('center_axis',(1.,0.,0.));
#35998=DIRECTION('ref_axis',(0.,1.,0.));
#35999=DIRECTION('',(-1.,0.,0.));
#36000=DIRECTION('center_axis',(1.,0.,0.));
#36001=DIRECTION('ref_axis',(0.,1.,0.));
#36002=DIRECTION('center_axis',(1.,0.,0.));
#36003=DIRECTION('ref_axis',(0.,1.,0.));
#36004=DIRECTION('',(-1.,0.,0.));
#36005=DIRECTION('center_axis',(1.,0.,0.));
#36006=DIRECTION('ref_axis',(0.,1.,0.));
#36007=DIRECTION('',(-1.,0.,0.));
#36008=DIRECTION('center_axis',(1.,0.,0.));
#36009=DIRECTION('ref_axis',(0.,1.,0.));
#36010=DIRECTION('',(-1.,0.,0.));
#36011=DIRECTION('center_axis',(1.,0.,0.));
#36012=DIRECTION('ref_axis',(0.,1.,0.));
#36013=DIRECTION('',(-1.,0.,0.));
#36014=DIRECTION('center_axis',(1.,0.,0.));
#36015=DIRECTION('ref_axis',(0.,1.,0.));
#36016=DIRECTION('',(-1.,0.,0.));
#36017=DIRECTION('center_axis',(1.,0.,0.));
#36018=DIRECTION('ref_axis',(0.,1.,0.));
#36019=DIRECTION('',(-1.,0.,0.));
#36020=DIRECTION('center_axis',(1.,0.,0.));
#36021=DIRECTION('ref_axis',(0.,1.,0.));
#36022=DIRECTION('',(-1.,0.,0.));
#36023=DIRECTION('center_axis',(1.,0.,0.));
#36024=DIRECTION('ref_axis',(0.,1.,0.));
#36025=DIRECTION('',(-1.,0.,0.));
#36026=DIRECTION('center_axis',(1.,0.,0.));
#36027=DIRECTION('ref_axis',(0.,1.,0.));
#36028=DIRECTION('',(-1.,0.,0.));
#36029=DIRECTION('center_axis',(1.,0.,0.));
#36030=DIRECTION('ref_axis',(0.,1.,5.66627894982857E-14));
#36031=DIRECTION('',(1.,0.,0.));
#36032=DIRECTION('center_axis',(1.,0.,0.));
#36033=DIRECTION('ref_axis',(0.,1.,5.66627894982857E-14));
#36034=DIRECTION('center_axis',(1.,0.,0.));
#36035=DIRECTION('ref_axis',(0.,1.,5.66627894982857E-14));
#36036=DIRECTION('',(1.,0.,0.));
#36037=DIRECTION('center_axis',(1.,0.,0.));
#36038=DIRECTION('ref_axis',(0.,1.,5.66627894982857E-14));
#36039=DIRECTION('',(1.,0.,0.));
#36040=DIRECTION('center_axis',(1.,0.,0.));
#36041=DIRECTION('ref_axis',(0.,1.,5.66627894982857E-14));
#36042=DIRECTION('',(1.,0.,0.));
#36043=DIRECTION('center_axis',(1.,0.,0.));
#36044=DIRECTION('ref_axis',(0.,1.,5.66627894982857E-14));
#36045=DIRECTION('',(1.,0.,0.));
#36046=DIRECTION('center_axis',(1.,0.,0.));
#36047=DIRECTION('ref_axis',(0.,1.,5.66627894982857E-14));
#36048=DIRECTION('',(1.,0.,0.));
#36049=DIRECTION('center_axis',(1.,0.,0.));
#36050=DIRECTION('ref_axis',(0.,1.,5.66627894982857E-14));
#36051=DIRECTION('',(1.,0.,0.));
#36052=DIRECTION('center_axis',(1.,0.,0.));
#36053=DIRECTION('ref_axis',(0.,1.,5.66627894982857E-14));
#36054=DIRECTION('',(1.,0.,0.));
#36055=DIRECTION('center_axis',(1.,0.,0.));
#36056=DIRECTION('ref_axis',(0.,1.,5.66627894982857E-14));
#36057=DIRECTION('',(1.,0.,0.));
#36058=DIRECTION('center_axis',(1.,0.,0.));
#36059=DIRECTION('ref_axis',(0.,1.,5.66627894982857E-14));
#36060=DIRECTION('',(1.,0.,0.));
#36061=DIRECTION('center_axis',(1.,0.,0.));
#36062=DIRECTION('ref_axis',(0.,0.,-1.));
#36063=DIRECTION('center_axis',(-1.,0.,0.));
#36064=DIRECTION('ref_axis',(0.,1.,0.));
#36065=DIRECTION('center_axis',(-1.,0.,0.));
#36066=DIRECTION('ref_axis',(0.,1.,0.));
#36067=DIRECTION('center_axis',(1.,0.,0.));
#36068=DIRECTION('ref_axis',(0.,0.,-1.));
#36069=DIRECTION('center_axis',(1.,0.,0.));
#36070=DIRECTION('ref_axis',(0.,1.,0.));
#36071=DIRECTION('center_axis',(1.,0.,0.));
#36072=DIRECTION('ref_axis',(0.,1.,0.));
#36073=DIRECTION('center_axis',(-1.,0.,0.));
#36074=DIRECTION('ref_axis',(0.,1.,5.66627894982857E-14));
#36075=DIRECTION('center_axis',(1.,0.,0.));
#36076=DIRECTION('ref_axis',(0.,1.,5.66627894982857E-14));
#36077=DIRECTION('center_axis',(0.,-0.479608080343199,0.877482814230291));
#36078=DIRECTION('ref_axis',(0.,-0.877482814230291,-0.479608080343199));
#36079=DIRECTION('',(-1.,0.,0.));
#36080=DIRECTION('',(0.,-0.877482814230291,-0.479608080343199));
#36081=DIRECTION('',(1.,0.,0.));
#36082=DIRECTION('',(0.,-0.877482814230291,-0.479608080343199));
#36083=DIRECTION('center_axis',(1.,0.,0.));
#36084=DIRECTION('ref_axis',(0.,-0.17364817766693,-0.984807753012208));
#36085=DIRECTION('center_axis',(-1.,0.,0.));
#36086=DIRECTION('ref_axis',(0.,1.,0.));
#36087=DIRECTION('',(0.,0.660528501019527,-0.750800971856654));
#36088=DIRECTION('center_axis',(0.,-0.750800971856655,-0.660528501019527));
#36089=DIRECTION('ref_axis',(0.,0.660528501019527,-0.750800971856654));
#36090=DIRECTION('',(1.,0.,0.));
#36091=DIRECTION('',(0.,0.660528501019527,-0.750800971856654));
#36092=DIRECTION('center_axis',(1.,0.,0.));
#36093=DIRECTION('ref_axis',(0.,-0.17364817766693,-0.984807753012208));
#36094=DIRECTION('center_axis',(1.,0.,0.));
#36095=DIRECTION('ref_axis',(0.,1.,0.));
#36096=DIRECTION('center_axis',(0.,-0.319948464304144,0.947434947734893));
#36097=DIRECTION('ref_axis',(0.,-0.947434947734893,-0.319948464304144));
#36098=DIRECTION('',(-1.,0.,0.));
#36099=DIRECTION('',(0.,-0.947434947734893,-0.319948464304144));
#36100=DIRECTION('',(1.,0.,0.));
#36101=DIRECTION('',(0.,-0.947434947734893,-0.319948464304144));
#36102=DIRECTION('center_axis',(1.,0.,0.));
#36103=DIRECTION('ref_axis',(0.,-0.342020143325669,-0.939692620785908));
#36104=DIRECTION('center_axis',(-1.,0.,0.));
#36105=DIRECTION('ref_axis',(0.,1.,0.));
#36106=DIRECTION('',(0.,0.520118368336093,-0.854094188552644));
#36107=DIRECTION('center_axis',(0.,-0.854094188552644,-0.520118368336093));
#36108=DIRECTION('ref_axis',(0.,0.520118368336093,-0.854094188552644));
#36109=DIRECTION('',(1.,0.,0.));
#36110=DIRECTION('',(0.,0.520118368336093,-0.854094188552644));
#36111=DIRECTION('center_axis',(1.,0.,0.));
#36112=DIRECTION('ref_axis',(0.,-0.342020143325669,-0.939692620785908));
#36113=DIRECTION('center_axis',(1.,0.,0.));
#36114=DIRECTION('ref_axis',(0.,1.,0.));
#36115=DIRECTION('center_axis',(0.,-0.150567376078943,0.988599749777787));
#36116=DIRECTION('ref_axis',(0.,-0.988599749777787,-0.150567376078943));
#36117=DIRECTION('',(-1.,0.,0.));
#36118=DIRECTION('',(0.,-0.988599749777787,-0.150567376078943));
#36119=DIRECTION('',(1.,0.,0.));
#36120=DIRECTION('',(0.,-0.988599749777787,-0.150567376078943));
#36121=DIRECTION('center_axis',(1.,0.,0.));
#36122=DIRECTION('ref_axis',(0.,-0.5,-0.866025403784438));
#36123=DIRECTION('center_axis',(-1.,0.,0.));
#36124=DIRECTION('ref_axis',(0.,1.,0.));
#36125=DIRECTION('',(0.,0.363904702223362,-0.931436185521974));
#36126=DIRECTION('center_axis',(0.,-0.931436185521975,-0.363904702223362));
#36127=DIRECTION('ref_axis',(0.,0.363904702223362,-0.931436185521975));
#36128=DIRECTION('',(1.,0.,0.));
#36129=DIRECTION('',(0.,0.363904702223362,-0.931436185521974));
#36130=DIRECTION('center_axis',(1.,0.,0.));
#36131=DIRECTION('ref_axis',(0.,-0.5,-0.866025403784438));
#36132=DIRECTION('center_axis',(1.,0.,0.));
#36133=DIRECTION('ref_axis',(0.,1.,0.));
#36134=DIRECTION('center_axis',(0.,0.0233886256776475,0.999726448679293));
#36135=DIRECTION('ref_axis',(0.,-0.999726448679293,0.0233886256776475));
#36136=DIRECTION('',(-1.,0.,0.));
#36137=DIRECTION('',(0.,-0.999726448679293,0.0233886256776475));
#36138=DIRECTION('',(1.,0.,0.));
#36139=DIRECTION('',(0.,-0.999726448679293,0.0233886256776475));
#36140=DIRECTION('center_axis',(1.,0.,0.));
#36141=DIRECTION('ref_axis',(0.,-0.64278760968654,-0.766044443118978));
#36142=DIRECTION('center_axis',(-1.,0.,0.));
#36143=DIRECTION('ref_axis',(0.,1.,0.));
#36144=DIRECTION('',(0.,0.196633975878238,-0.980476965323672));
#36145=DIRECTION('center_axis',(0.,-0.980476965323672,-0.196633975878238));
#36146=DIRECTION('ref_axis',(0.,0.196633975878238,-0.980476965323672));
#36147=DIRECTION('',(1.,0.,0.));
#36148=DIRECTION('',(0.,0.196633975878238,-0.980476965323672));
#36149=DIRECTION('center_axis',(1.,0.,0.));
#36150=DIRECTION('ref_axis',(0.,-0.64278760968654,-0.766044443118978));
#36151=DIRECTION('center_axis',(1.,0.,0.));
#36152=DIRECTION('ref_axis',(0.,1.,0.));
#36153=DIRECTION('center_axis',(0.,0.196633975878239,0.980476965323672));
#36154=DIRECTION('ref_axis',(0.,-0.980476965323671,0.196633975878239));
#36155=DIRECTION('',(-1.,0.,0.));
#36156=DIRECTION('',(0.,-0.980476965323671,0.196633975878239));
#36157=DIRECTION('',(1.,0.,0.));
#36158=DIRECTION('',(0.,-0.980476965323671,0.196633975878239));
#36159=DIRECTION('center_axis',(1.,0.,0.));
#36160=DIRECTION('ref_axis',(0.,-0.766044443118978,-0.642787609686539));
#36161=DIRECTION('center_axis',(-1.,0.,0.));
#36162=DIRECTION('ref_axis',(0.,1.,0.));
#36163=DIRECTION('',(0.,0.0233886256776471,-0.999726448679293));
#36164=DIRECTION('center_axis',(0.,-0.999726448679293,-0.0233886256776472));
#36165=DIRECTION('ref_axis',(0.,0.0233886256776472,-0.999726448679293));
#36166=DIRECTION('',(1.,0.,0.));
#36167=DIRECTION('',(0.,0.0233886256776471,-0.999726448679293));
#36168=DIRECTION('center_axis',(1.,0.,0.));
#36169=DIRECTION('ref_axis',(0.,-0.766044443118978,-0.642787609686539));
#36170=DIRECTION('center_axis',(1.,0.,0.));
#36171=DIRECTION('ref_axis',(0.,1.,0.));
#36172=DIRECTION('center_axis',(0.,0.363904702223362,0.931436185521974));
#36173=DIRECTION('ref_axis',(0.,-0.931436185521974,0.363904702223362));
#36174=DIRECTION('',(-1.,0.,0.));
#36175=DIRECTION('',(0.,-0.931436185521974,0.363904702223362));
#36176=DIRECTION('',(1.,0.,0.));
#36177=DIRECTION('',(0.,-0.931436185521974,0.363904702223362));
#36178=DIRECTION('center_axis',(1.,0.,0.));
#36179=DIRECTION('ref_axis',(0.,-0.866025403784439,-0.5));
#36180=DIRECTION('center_axis',(-1.,0.,0.));
#36181=DIRECTION('ref_axis',(0.,1.,0.));
#36182=DIRECTION('',(0.,-0.150567376078944,-0.988599749777787));
#36183=DIRECTION('center_axis',(0.,-0.988599749777787,0.150567376078944));
#36184=DIRECTION('ref_axis',(0.,-0.150567376078944,-0.988599749777787));
#36185=DIRECTION('',(1.,0.,0.));
#36186=DIRECTION('',(0.,-0.150567376078944,-0.988599749777787));
#36187=DIRECTION('center_axis',(1.,0.,0.));
#36188=DIRECTION('ref_axis',(0.,-0.866025403784439,-0.5));
#36189=DIRECTION('center_axis',(1.,0.,0.));
#36190=DIRECTION('ref_axis',(0.,1.,0.));
#36191=DIRECTION('center_axis',(0.,0.520118368336095,0.854094188552644));
#36192=DIRECTION('ref_axis',(0.,-0.854094188552644,0.520118368336094));
#36193=DIRECTION('',(-1.,0.,0.));
#36194=DIRECTION('',(0.,-0.854094188552644,0.520118368336095));
#36195=DIRECTION('',(1.,0.,0.));
#36196=DIRECTION('',(0.,-0.854094188552644,0.520118368336095));
#36197=DIRECTION('center_axis',(1.,0.,0.));
#36198=DIRECTION('ref_axis',(0.,-0.939692620785909,-0.342020143325668));
#36199=DIRECTION('center_axis',(-1.,0.,0.));
#36200=DIRECTION('ref_axis',(0.,1.,0.));
#36201=DIRECTION('',(0.,-0.319948464304145,-0.947434947734893));
#36202=DIRECTION('center_axis',(0.,-0.947434947734893,0.319948464304145));
#36203=DIRECTION('ref_axis',(0.,-0.319948464304145,-0.947434947734893));
#36204=DIRECTION('',(1.,0.,0.));
#36205=DIRECTION('',(0.,-0.319948464304145,-0.947434947734893));
#36206=DIRECTION('center_axis',(1.,0.,0.));
#36207=DIRECTION('ref_axis',(0.,-0.939692620785909,-0.342020143325668));
#36208=DIRECTION('center_axis',(1.,0.,0.));
#36209=DIRECTION('ref_axis',(0.,1.,0.));
#36210=DIRECTION('center_axis',(0.,0.660528501019527,0.750800971856654));
#36211=DIRECTION('ref_axis',(0.,-0.750800971856654,0.660528501019527));
#36212=DIRECTION('',(-1.,0.,0.));
#36213=DIRECTION('',(0.,-0.750800971856654,0.660528501019527));
#36214=DIRECTION('',(1.,0.,0.));
#36215=DIRECTION('',(0.,-0.750800971856654,0.660528501019527));
#36216=DIRECTION('center_axis',(1.,0.,0.));
#36217=DIRECTION('ref_axis',(0.,-0.984807753012208,-0.17364817766693));
#36218=DIRECTION('center_axis',(-1.,0.,0.));
#36219=DIRECTION('ref_axis',(0.,1.,0.));
#36220=DIRECTION('',(0.,-0.479608080343199,-0.877482814230291));
#36221=DIRECTION('center_axis',(0.,-0.877482814230291,0.479608080343199));
#36222=DIRECTION('ref_axis',(0.,-0.479608080343199,-0.877482814230291));
#36223=DIRECTION('',(1.,0.,0.));
#36224=DIRECTION('',(0.,-0.479608080343199,-0.877482814230291));
#36225=DIRECTION('center_axis',(1.,0.,0.));
#36226=DIRECTION('ref_axis',(0.,-0.984807753012208,-0.17364817766693));
#36227=DIRECTION('center_axis',(1.,0.,0.));
#36228=DIRECTION('ref_axis',(0.,1.,0.));
#36229=DIRECTION('center_axis',(0.,0.780868809443031,0.624695047554424));
#36230=DIRECTION('ref_axis',(0.,-0.624695047554424,0.780868809443031));
#36231=DIRECTION('',(-1.,0.,0.));
#36232=DIRECTION('',(0.,-0.624695047554424,0.780868809443031));
#36233=DIRECTION('',(1.,0.,0.));
#36234=DIRECTION('',(0.,-0.624695047554424,0.780868809443031));
#36235=DIRECTION('center_axis',(1.,0.,0.));
#36236=DIRECTION('ref_axis',(0.,-1.,1.83697019872103E-16));
#36237=DIRECTION('center_axis',(-1.,0.,0.));
#36238=DIRECTION('ref_axis',(0.,1.,0.));
#36239=DIRECTION('',(0.,-0.624695047554424,-0.78086880944303));
#36240=DIRECTION('center_axis',(0.,-0.78086880944303,0.624695047554424));
#36241=DIRECTION('ref_axis',(0.,-0.624695047554424,-0.78086880944303));
#36242=DIRECTION('',(1.,0.,0.));
#36243=DIRECTION('',(0.,-0.624695047554424,-0.78086880944303));
#36244=DIRECTION('center_axis',(1.,0.,0.));
#36245=DIRECTION('ref_axis',(0.,-1.,1.83697019872103E-16));
#36246=DIRECTION('center_axis',(1.,0.,0.));
#36247=DIRECTION('ref_axis',(0.,1.,0.));
#36248=DIRECTION('center_axis',(0.,0.877482814230291,0.479608080343199));
#36249=DIRECTION('ref_axis',(0.,-0.479608080343199,0.877482814230291));
#36250=DIRECTION('',(-1.,0.,0.));
#36251=DIRECTION('',(0.,-0.479608080343199,0.877482814230291));
#36252=DIRECTION('',(1.,0.,0.));
#36253=DIRECTION('',(0.,-0.479608080343199,0.877482814230291));
#36254=DIRECTION('center_axis',(1.,0.,0.));
#36255=DIRECTION('ref_axis',(0.,-0.984807753012208,0.17364817766693));
#36256=DIRECTION('center_axis',(-1.,0.,0.));
#36257=DIRECTION('ref_axis',(0.,1.,0.));
#36258=DIRECTION('',(0.,-0.750800971856654,-0.660528501019527));
#36259=DIRECTION('center_axis',(0.,-0.660528501019527,0.750800971856655));
#36260=DIRECTION('ref_axis',(0.,-0.750800971856654,-0.660528501019527));
#36261=DIRECTION('',(1.,0.,0.));
#36262=DIRECTION('',(0.,-0.750800971856654,-0.660528501019527));
#36263=DIRECTION('center_axis',(1.,0.,0.));
#36264=DIRECTION('ref_axis',(0.,-0.984807753012208,0.17364817766693));
#36265=DIRECTION('center_axis',(1.,0.,0.));
#36266=DIRECTION('ref_axis',(0.,1.,0.));
#36267=DIRECTION('center_axis',(0.,0.947434947734893,0.319948464304144));
#36268=DIRECTION('ref_axis',(0.,-0.319948464304144,0.947434947734893));
#36269=DIRECTION('',(-1.,0.,0.));
#36270=DIRECTION('',(0.,-0.319948464304144,0.947434947734893));
#36271=DIRECTION('',(1.,0.,0.));
#36272=DIRECTION('',(0.,-0.319948464304144,0.947434947734893));
#36273=DIRECTION('center_axis',(1.,0.,0.));
#36274=DIRECTION('ref_axis',(0.,-0.939692620785908,0.342020143325669));
#36275=DIRECTION('center_axis',(-1.,0.,0.));
#36276=DIRECTION('ref_axis',(0.,1.,0.));
#36277=DIRECTION('',(0.,-0.854094188552644,-0.520118368336093));
#36278=DIRECTION('center_axis',(0.,-0.520118368336093,0.854094188552644));
#36279=DIRECTION('ref_axis',(0.,-0.854094188552644,-0.520118368336093));
#36280=DIRECTION('',(1.,0.,0.));
#36281=DIRECTION('',(0.,-0.854094188552644,-0.520118368336093));
#36282=DIRECTION('center_axis',(1.,0.,0.));
#36283=DIRECTION('ref_axis',(0.,-0.939692620785908,0.342020143325669));
#36284=DIRECTION('center_axis',(1.,0.,0.));
#36285=DIRECTION('ref_axis',(0.,1.,0.));
#36286=DIRECTION('center_axis',(0.,0.988599749777787,0.150567376078943));
#36287=DIRECTION('ref_axis',(0.,-0.150567376078943,0.988599749777787));
#36288=DIRECTION('',(-1.,0.,0.));
#36289=DIRECTION('',(0.,-0.150567376078943,0.988599749777787));
#36290=DIRECTION('',(1.,0.,0.));
#36291=DIRECTION('',(0.,-0.150567376078943,0.988599749777787));
#36292=DIRECTION('center_axis',(1.,0.,0.));
#36293=DIRECTION('ref_axis',(0.,-0.866025403784438,0.5));
#36294=DIRECTION('center_axis',(-1.,0.,0.));
#36295=DIRECTION('ref_axis',(0.,1.,0.));
#36296=DIRECTION('',(0.,-0.931436185521974,-0.363904702223362));
#36297=DIRECTION('center_axis',(0.,-0.363904702223362,0.931436185521975));
#36298=DIRECTION('ref_axis',(0.,-0.931436185521975,-0.363904702223362));
#36299=DIRECTION('',(1.,0.,0.));
#36300=DIRECTION('',(0.,-0.931436185521974,-0.363904702223362));
#36301=DIRECTION('center_axis',(1.,0.,0.));
#36302=DIRECTION('ref_axis',(0.,-0.866025403784438,0.5));
#36303=DIRECTION('center_axis',(1.,0.,0.));
#36304=DIRECTION('ref_axis',(0.,1.,0.));
#36305=DIRECTION('center_axis',(0.,0.999726448679293,-0.0233886256776474));
#36306=DIRECTION('ref_axis',(0.,0.0233886256776474,0.999726448679293));
#36307=DIRECTION('',(-1.,0.,0.));
#36308=DIRECTION('',(0.,0.0233886256776475,0.999726448679293));
#36309=DIRECTION('',(1.,0.,0.));
#36310=DIRECTION('',(0.,0.0233886256776475,0.999726448679293));
#36311=DIRECTION('center_axis',(1.,0.,0.));
#36312=DIRECTION('ref_axis',(0.,-0.766044443118978,0.642787609686539));
#36313=DIRECTION('center_axis',(-1.,0.,0.));
#36314=DIRECTION('ref_axis',(0.,1.,0.));
#36315=DIRECTION('',(0.,-0.980476965323672,-0.196633975878238));
#36316=DIRECTION('center_axis',(0.,-0.196633975878238,0.980476965323672));
#36317=DIRECTION('ref_axis',(0.,-0.980476965323672,-0.196633975878238));
#36318=DIRECTION('',(1.,0.,0.));
#36319=DIRECTION('',(0.,-0.980476965323672,-0.196633975878238));
#36320=DIRECTION('center_axis',(1.,0.,0.));
#36321=DIRECTION('ref_axis',(0.,-0.766044443118978,0.642787609686539));
#36322=DIRECTION('center_axis',(1.,0.,0.));
#36323=DIRECTION('ref_axis',(0.,1.,0.));
#36324=DIRECTION('center_axis',(0.,0.980476965323672,-0.196633975878239));
#36325=DIRECTION('ref_axis',(0.,0.196633975878239,0.980476965323671));
#36326=DIRECTION('',(-1.,0.,0.));
#36327=DIRECTION('',(0.,0.196633975878239,0.980476965323671));
#36328=DIRECTION('',(1.,0.,0.));
#36329=DIRECTION('',(0.,0.196633975878239,0.980476965323671));
#36330=DIRECTION('center_axis',(1.,0.,0.));
#36331=DIRECTION('ref_axis',(0.,-0.642787609686539,0.766044443118978));
#36332=DIRECTION('center_axis',(-1.,0.,0.));
#36333=DIRECTION('ref_axis',(0.,1.,0.));
#36334=DIRECTION('',(0.,-0.999726448679293,-0.0233886256776472));
#36335=DIRECTION('center_axis',(0.,-0.0233886256776472,0.999726448679293));
#36336=DIRECTION('ref_axis',(0.,-0.999726448679293,-0.0233886256776472));
#36337=DIRECTION('',(1.,0.,0.));
#36338=DIRECTION('',(0.,-0.999726448679293,-0.0233886256776472));
#36339=DIRECTION('center_axis',(1.,0.,0.));
#36340=DIRECTION('ref_axis',(0.,-0.642787609686539,0.766044443118978));
#36341=DIRECTION('center_axis',(1.,0.,0.));
#36342=DIRECTION('ref_axis',(0.,1.,0.));
#36343=DIRECTION('center_axis',(0.,0.931436185521974,-0.363904702223363));
#36344=DIRECTION('ref_axis',(0.,0.363904702223363,0.931436185521974));
#36345=DIRECTION('',(-1.,0.,0.));
#36346=DIRECTION('',(0.,0.363904702223363,0.931436185521974));
#36347=DIRECTION('',(1.,0.,0.));
#36348=DIRECTION('',(0.,0.363904702223363,0.931436185521974));
#36349=DIRECTION('center_axis',(1.,0.,0.));
#36350=DIRECTION('ref_axis',(0.,-0.5,0.866025403784439));
#36351=DIRECTION('center_axis',(-1.,0.,0.));
#36352=DIRECTION('ref_axis',(0.,1.,0.));
#36353=DIRECTION('',(0.,-0.988599749777786,0.150567376078944));
#36354=DIRECTION('center_axis',(0.,0.150567376078944,0.988599749777786));
#36355=DIRECTION('ref_axis',(0.,-0.988599749777786,0.150567376078944));
#36356=DIRECTION('',(1.,0.,0.));
#36357=DIRECTION('',(0.,-0.988599749777786,0.150567376078944));
#36358=DIRECTION('center_axis',(1.,0.,0.));
#36359=DIRECTION('ref_axis',(0.,-0.5,0.866025403784439));
#36360=DIRECTION('center_axis',(1.,0.,0.));
#36361=DIRECTION('ref_axis',(0.,1.,0.));
#36362=DIRECTION('center_axis',(0.,0.854094188552644,-0.520118368336094));
#36363=DIRECTION('ref_axis',(0.,0.520118368336094,0.854094188552644));
#36364=DIRECTION('',(-1.,0.,0.));
#36365=DIRECTION('',(0.,0.520118368336094,0.854094188552644));
#36366=DIRECTION('',(1.,0.,0.));
#36367=DIRECTION('',(0.,0.520118368336094,0.854094188552644));
#36368=DIRECTION('center_axis',(1.,0.,0.));
#36369=DIRECTION('ref_axis',(0.,-0.342020143325669,0.939692620785909));
#36370=DIRECTION('center_axis',(-1.,0.,0.));
#36371=DIRECTION('ref_axis',(0.,1.,0.));
#36372=DIRECTION('',(0.,-0.947434947734893,0.319948464304145));
#36373=DIRECTION('center_axis',(0.,0.319948464304145,0.947434947734893));
#36374=DIRECTION('ref_axis',(0.,-0.947434947734893,0.319948464304145));
#36375=DIRECTION('',(1.,0.,0.));
#36376=DIRECTION('',(0.,-0.947434947734893,0.319948464304145));
#36377=DIRECTION('center_axis',(1.,0.,0.));
#36378=DIRECTION('ref_axis',(0.,-0.342020143325669,0.939692620785909));
#36379=DIRECTION('center_axis',(1.,0.,0.));
#36380=DIRECTION('ref_axis',(0.,1.,0.));
#36381=DIRECTION('center_axis',(0.,0.750800971856654,-0.660528501019527));
#36382=DIRECTION('ref_axis',(0.,0.660528501019527,0.750800971856654));
#36383=DIRECTION('',(-1.,0.,0.));
#36384=DIRECTION('',(0.,0.660528501019527,0.750800971856654));
#36385=DIRECTION('',(1.,0.,0.));
#36386=DIRECTION('',(0.,0.660528501019527,0.750800971856654));
#36387=DIRECTION('center_axis',(1.,0.,0.));
#36388=DIRECTION('ref_axis',(0.,-0.17364817766693,0.984807753012208));
#36389=DIRECTION('center_axis',(-1.,0.,0.));
#36390=DIRECTION('ref_axis',(0.,1.,0.));
#36391=DIRECTION('',(0.,-0.877482814230291,0.479608080343199));
#36392=DIRECTION('center_axis',(0.,0.479608080343199,0.877482814230291));
#36393=DIRECTION('ref_axis',(0.,-0.877482814230291,0.479608080343199));
#36394=DIRECTION('',(1.,0.,0.));
#36395=DIRECTION('',(0.,-0.877482814230291,0.479608080343199));
#36396=DIRECTION('center_axis',(1.,0.,0.));
#36397=DIRECTION('ref_axis',(0.,-0.17364817766693,0.984807753012208));
#36398=DIRECTION('center_axis',(1.,0.,0.));
#36399=DIRECTION('ref_axis',(0.,1.,0.));
#36400=DIRECTION('center_axis',(0.,0.624695047554424,-0.780868809443031));
#36401=DIRECTION('ref_axis',(0.,0.780868809443031,0.624695047554424));
#36402=DIRECTION('',(-1.,0.,0.));
#36403=DIRECTION('',(0.,0.780868809443031,0.624695047554424));
#36404=DIRECTION('',(1.,0.,0.));
#36405=DIRECTION('',(0.,0.780868809443031,0.624695047554424));
#36406=DIRECTION('center_axis',(1.,0.,0.));
#36407=DIRECTION('ref_axis',(0.,1.22464679914735E-16,1.));
#36408=DIRECTION('center_axis',(-1.,0.,0.));
#36409=DIRECTION('ref_axis',(0.,1.,0.));
#36410=DIRECTION('',(0.,-0.78086880944303,0.624695047554424));
#36411=DIRECTION('center_axis',(-1.,0.,0.));
#36412=DIRECTION('ref_axis',(0.,1.,0.));
#36413=DIRECTION('center_axis',(0.,0.624695047554424,0.78086880944303));
#36414=DIRECTION('ref_axis',(0.,-0.78086880944303,0.624695047554424));
#36415=DIRECTION('',(1.,0.,0.));
#36416=DIRECTION('',(0.,-0.78086880944303,0.624695047554424));
#36417=DIRECTION('center_axis',(1.,0.,0.));
#36418=DIRECTION('ref_axis',(0.,1.22464679914735E-16,1.));
#36419=DIRECTION('center_axis',(1.,0.,0.));
#36420=DIRECTION('ref_axis',(0.,1.,0.));
#36421=DIRECTION('center_axis',(1.,0.,0.));
#36422=DIRECTION('ref_axis',(0.,1.,0.));
#36423=DIRECTION('center_axis',(0.,0.479608080343199,-0.877482814230291));
#36424=DIRECTION('ref_axis',(0.,0.877482814230291,0.479608080343199));
#36425=DIRECTION('',(-1.,0.,0.));
#36426=DIRECTION('',(0.,0.877482814230291,0.479608080343199));
#36427=DIRECTION('',(1.,0.,0.));
#36428=DIRECTION('',(0.,0.877482814230291,0.479608080343199));
#36429=DIRECTION('center_axis',(1.,0.,0.));
#36430=DIRECTION('ref_axis',(0.,0.173648177666931,0.984807753012208));
#36431=DIRECTION('center_axis',(-1.,0.,0.));
#36432=DIRECTION('ref_axis',(0.,1.,0.));
#36433=DIRECTION('',(0.,-0.660528501019527,0.750800971856655));
#36434=DIRECTION('center_axis',(0.,0.750800971856655,0.660528501019527));
#36435=DIRECTION('ref_axis',(0.,-0.660528501019527,0.750800971856655));
#36436=DIRECTION('',(1.,0.,0.));
#36437=DIRECTION('',(0.,-0.660528501019527,0.750800971856655));
#36438=DIRECTION('center_axis',(1.,0.,0.));
#36439=DIRECTION('ref_axis',(0.,0.173648177666931,0.984807753012208));
#36440=DIRECTION('center_axis',(1.,0.,0.));
#36441=DIRECTION('ref_axis',(0.,1.,0.));
#36442=DIRECTION('center_axis',(0.,0.319948464304145,-0.947434947734893));
#36443=DIRECTION('ref_axis',(0.,0.947434947734893,0.319948464304145));
#36444=DIRECTION('',(-1.,0.,0.));
#36445=DIRECTION('',(0.,0.947434947734893,0.319948464304144));
#36446=DIRECTION('',(1.,0.,0.));
#36447=DIRECTION('',(0.,0.947434947734893,0.319948464304144));
#36448=DIRECTION('center_axis',(1.,0.,0.));
#36449=DIRECTION('ref_axis',(0.,0.342020143325669,0.939692620785908));
#36450=DIRECTION('center_axis',(-1.,0.,0.));
#36451=DIRECTION('ref_axis',(0.,1.,0.));
#36452=DIRECTION('',(0.,-0.520118368336094,0.854094188552644));
#36453=DIRECTION('center_axis',(0.,0.854094188552644,0.520118368336094));
#36454=DIRECTION('ref_axis',(0.,-0.520118368336094,0.854094188552644));
#36455=DIRECTION('',(1.,0.,0.));
#36456=DIRECTION('',(0.,-0.520118368336094,0.854094188552644));
#36457=DIRECTION('center_axis',(1.,0.,0.));
#36458=DIRECTION('ref_axis',(0.,0.342020143325669,0.939692620785908));
#36459=DIRECTION('center_axis',(1.,0.,0.));
#36460=DIRECTION('ref_axis',(0.,1.,0.));
#36461=DIRECTION('center_axis',(0.,0.150567376078944,-0.988599749777787));
#36462=DIRECTION('ref_axis',(0.,0.988599749777787,0.150567376078944));
#36463=DIRECTION('',(-1.,0.,0.));
#36464=DIRECTION('',(0.,0.988599749777787,0.150567376078944));
#36465=DIRECTION('',(1.,0.,0.));
#36466=DIRECTION('',(0.,0.988599749777787,0.150567376078944));
#36467=DIRECTION('center_axis',(1.,0.,0.));
#36468=DIRECTION('ref_axis',(0.,0.5,0.866025403784439));
#36469=DIRECTION('center_axis',(-1.,0.,0.));
#36470=DIRECTION('ref_axis',(0.,1.,0.));
#36471=DIRECTION('',(0.,-0.363904702223363,0.931436185521974));
#36472=DIRECTION('center_axis',(0.,0.931436185521974,0.363904702223363));
#36473=DIRECTION('ref_axis',(0.,-0.363904702223363,0.931436185521974));
#36474=DIRECTION('',(1.,0.,0.));
#36475=DIRECTION('',(0.,-0.363904702223363,0.931436185521974));
#36476=DIRECTION('center_axis',(1.,0.,0.));
#36477=DIRECTION('ref_axis',(0.,0.5,0.866025403784439));
#36478=DIRECTION('center_axis',(1.,0.,0.));
#36479=DIRECTION('ref_axis',(0.,1.,0.));
#36480=DIRECTION('center_axis',(0.,-0.0233886256776474,-0.999726448679293));
#36481=DIRECTION('ref_axis',(0.,0.999726448679293,-0.0233886256776474));
#36482=DIRECTION('',(-1.,0.,0.));
#36483=DIRECTION('',(0.,0.999726448679293,-0.0233886256776475));
#36484=DIRECTION('',(1.,0.,0.));
#36485=DIRECTION('',(0.,0.999726448679293,-0.0233886256776475));
#36486=DIRECTION('center_axis',(1.,0.,0.));
#36487=DIRECTION('ref_axis',(0.,0.642787609686539,0.766044443118978));
#36488=DIRECTION('center_axis',(-1.,0.,0.));
#36489=DIRECTION('ref_axis',(0.,1.,0.));
#36490=DIRECTION('',(0.,-0.196633975878238,0.980476965323672));
#36491=DIRECTION('center_axis',(0.,0.980476965323672,0.196633975878238));
#36492=DIRECTION('ref_axis',(0.,-0.196633975878238,0.980476965323672));
#36493=DIRECTION('',(1.,0.,0.));
#36494=DIRECTION('',(0.,-0.196633975878238,0.980476965323672));
#36495=DIRECTION('center_axis',(1.,0.,0.));
#36496=DIRECTION('ref_axis',(0.,0.642787609686539,0.766044443118978));
#36497=DIRECTION('center_axis',(1.,0.,0.));
#36498=DIRECTION('ref_axis',(0.,1.,0.));
#36499=DIRECTION('center_axis',(0.,-0.196633975878238,-0.980476965323672));
#36500=DIRECTION('ref_axis',(0.,0.980476965323672,-0.196633975878239));
#36501=DIRECTION('',(-1.,0.,0.));
#36502=DIRECTION('',(0.,0.980476965323672,-0.196633975878239));
#36503=DIRECTION('',(1.,0.,0.));
#36504=DIRECTION('',(0.,0.980476965323672,-0.196633975878239));
#36505=DIRECTION('center_axis',(1.,0.,0.));
#36506=DIRECTION('ref_axis',(0.,0.766044443118978,0.642787609686539));
#36507=DIRECTION('center_axis',(-1.,0.,0.));
#36508=DIRECTION('ref_axis',(0.,1.,0.));
#36509=DIRECTION('',(0.,-0.0233886256776473,0.999726448679293));
#36510=DIRECTION('center_axis',(0.,0.999726448679293,0.0233886256776472));
#36511=DIRECTION('ref_axis',(0.,-0.0233886256776472,0.999726448679293));
#36512=DIRECTION('',(1.,0.,0.));
#36513=DIRECTION('',(0.,-0.0233886256776473,0.999726448679293));
#36514=DIRECTION('center_axis',(1.,0.,0.));
#36515=DIRECTION('ref_axis',(0.,0.766044443118978,0.642787609686539));
#36516=DIRECTION('center_axis',(1.,0.,0.));
#36517=DIRECTION('ref_axis',(0.,1.,0.));
#36518=DIRECTION('center_axis',(0.,-0.363904702223363,-0.931436185521974));
#36519=DIRECTION('ref_axis',(0.,0.931436185521974,-0.363904702223363));
#36520=DIRECTION('',(-1.,0.,0.));
#36521=DIRECTION('',(0.,0.931436185521974,-0.363904702223363));
#36522=DIRECTION('',(1.,0.,0.));
#36523=DIRECTION('',(0.,0.931436185521974,-0.363904702223363));
#36524=DIRECTION('center_axis',(1.,0.,0.));
#36525=DIRECTION('ref_axis',(0.,0.866025403784439,0.5));
#36526=DIRECTION('center_axis',(-1.,0.,0.));
#36527=DIRECTION('ref_axis',(0.,1.,0.));
#36528=DIRECTION('',(0.,0.150567376078944,0.988599749777786));
#36529=DIRECTION('center_axis',(0.,0.988599749777786,-0.150567376078944));
#36530=DIRECTION('ref_axis',(0.,0.150567376078944,0.988599749777786));
#36531=DIRECTION('',(1.,0.,0.));
#36532=DIRECTION('',(0.,0.150567376078944,0.988599749777786));
#36533=DIRECTION('center_axis',(1.,0.,0.));
#36534=DIRECTION('ref_axis',(0.,0.866025403784439,0.5));
#36535=DIRECTION('center_axis',(1.,0.,0.));
#36536=DIRECTION('ref_axis',(0.,1.,0.));
#36537=DIRECTION('center_axis',(0.,-0.520118368336094,-0.854094188552644));
#36538=DIRECTION('ref_axis',(0.,0.854094188552644,-0.520118368336094));
#36539=DIRECTION('',(-1.,0.,0.));
#36540=DIRECTION('',(0.,0.854094188552644,-0.520118368336094));
#36541=DIRECTION('',(1.,0.,0.));
#36542=DIRECTION('',(0.,0.854094188552644,-0.520118368336094));
#36543=DIRECTION('center_axis',(1.,0.,0.));
#36544=DIRECTION('ref_axis',(0.,0.939692620785908,0.342020143325669));
#36545=DIRECTION('center_axis',(-1.,0.,0.));
#36546=DIRECTION('ref_axis',(0.,1.,0.));
#36547=DIRECTION('',(0.,0.319948464304145,0.947434947734893));
#36548=DIRECTION('center_axis',(0.,0.947434947734893,-0.319948464304145));
#36549=DIRECTION('ref_axis',(0.,0.319948464304145,0.947434947734893));
#36550=DIRECTION('',(1.,0.,0.));
#36551=DIRECTION('',(0.,0.319948464304145,0.947434947734893));
#36552=DIRECTION('center_axis',(1.,0.,0.));
#36553=DIRECTION('ref_axis',(0.,0.939692620785908,0.342020143325669));
#36554=DIRECTION('center_axis',(1.,0.,0.));
#36555=DIRECTION('ref_axis',(0.,1.,0.));
#36556=DIRECTION('center_axis',(0.,-0.660528501019527,-0.750800971856654));
#36557=DIRECTION('ref_axis',(0.,0.750800971856654,-0.660528501019527));
#36558=DIRECTION('',(-1.,0.,0.));
#36559=DIRECTION('',(0.,0.750800971856654,-0.660528501019527));
#36560=DIRECTION('',(1.,0.,0.));
#36561=DIRECTION('',(0.,0.750800971856654,-0.660528501019527));
#36562=DIRECTION('center_axis',(1.,0.,0.));
#36563=DIRECTION('ref_axis',(0.,0.984807753012208,0.17364817766693));
#36564=DIRECTION('center_axis',(-1.,0.,0.));
#36565=DIRECTION('ref_axis',(0.,1.,0.));
#36566=DIRECTION('',(0.,0.479608080343199,0.877482814230291));
#36567=DIRECTION('center_axis',(0.,0.877482814230291,-0.479608080343199));
#36568=DIRECTION('ref_axis',(0.,0.479608080343199,0.877482814230291));
#36569=DIRECTION('',(1.,0.,0.));
#36570=DIRECTION('',(0.,0.479608080343199,0.877482814230291));
#36571=DIRECTION('center_axis',(1.,0.,0.));
#36572=DIRECTION('ref_axis',(0.,0.984807753012208,0.17364817766693));
#36573=DIRECTION('center_axis',(1.,0.,0.));
#36574=DIRECTION('ref_axis',(0.,1.,0.));
#36575=DIRECTION('center_axis',(0.,-0.780868809443031,-0.624695047554424));
#36576=DIRECTION('ref_axis',(0.,0.624695047554424,-0.780868809443031));
#36577=DIRECTION('',(-1.,0.,0.));
#36578=DIRECTION('',(0.,0.624695047554424,-0.78086880944303));
#36579=DIRECTION('',(1.,0.,0.));
#36580=DIRECTION('',(0.,0.624695047554424,-0.78086880944303));
#36581=DIRECTION('center_axis',(1.,0.,0.));
#36582=DIRECTION('ref_axis',(0.,1.,-6.12323399573677E-17));
#36583=DIRECTION('center_axis',(-1.,0.,0.));
#36584=DIRECTION('ref_axis',(0.,1.,0.));
#36585=DIRECTION('',(0.,0.624695047554424,0.78086880944303));
#36586=DIRECTION('center_axis',(0.,0.780868809443031,-0.624695047554424));
#36587=DIRECTION('ref_axis',(0.,0.624695047554424,0.780868809443031));
#36588=DIRECTION('',(1.,0.,0.));
#36589=DIRECTION('',(0.,0.624695047554424,0.78086880944303));
#36590=DIRECTION('center_axis',(1.,0.,0.));
#36591=DIRECTION('ref_axis',(0.,1.,-6.12323399573677E-17));
#36592=DIRECTION('center_axis',(1.,0.,0.));
#36593=DIRECTION('ref_axis',(0.,1.,0.));
#36594=DIRECTION('center_axis',(0.,-0.877482814230291,-0.479608080343199));
#36595=DIRECTION('ref_axis',(0.,0.479608080343199,-0.877482814230291));
#36596=DIRECTION('',(-1.,0.,0.));
#36597=DIRECTION('',(0.,0.479608080343199,-0.877482814230291));
#36598=DIRECTION('',(1.,0.,0.));
#36599=DIRECTION('',(0.,0.479608080343199,-0.877482814230291));
#36600=DIRECTION('center_axis',(1.,0.,0.));
#36601=DIRECTION('ref_axis',(0.,0.984807753012208,-0.17364817766693));
#36602=DIRECTION('center_axis',(-1.,0.,0.));
#36603=DIRECTION('ref_axis',(0.,1.,0.));
#36604=DIRECTION('',(0.,0.750800971856654,0.660528501019527));
#36605=DIRECTION('center_axis',(0.,0.660528501019527,-0.750800971856655));
#36606=DIRECTION('ref_axis',(0.,0.750800971856654,0.660528501019527));
#36607=DIRECTION('',(1.,0.,0.));
#36608=DIRECTION('',(0.,0.750800971856654,0.660528501019527));
#36609=DIRECTION('center_axis',(1.,0.,0.));
#36610=DIRECTION('ref_axis',(0.,0.984807753012208,-0.17364817766693));
#36611=DIRECTION('center_axis',(1.,0.,0.));
#36612=DIRECTION('ref_axis',(0.,1.,0.));
#36613=DIRECTION('center_axis',(0.,-0.947434947734893,-0.319948464304145));
#36614=DIRECTION('ref_axis',(0.,0.319948464304145,-0.947434947734893));
#36615=DIRECTION('',(-1.,0.,0.));
#36616=DIRECTION('',(0.,0.319948464304145,-0.947434947734893));
#36617=DIRECTION('',(1.,0.,0.));
#36618=DIRECTION('',(0.,0.319948464304145,-0.947434947734893));
#36619=DIRECTION('center_axis',(1.,0.,0.));
#36620=DIRECTION('ref_axis',(0.,0.939692620785908,-0.342020143325669));
#36621=DIRECTION('center_axis',(-1.,0.,0.));
#36622=DIRECTION('ref_axis',(0.,1.,0.));
#36623=DIRECTION('',(0.,0.854094188552644,0.520118368336094));
#36624=DIRECTION('center_axis',(0.,0.520118368336094,-0.854094188552644));
#36625=DIRECTION('ref_axis',(0.,0.854094188552644,0.520118368336094));
#36626=DIRECTION('',(1.,0.,0.));
#36627=DIRECTION('',(0.,0.854094188552644,0.520118368336094));
#36628=DIRECTION('center_axis',(1.,0.,0.));
#36629=DIRECTION('ref_axis',(0.,0.939692620785908,-0.342020143325669));
#36630=DIRECTION('center_axis',(1.,0.,0.));
#36631=DIRECTION('ref_axis',(0.,1.,0.));
#36632=DIRECTION('center_axis',(0.,-0.988599749777787,-0.150567376078944));
#36633=DIRECTION('ref_axis',(0.,0.150567376078944,-0.988599749777787));
#36634=DIRECTION('',(-1.,0.,0.));
#36635=DIRECTION('',(0.,0.150567376078944,-0.988599749777787));
#36636=DIRECTION('',(1.,0.,0.));
#36637=DIRECTION('',(0.,0.150567376078944,-0.988599749777787));
#36638=DIRECTION('center_axis',(1.,0.,0.));
#36639=DIRECTION('ref_axis',(0.,0.866025403784439,-0.5));
#36640=DIRECTION('center_axis',(-1.,0.,0.));
#36641=DIRECTION('ref_axis',(0.,1.,0.));
#36642=DIRECTION('',(0.,0.931436185521974,0.363904702223362));
#36643=DIRECTION('center_axis',(0.,0.363904702223362,-0.931436185521974));
#36644=DIRECTION('ref_axis',(0.,0.931436185521974,0.363904702223362));
#36645=DIRECTION('',(1.,0.,0.));
#36646=DIRECTION('',(0.,0.931436185521974,0.363904702223362));
#36647=DIRECTION('center_axis',(1.,0.,0.));
#36648=DIRECTION('ref_axis',(0.,0.866025403784439,-0.5));
#36649=DIRECTION('center_axis',(1.,0.,0.));
#36650=DIRECTION('ref_axis',(0.,1.,0.));
#36651=DIRECTION('center_axis',(0.,-0.999726448679293,0.0233886256776472));
#36652=DIRECTION('ref_axis',(0.,-0.0233886256776472,-0.999726448679293));
#36653=DIRECTION('',(-1.,0.,0.));
#36654=DIRECTION('',(0.,-0.0233886256776473,-0.999726448679293));
#36655=DIRECTION('',(1.,0.,0.));
#36656=DIRECTION('',(0.,-0.0233886256776473,-0.999726448679293));
#36657=DIRECTION('center_axis',(1.,0.,0.));
#36658=DIRECTION('ref_axis',(0.,0.766044443118978,-0.642787609686539));
#36659=DIRECTION('center_axis',(-1.,0.,0.));
#36660=DIRECTION('ref_axis',(0.,1.,0.));
#36661=DIRECTION('',(0.,0.980476965323672,0.196633975878239));
#36662=DIRECTION('center_axis',(0.,0.196633975878238,-0.980476965323672));
#36663=DIRECTION('ref_axis',(0.,0.980476965323672,0.196633975878239));
#36664=DIRECTION('',(1.,0.,0.));
#36665=DIRECTION('',(0.,0.980476965323672,0.196633975878239));
#36666=DIRECTION('center_axis',(1.,0.,0.));
#36667=DIRECTION('ref_axis',(0.,0.766044443118978,-0.642787609686539));
#36668=DIRECTION('center_axis',(1.,0.,0.));
#36669=DIRECTION('ref_axis',(0.,1.,0.));
#36670=DIRECTION('center_axis',(0.,-0.980476965323672,0.196633975878239));
#36671=DIRECTION('ref_axis',(0.,-0.196633975878239,-0.980476965323671));
#36672=DIRECTION('',(-1.,0.,0.));
#36673=DIRECTION('',(0.,-0.196633975878239,-0.980476965323671));
#36674=DIRECTION('',(1.,0.,0.));
#36675=DIRECTION('',(0.,-0.196633975878239,-0.980476965323671));
#36676=DIRECTION('center_axis',(1.,0.,0.));
#36677=DIRECTION('ref_axis',(0.,0.642787609686539,-0.766044443118978));
#36678=DIRECTION('center_axis',(-1.,0.,0.));
#36679=DIRECTION('ref_axis',(0.,1.,0.));
#36680=DIRECTION('',(0.,0.999726448679293,0.0233886256776472));
#36681=DIRECTION('center_axis',(0.,0.0233886256776472,-0.999726448679293));
#36682=DIRECTION('ref_axis',(0.,0.999726448679293,0.0233886256776472));
#36683=DIRECTION('',(1.,0.,0.));
#36684=DIRECTION('',(0.,0.999726448679293,0.0233886256776472));
#36685=DIRECTION('center_axis',(1.,0.,0.));
#36686=DIRECTION('ref_axis',(0.,0.642787609686539,-0.766044443118978));
#36687=DIRECTION('center_axis',(1.,0.,0.));
#36688=DIRECTION('ref_axis',(0.,1.,0.));
#36689=DIRECTION('center_axis',(0.,-0.931436185521974,0.363904702223363));
#36690=DIRECTION('ref_axis',(0.,-0.363904702223363,-0.931436185521974));
#36691=DIRECTION('',(-1.,0.,0.));
#36692=DIRECTION('',(0.,-0.363904702223363,-0.931436185521974));
#36693=DIRECTION('',(1.,0.,0.));
#36694=DIRECTION('',(0.,-0.363904702223363,-0.931436185521974));
#36695=DIRECTION('center_axis',(1.,0.,0.));
#36696=DIRECTION('ref_axis',(0.,0.5,-0.866025403784439));
#36697=DIRECTION('center_axis',(-1.,0.,0.));
#36698=DIRECTION('ref_axis',(0.,1.,0.));
#36699=DIRECTION('',(0.,0.988599749777787,-0.150567376078944));
#36700=DIRECTION('center_axis',(0.,-0.150567376078944,-0.988599749777787));
#36701=DIRECTION('ref_axis',(0.,0.988599749777787,-0.150567376078944));
#36702=DIRECTION('',(1.,0.,0.));
#36703=DIRECTION('',(0.,0.988599749777787,-0.150567376078944));
#36704=DIRECTION('center_axis',(1.,0.,0.));
#36705=DIRECTION('ref_axis',(0.,0.5,-0.866025403784439));
#36706=DIRECTION('center_axis',(1.,0.,0.));
#36707=DIRECTION('ref_axis',(0.,1.,0.));
#36708=DIRECTION('center_axis',(0.,-0.854094188552644,0.520118368336094));
#36709=DIRECTION('ref_axis',(0.,-0.520118368336094,-0.854094188552644));
#36710=DIRECTION('',(-1.,0.,0.));
#36711=DIRECTION('',(0.,-0.520118368336094,-0.854094188552644));
#36712=DIRECTION('',(1.,0.,0.));
#36713=DIRECTION('',(0.,-0.520118368336094,-0.854094188552644));
#36714=DIRECTION('center_axis',(1.,0.,0.));
#36715=DIRECTION('ref_axis',(0.,0.342020143325669,-0.939692620785908));
#36716=DIRECTION('center_axis',(-1.,0.,0.));
#36717=DIRECTION('ref_axis',(0.,1.,0.));
#36718=DIRECTION('',(0.,0.947434947734893,-0.319948464304145));
#36719=DIRECTION('center_axis',(0.,-0.319948464304145,-0.947434947734893));
#36720=DIRECTION('ref_axis',(0.,0.947434947734893,-0.319948464304145));
#36721=DIRECTION('',(1.,0.,0.));
#36722=DIRECTION('',(0.,0.947434947734893,-0.319948464304145));
#36723=DIRECTION('center_axis',(1.,0.,0.));
#36724=DIRECTION('ref_axis',(0.,0.342020143325669,-0.939692620785908));
#36725=DIRECTION('center_axis',(1.,0.,0.));
#36726=DIRECTION('ref_axis',(0.,1.,0.));
#36727=DIRECTION('center_axis',(0.,-0.750800971856655,0.660528501019527));
#36728=DIRECTION('ref_axis',(0.,-0.660528501019527,-0.750800971856654));
#36729=DIRECTION('',(-1.,0.,0.));
#36730=DIRECTION('',(0.,-0.660528501019527,-0.750800971856654));
#36731=DIRECTION('',(1.,0.,0.));
#36732=DIRECTION('',(0.,-0.660528501019527,-0.750800971856654));
#36733=DIRECTION('center_axis',(1.,0.,0.));
#36734=DIRECTION('ref_axis',(0.,0.17364817766693,-0.984807753012208));
#36735=DIRECTION('center_axis',(-1.,0.,0.));
#36736=DIRECTION('ref_axis',(0.,1.,0.));
#36737=DIRECTION('',(0.,0.877482814230291,-0.479608080343199));
#36738=DIRECTION('center_axis',(0.,-0.479608080343199,-0.877482814230291));
#36739=DIRECTION('ref_axis',(0.,0.877482814230291,-0.479608080343199));
#36740=DIRECTION('',(1.,0.,0.));
#36741=DIRECTION('',(0.,0.877482814230291,-0.479608080343199));
#36742=DIRECTION('center_axis',(1.,0.,0.));
#36743=DIRECTION('ref_axis',(0.,0.17364817766693,-0.984807753012208));
#36744=DIRECTION('center_axis',(1.,0.,0.));
#36745=DIRECTION('ref_axis',(0.,1.,0.));
#36746=DIRECTION('center_axis',(0.,-0.624695047554424,0.780868809443031));
#36747=DIRECTION('ref_axis',(0.,-0.780868809443031,-0.624695047554424));
#36748=DIRECTION('',(-1.,0.,0.));
#36749=DIRECTION('',(0.,-0.78086880944303,-0.624695047554424));
#36750=DIRECTION('',(1.,0.,0.));
#36751=DIRECTION('',(0.,-0.78086880944303,-0.624695047554424));
#36752=DIRECTION('center_axis',(1.,0.,0.));
#36753=DIRECTION('ref_axis',(0.,0.,-1.));
#36754=DIRECTION('center_axis',(-1.,0.,0.));
#36755=DIRECTION('ref_axis',(0.,1.,0.));
#36756=DIRECTION('',(0.,0.78086880944303,-0.624695047554424));
#36757=DIRECTION('center_axis',(0.,-0.624695047554424,-0.780868809443031));
#36758=DIRECTION('ref_axis',(0.,0.780868809443031,-0.624695047554424));
#36759=DIRECTION('',(1.,0.,0.));
#36760=DIRECTION('',(0.,0.78086880944303,-0.624695047554424));
#36761=DIRECTION('center_axis',(1.,0.,0.));
#36762=DIRECTION('ref_axis',(0.,0.,-1.));
#36763=DIRECTION('center_axis',(1.,0.,0.));
#36764=DIRECTION('ref_axis',(0.,1.,0.));
#36765=DIRECTION('center_axis',(1.,0.,0.));
#36766=DIRECTION('ref_axis',(0.,1.,0.));
#36767=DIRECTION('',(0.517550572850554,-0.855652619082103,-1.04787224114095E-16));
#36768=DIRECTION('center_axis',(-1.,0.,0.));
#36769=DIRECTION('ref_axis',(0.,1.,0.));
#36770=DIRECTION('center_axis',(0.,0.5,0.866025403784439));
#36771=DIRECTION('ref_axis',(0.,0.866025403784439,-0.5));
#36772=DIRECTION('',(0.,0.866025403784439,-0.5));
#36773=DIRECTION('',(-1.,0.,0.));
#36774=DIRECTION('',(0.,0.866025403784439,-0.5));
#36775=DIRECTION('',(-1.,0.,0.));
#36776=DIRECTION('center_axis',(0.,-0.5,0.866025403784439));
#36777=DIRECTION('ref_axis',(0.,0.866025403784439,0.5));
#36778=DIRECTION('',(0.,0.866025403784439,0.5));
#36779=DIRECTION('',(-1.,0.,0.));
#36780=DIRECTION('',(0.,0.866025403784439,0.5));
#36781=DIRECTION('center_axis',(0.,-1.,-1.92296268638356E-16));
#36782=DIRECTION('ref_axis',(0.,-1.92296268638356E-16,1.));
#36783=DIRECTION('',(0.,-1.92296268638356E-16,1.));
#36784=DIRECTION('',(-1.,0.,0.));
#36785=DIRECTION('',(0.,-1.92296268638356E-16,1.));
#36786=DIRECTION('center_axis',(0.,-0.5,-0.866025403784439));
#36787=DIRECTION('ref_axis',(0.,-0.866025403784439,0.5));
#36788=DIRECTION('',(0.,-0.866025403784439,0.5));
#36789=DIRECTION('',(-1.,0.,0.));
#36790=DIRECTION('',(0.,-0.866025403784439,0.5));
#36791=DIRECTION('center_axis',(0.,0.5,-0.866025403784439));
#36792=DIRECTION('ref_axis',(0.,-0.866025403784439,-0.5));
#36793=DIRECTION('',(0.,-0.866025403784439,-0.5));
#36794=DIRECTION('',(-1.,0.,0.));
#36795=DIRECTION('',(0.,-0.866025403784439,-0.5));
#36796=DIRECTION('center_axis',(0.,1.,-3.84592537276713E-16));
#36797=DIRECTION('ref_axis',(0.,-3.84592537276713E-16,-1.));
#36798=DIRECTION('',(0.,-3.84592537276713E-16,-1.));
#36799=DIRECTION('',(0.,-3.84592537276713E-16,-1.));
#36800=DIRECTION('center_axis',(-1.,0.,0.));
#36801=DIRECTION('ref_axis',(0.,0.,1.));
#36802=DIRECTION('center_axis',(1.,0.,0.));
#36803=DIRECTION('ref_axis',(0.,0.,-1.));
#36804=DIRECTION('center_axis',(1.,0.,0.));
#36805=DIRECTION('ref_axis',(0.,-1.,1.83697019872103E-16));
#36806=DIRECTION('center_axis',(0.,-1.,-1.22464679914735E-16));
#36807=DIRECTION('ref_axis',(0.,-1.22464679914735E-16,1.));
#36808=DIRECTION('center_axis',(-1.,0.,0.));
#36809=DIRECTION('ref_axis',(0.,-1.,1.83697019872103E-16));
#36810=DIRECTION('center_axis',(1.,0.,0.));
#36811=DIRECTION('ref_axis',(0.,-1.,1.83697019872103E-16));
#36812=DIRECTION('center_axis',(1.,0.,0.));
#36813=DIRECTION('ref_axis',(0.,1.,0.));
#36814=DIRECTION('',(-1.,0.,0.));
#36815=DIRECTION('center_axis',(1.,0.,0.));
#36816=DIRECTION('ref_axis',(0.,0.,-1.));
#36817=DIRECTION('center_axis',(-1.,0.,0.));
#36818=DIRECTION('ref_axis',(0.,0.,1.));
#36819=DIRECTION('center_axis',(1.,0.,0.));
#36820=DIRECTION('ref_axis',(0.,0.,-1.));
#36821=DIRECTION('center_axis',(-1.,0.,0.));
#36822=DIRECTION('ref_axis',(0.,0.,1.));
#36823=DIRECTION('center_axis',(1.,0.,0.));
#36824=DIRECTION('ref_axis',(0.,0.,-1.));
#36825=DIRECTION('center_axis',(1.,0.,0.));
#36826=DIRECTION('ref_axis',(0.,1.,0.));
#36827=DIRECTION('',(-0.707106781186548,0.707106781186547,8.65956056235493E-17));
#36828=DIRECTION('center_axis',(1.,0.,0.));
#36829=DIRECTION('ref_axis',(0.,1.,0.));
#36830=DIRECTION('center_axis',(-1.,0.,0.));
#36831=DIRECTION('ref_axis',(0.,1.,0.));
#36832=DIRECTION('center_axis',(-1.,0.,0.));
#36833=DIRECTION('ref_axis',(0.,1.,0.));
#36834=DIRECTION('center_axis',(1.,0.,0.));
#36835=DIRECTION('ref_axis',(0.,0.,-1.));
#36836=DIRECTION('',(-0.554700196225228,-0.832050294337845,-1.01896772969045E-16));
#36837=DIRECTION('center_axis',(1.,0.,0.));
#36838=DIRECTION('ref_axis',(0.,1.,0.));
#36839=DIRECTION('center_axis',(1.,0.,0.));
#36840=DIRECTION('ref_axis',(0.,0.,-1.));
#36841=DIRECTION('',(-1.,0.,0.));
#36842=DIRECTION('center_axis',(-1.,0.,0.));
#36843=DIRECTION('ref_axis',(0.,0.,1.));
#36844=DIRECTION('center_axis',(1.,0.,0.));
#36845=DIRECTION('ref_axis',(0.,1.,0.));
#36846=DIRECTION('center_axis',(1.,0.,0.));
#36847=DIRECTION('ref_axis',(0.,0.,-1.));
#36848=DIRECTION('',(-1.,0.,0.));
#36849=DIRECTION('',(-1.,0.,0.));
#36850=DIRECTION('center_axis',(-1.,0.,0.));
#36851=DIRECTION('ref_axis',(0.,1.,0.));
#36852=DIRECTION('center_axis',(1.,0.,0.));
#36853=DIRECTION('ref_axis',(0.,0.,-1.));
#36854=DIRECTION('',(-0.707106781186547,-0.707106781186548,-8.65956056235494E-17));
#36855=DIRECTION('center_axis',(1.,0.,0.));
#36856=DIRECTION('ref_axis',(0.,0.,-1.));
#46413=CARTESIAN_POINT('',(0.,0.,0.));
#46414=CARTESIAN_POINT('Origin',(-20.1,0.,0.));
#46415=CARTESIAN_POINT('',(-25.862836477965,-3.93796551936703,0.00241968030858936));
#46416=CARTESIAN_POINT('',(-26.046163522035,-3.93691440463921,0.00389705969986015));
#46417=CARTESIAN_POINT('',(-20.1,-3.933,-4.81653586104654E-16));
#46418=CARTESIAN_POINT('',(-26.267,1.75076268474097,3.52556565592089));
#46419=CARTESIAN_POINT('Ctrl Pts',(-25.862836477965,-3.93796551936703,0.00241968030858936));
#46420=CARTESIAN_POINT('Ctrl Pts',(-25.8692092928874,-3.93880098183899,
0.127947404661549));
#46421=CARTESIAN_POINT('Ctrl Pts',(-25.8755821078097,-3.93332319567765,
0.253396721851654));
#46422=CARTESIAN_POINT('Ctrl Pts',(-25.881954922732,-3.92129417144253,0.378208920623738));
#46423=CARTESIAN_POINT('Ctrl Pts',(-25.948213931562,-3.79622679811926,1.67589803937646));
#46424=CARTESIAN_POINT('Ctrl Pts',(-26.014472940392,-2.96296803864307,2.90471440911298));
#46425=CARTESIAN_POINT('Ctrl Pts',(-26.080731949222,-1.80365763965045,3.50203017167187));
#46426=CARTESIAN_POINT('Ctrl Pts',(-26.1428212994813,-0.717302279173672,
4.06175704129799));
#46427=CARTESIAN_POINT('Ctrl Pts',(-26.2049106497407,0.655359278582525,
4.066962738484));
#46428=CARTESIAN_POINT('Ctrl Pts',(-26.267,1.75283089415091,3.52826931739086));
#46429=CARTESIAN_POINT('',(-26.267,-1.74869447533124,3.52286199445082));
#46430=CARTESIAN_POINT('Origin',(-26.267,0.,0.));
#46431=CARTESIAN_POINT('Ctrl Pts',(-26.267,-1.74869447533123,3.52286199445082));
#46432=CARTESIAN_POINT('Ctrl Pts',(-26.20074099117,-2.92199812251929,2.94045212175197));
#46433=CARTESIAN_POINT('Ctrl Pts',(-26.13448198234,-3.77113385184886,1.73058568782258));
#46434=CARTESIAN_POINT('Ctrl Pts',(-26.06822297351,-3.91479953860179,0.43684538414918));
#46435=CARTESIAN_POINT('Ctrl Pts',(-26.0608698230183,-3.93074296175041,
0.29327144125381));
#46436=CARTESIAN_POINT('Ctrl Pts',(-26.0535166725267,-3.93799806875422,
0.148664537846095));
#46437=CARTESIAN_POINT('Ctrl Pts',(-26.046163522035,-3.93691440463921,0.00389705969986015));
#46438=CARTESIAN_POINT('Origin',(-20.1,0.,0.));
#46439=CARTESIAN_POINT('',(-24.612836477965,-3.92791610626173,0.00232109521066254));
#46440=CARTESIAN_POINT('',(-24.796163522035,-3.92757907140906,0.00208605505030474));
#46441=CARTESIAN_POINT('',(-20.1,-3.933,-4.81653586104654E-16));
#46442=CARTESIAN_POINT('Ctrl Pts',(-24.612836477965,-3.92791610626173,0.00232109521066254));
#46443=CARTESIAN_POINT('Ctrl Pts',(-24.6383219065741,-3.9306200668013,0.507662989981787));
#46444=CARTESIAN_POINT('Ctrl Pts',(-24.6638073351831,-3.84018781632386,
1.01207323610777));
#46445=CARTESIAN_POINT('Ctrl Pts',(-24.6892927637922,-3.65215730231515,
1.47701096116609));
#46446=CARTESIAN_POINT('Ctrl Pts',(-24.7555517726221,-3.16330087854708,
2.68579239084588));
#46447=CARTESIAN_POINT('Ctrl Pts',(-24.8218107814521,-2.01474203513748,
3.62776458934148));
#46448=CARTESIAN_POINT('Ctrl Pts',(-24.8880697902821,-0.733655209919689,
3.87059482446554));
#46449=CARTESIAN_POINT('Ctrl Pts',(-24.9543287991121,0.547431615298105,
4.1134250595896));
#46450=CARTESIAN_POINT('Ctrl Pts',(-25.0205878079421,1.96104642232409,3.65711333134211));
#46451=CARTESIAN_POINT('Ctrl Pts',(-25.0868468167721,2.8583382289552,2.71105327307234));
#46452=CARTESIAN_POINT('Ctrl Pts',(-25.1531058256021,3.7556300355863,1.76499321480257));
#46453=CARTESIAN_POINT('Ctrl Pts',(-25.2193648344321,4.13659884182251,0.329184826510518));
#46454=CARTESIAN_POINT('Ctrl Pts',(-25.2856238432621,3.82640530464537,-0.937248424257726));
#46455=CARTESIAN_POINT('Ctrl Pts',(-25.3518828520921,3.51621176746824,-2.20368167502597));
#46456=CARTESIAN_POINT('Ctrl Pts',(-25.4181418609221,2.51485588687775,-3.30073978827041));
#46457=CARTESIAN_POINT('Ctrl Pts',(-25.4844008697521,1.28190902568355,-3.72506985025129));
#46458=CARTESIAN_POINT('Ctrl Pts',(-25.5506598785821,0.0489621644893422,
-4.14939991223217));
#46459=CARTESIAN_POINT('Ctrl Pts',(-25.616918887412,-1.41557567730859,-3.90100192294949));
#46460=CARTESIAN_POINT('Ctrl Pts',(-25.683177896242,-2.43940660462237,-3.0935219944237));
#46461=CARTESIAN_POINT('Ctrl Pts',(-25.7430640901497,-3.3647651109516,-2.36370577123936));
#46462=CARTESIAN_POINT('Ctrl Pts',(-25.8029502840574,-3.9301145668118,-1.17718112922547));
#46463=CARTESIAN_POINT('Ctrl Pts',(-25.862836477965,-3.93796551936703,0.00241968030858936));
#46464=CARTESIAN_POINT('Ctrl Pts',(-26.046163522035,-3.93691440463921,0.00389705969986015));
#46465=CARTESIAN_POINT('Ctrl Pts',(-25.9872576636967,-3.92823320534685,
-1.15583067459948));
#46466=CARTESIAN_POINT('Ctrl Pts',(-25.9283518053584,-3.38440620529298,
-2.32586339218745));
#46467=CARTESIAN_POINT('Ctrl Pts',(-25.86944594702,-2.48513760513297,-3.05769982285182));
#46468=CARTESIAN_POINT('Ctrl Pts',(-25.80318693819,-1.47361434073496,-3.88089055276197));
#46469=CARTESIAN_POINT('Ctrl Pts',(-25.73692792936,-0.0123721677626969,
-4.14965783916484));
#46470=CARTESIAN_POINT('Ctrl Pts',(-25.6706689205301,1.22684276968273,-3.74329298057656));
#46471=CARTESIAN_POINT('Ctrl Pts',(-25.6044099117001,2.46605770712816,-3.33692812198827));
#46472=CARTESIAN_POINT('Ctrl Pts',(-25.5381509028701,3.48324540904674,-2.25543111840884));
#46473=CARTESIAN_POINT('Ctrl Pts',(-25.4718918940401,3.81205929712905,-0.993876849486107));
#46474=CARTESIAN_POINT('Ctrl Pts',(-25.4056328852101,4.14087318521135,0.267677419436621));
#46475=CARTESIAN_POINT('Ctrl Pts',(-25.3393738763801,3.78131325945737,1.70928895370264));
#46476=CARTESIAN_POINT('Ctrl Pts',(-25.2731148675501,2.89813926393057,2.66858937313117));
#46477=CARTESIAN_POINT('Ctrl Pts',(-25.2068558587201,2.01496526840376,3.6278897925597));
#46478=CARTESIAN_POINT('Ctrl Pts',(-25.1405968498901,0.608177203104113,
4.10487909715074));
#46479=CARTESIAN_POINT('Ctrl Pts',(-25.0743378410601,-0.67637689196117,
3.88097217602644));
#46480=CARTESIAN_POINT('Ctrl Pts',(-25.0080788322301,-1.96093098702646,
3.65706525490214));
#46481=CARTESIAN_POINT('Ctrl Pts',(-24.9418198234001,-3.12325111185738,
2.73226210806249));
#46482=CARTESIAN_POINT('Ctrl Pts',(-24.8755608145702,-3.62991379199177,
1.53086062077391));
#46483=CARTESIAN_POINT('Ctrl Pts',(-24.8490950503918,-3.83228951790751,
1.0509861251));
#46484=CARTESIAN_POINT('Ctrl Pts',(-24.8226292862134,-3.93005938637917,
0.526982173100531));
#46485=CARTESIAN_POINT('Ctrl Pts',(-24.796163522035,-3.92757907140906,0.00208605505030474));
#46486=CARTESIAN_POINT('Origin',(-20.1,0.,0.));
#46487=CARTESIAN_POINT('',(-23.362836477965,-3.92954087356332,-0.00313358730535757));
#46488=CARTESIAN_POINT('',(-23.546163522035,-3.93003375797999,-0.00328548955642192));
#46489=CARTESIAN_POINT('',(-20.1,-3.933,-4.81653586104654E-16));
#46490=CARTESIAN_POINT('Ctrl Pts',(-23.362836477965,-3.92954087356332,-0.00313358730535757));
#46491=CARTESIAN_POINT('Ctrl Pts',(-23.4074345202608,-3.92297089886225,
0.880266467358495));
#46492=CARTESIAN_POINT('Ctrl Pts',(-23.4520325625565,-3.62843124950771,
1.76763631385351));
#46493=CARTESIAN_POINT('Ctrl Pts',(-23.4966306048523,-3.0816991297842,2.45416793101582));
#46494=CARTESIAN_POINT('Ctrl Pts',(-23.5628896136823,-2.26942292922431,
3.47414329634622));
#46495=CARTESIAN_POINT('Ctrl Pts',(-23.6291486225123,-0.900486241088972,
4.05081158553528));
#46496=CARTESIAN_POINT('Ctrl Pts',(-23.6954076313422,0.39677869711984,3.91948657984679));
#46497=CARTESIAN_POINT('Ctrl Pts',(-23.7616666401722,1.69404363532865,3.78816157415829));
#46498=CARTESIAN_POINT('Ctrl Pts',(-23.8279256490022,2.91963682361093,2.94884327359225));
#46499=CARTESIAN_POINT('Ctrl Pts',(-23.8941846578322,3.51101935415754,1.78677195511959));
#46500=CARTESIAN_POINT('Ctrl Pts',(-23.9604436666622,4.10240188470415,0.624700636646922));
#46501=CARTESIAN_POINT('Ctrl Pts',(-24.0267026754922,4.05957375751508,-0.860123699732376));
#46502=CARTESIAN_POINT('Ctrl Pts',(-24.0929616843222,3.40219320868621,-1.98617525416531));
#46503=CARTESIAN_POINT('Ctrl Pts',(-24.1592206931522,2.74481265985733,-3.11222680859825));
#46504=CARTESIAN_POINT('Ctrl Pts',(-24.2254797019822,1.47287968938866,-3.87950558108483));
#46505=CARTESIAN_POINT('Ctrl Pts',(-24.2917387108122,0.170201795278273,
-3.93583954010648));
#46506=CARTESIAN_POINT('Ctrl Pts',(-24.3579977196422,-1.13247609883211,
-3.99217349912814));
#46507=CARTESIAN_POINT('Ctrl Pts',(-24.4242567284722,-2.46589891658421,
-3.33756264468487));
#46508=CARTESIAN_POINT('Ctrl Pts',(-24.4905157373022,-3.21803332339699,
-2.27246188703126));
#46509=CARTESIAN_POINT('Ctrl Pts',(-24.5312893175231,-3.68087170740913,
-1.6170344673876));
#46510=CARTESIAN_POINT('Ctrl Pts',(-24.5720628977441,-3.92359009889234,
-0.806164357459004));
#46511=CARTESIAN_POINT('Ctrl Pts',(-24.612836477965,-3.92791610626173,0.00232109521066254));
#46512=CARTESIAN_POINT('Ctrl Pts',(-24.796163522035,-3.92757907140906,0.00208605505030474));
#46513=CARTESIAN_POINT('Ctrl Pts',(-24.7563702773834,-3.92384973339512,
-0.78713429398102));
#46514=CARTESIAN_POINT('Ctrl Pts',(-24.7165770327318,-3.69348120864786,
-1.57837159481464));
#46515=CARTESIAN_POINT('Ctrl Pts',(-24.6767837880802,-3.25127923682329,
-2.22465431953071));
#46516=CARTESIAN_POINT('Ctrl Pts',(-24.6105247792502,-2.51497676608259,
-3.30076794480929));
#46517=CARTESIAN_POINT('Ctrl Pts',(-24.5442657704202,-1.19136658916336,
-3.97499536762895));
#46518=CARTESIAN_POINT('Ctrl Pts',(-24.4780067615902,0.112003991582728,
-3.93791887508927));
#46519=CARTESIAN_POINT('Ctrl Pts',(-24.4117477527602,1.41537457232881,-3.9008423825496));
#46520=CARTESIAN_POINT('Ctrl Pts',(-24.3454887439302,2.69850555690174,-3.15246197465059));
#46521=CARTESIAN_POINT('Ctrl Pts',(-24.2792297351002,3.37245887007014,-2.03625428556874));
#46522=CARTESIAN_POINT('Ctrl Pts',(-24.2129707262702,4.04641218323854,-0.920046596486897));
#46523=CARTESIAN_POINT('Ctrl Pts',(-24.1467117174402,4.11118782500241,0.563988373777779));
#46524=CARTESIAN_POINT('Ctrl Pts',(-24.0804527086102,3.53704904185838,1.73467621447729));
#46525=CARTESIAN_POINT('Ctrl Pts',(-24.0141936997803,2.96291025871434,2.90536405517679));
#46526=CARTESIAN_POINT('Ctrl Pts',(-23.9479346909503,1.7498570506624,3.76270476631113));
#46527=CARTESIAN_POINT('Ctrl Pts',(-23.8816756821203,0.454675018478186,
3.91319154529663));
#46528=CARTESIAN_POINT('Ctrl Pts',(-23.8154166732903,-0.840507013706024,
4.06367832428214));
#46529=CARTESIAN_POINT('Ctrl Pts',(-23.7491576644603,-2.21781787002251,
3.50731117111882));
#46530=CARTESIAN_POINT('Ctrl Pts',(-23.6828986556303,-3.04508289517983,
2.4994553191023));
#46531=CARTESIAN_POINT('Ctrl Pts',(-23.6373202777652,-3.61414359465313,
1.80616944495611));
#46532=CARTESIAN_POINT('Ctrl Pts',(-23.5917418999001,-3.92293272121378,
0.899247420609198));
#46533=CARTESIAN_POINT('Ctrl Pts',(-23.546163522035,-3.93003375797999,-0.00328548955642192));
#46534=CARTESIAN_POINT('Origin',(-20.1,0.,0.));
#46535=CARTESIAN_POINT('',(-22.112836477965,-3.93925214816407,-0.000930796536843803));
#46536=CARTESIAN_POINT('',(-22.296163522035,-3.93941472965677,-0.000577549300834287));
#46537=CARTESIAN_POINT('',(-20.1,-3.933,-4.81653586104654E-16));
#46538=CARTESIAN_POINT('Ctrl Pts',(-22.112836477965,-3.93925214816407,-0.000930796536843803));
#46539=CARTESIAN_POINT('Ctrl Pts',(-22.1765471339475,-3.93525732598551,
1.25304394614318));
#46540=CARTESIAN_POINT('Ctrl Pts',(-22.24025778993,-3.28460955709606,2.51058367703939));
#46541=CARTESIAN_POINT('Ctrl Pts',(-22.3039684459124,-2.25702327318862,
3.22887835952372));
#46542=CARTESIAN_POINT('Ctrl Pts',(-22.3702274547424,-1.18833472165735,
3.97590400186476));
#46543=CARTESIAN_POINT('Ctrl Pts',(-22.4364864635724,0.288049624548706,
4.13968349190898));
#46544=CARTESIAN_POINT('Ctrl Pts',(-22.5027454724024,1.49447969449625,3.6450432001131));
#46545=CARTESIAN_POINT('Ctrl Pts',(-22.5690044812324,2.70090976444378,3.15040290831721));
#46546=CARTESIAN_POINT('Ctrl Pts',(-22.6352634900624,3.63738555813281,1.99734283468122));
#46547=CARTESIAN_POINT('Ctrl Pts',(-22.7015224988924,3.8740712420106,0.715109458270375));
#46548=CARTESIAN_POINT('Ctrl Pts',(-22.7677815077224,4.11075692588839,-0.567123918140469));
#46549=CARTESIAN_POINT('Ctrl Pts',(-22.8340405165524,3.64765249995493,-1.97853059732616));
#46550=CARTESIAN_POINT('Ctrl Pts',(-22.9002995253823,2.69731965973127,-2.87128476585916));
#46551=CARTESIAN_POINT('Ctrl Pts',(-22.9665585342123,1.74698681950761,-3.76403893439215));
#46552=CARTESIAN_POINT('Ctrl Pts',(-23.0328175430423,0.30942556499374,-4.13814059227245));
#46553=CARTESIAN_POINT('Ctrl Pts',(-23.0990765518723,-0.955533573395335,
-3.82187976573015));
#46554=CARTESIAN_POINT('Ctrl Pts',(-23.1653355607023,-2.22049271178442,
-3.50561893918785));
#46555=CARTESIAN_POINT('Ctrl Pts',(-23.2315945695323,-3.31284973404871,
-2.49899562822293));
#46556=CARTESIAN_POINT('Ctrl Pts',(-23.2978535783623,-3.73122038868862,
-1.26404275200461));
#46557=CARTESIAN_POINT('Ctrl Pts',(-23.3195145448965,-3.86799141664524,
-0.860319946676077));
#46558=CARTESIAN_POINT('Ctrl Pts',(-23.3411755114308,-3.93273186569672,
-0.432194999766649));
#46559=CARTESIAN_POINT('Ctrl Pts',(-23.362836477965,-3.92954087356332,-0.00313358730535757));
#46560=CARTESIAN_POINT('Ctrl Pts',(-23.546163522035,-3.93003375797999,-0.00328548955642192));
#46561=CARTESIAN_POINT('Ctrl Pts',(-23.5254828910701,-3.93325576647851,
-0.412798748322419));
#46562=CARTESIAN_POINT('Ctrl Pts',(-23.5048022601052,-3.87436684872067,
-0.821408385246961));
#46563=CARTESIAN_POINT('Ctrl Pts',(-23.4841216291403,-3.74949809732583,
-1.20874765734832));
#46564=CARTESIAN_POINT('Ctrl Pts',(-23.4178626203103,-3.34942908031632,
-2.44975023091271));
#46565=CARTESIAN_POINT('Ctrl Pts',(-23.3516036114803,-2.27207185229914,
-3.47241082717177));
#46566=CARTESIAN_POINT('Ctrl Pts',(-23.2853446026503,-1.01192620125752,
-3.80733629848171));
#46567=CARTESIAN_POINT('Ctrl Pts',(-23.2190855938203,0.248219449784087,
-4.14226176979165));
#46568=CARTESIAN_POINT('Ctrl Pts',(-23.1528265849903,1.69115352385012,-3.78945211615245));
#46569=CARTESIAN_POINT('Ctrl Pts',(-23.0865675761603,2.65457957778525,-2.91084403176621));
#46570=CARTESIAN_POINT('Ctrl Pts',(-23.0203085673304,3.61800563172037,-2.03223594737998));
#46571=CARTESIAN_POINT('Ctrl Pts',(-22.9540495585004,4.10192366552458,-0.627829432246697));
#46572=CARTESIAN_POINT('Ctrl Pts',(-22.8877905496704,3.88421859382125,0.657762520794241));
#46573=CARTESIAN_POINT('Ctrl Pts',(-22.8215315408404,3.66651352211792,1.94335447383518));
#46574=CARTESIAN_POINT('Ctrl Pts',(-22.7552725320104,2.74718534490704,3.11013186478378));
#46575=CARTESIAN_POINT('Ctrl Pts',(-22.6890135231804,1.54819930612708,3.62255216810003));
#46576=CARTESIAN_POINT('Ctrl Pts',(-22.6227545143504,0.349213267347125,
4.13497247141627));
#46577=CARTESIAN_POINT('Ctrl Pts',(-22.5564955055204,-1.12943063300191,
3.99303568710015));
#46578=CARTESIAN_POINT('Ctrl Pts',(-22.4902364966904,-2.20904522830817,
3.26188974105464));
#46579=CARTESIAN_POINT('Ctrl Pts',(-22.4255455051386,-3.26311077950542,
2.54804633992363));
#46580=CARTESIAN_POINT('Ctrl Pts',(-22.3608545135868,-3.93680958792955,
1.27255103296312));
#46581=CARTESIAN_POINT('Ctrl Pts',(-22.296163522035,-3.93941472965677,-0.000577549300834287));
#46582=CARTESIAN_POINT('Origin',(-20.1,0.,0.));
#46583=CARTESIAN_POINT('',(-20.862836477965,-3.93234356276048,0.00362164229294471));
#46584=CARTESIAN_POINT('',(-21.046163522035,-3.9317665782605,0.00358829654485505));
#46585=CARTESIAN_POINT('',(-20.1,-3.933,-4.81653586104654E-16));
#46586=CARTESIAN_POINT('Ctrl Pts',(-20.862836477965,-3.93234356276048,0.0036216422929447));
#46587=CARTESIAN_POINT('Ctrl Pts',(-20.8794007388042,-3.93531979599253,
0.331135104398647));
#46588=CARTESIAN_POINT('Ctrl Pts',(-20.8959649996434,-3.89783641446075,
0.657976746908121));
#46589=CARTESIAN_POINT('Ctrl Pts',(-20.9125292604826,-3.81726008563346,
0.973824906028897));
#46590=CARTESIAN_POINT('Ctrl Pts',(-20.9787882693126,-3.49494520934099,
2.23725502025529));
#46591=CARTESIAN_POINT('Ctrl Pts',(-21.0450472781426,-2.48310226931282,
3.32477896443637));
#46592=CARTESIAN_POINT('Ctrl Pts',(-21.1113062869725,-1.2461600872343,3.73723086604704));
#46593=CARTESIAN_POINT('Ctrl Pts',(-21.1775652958025,-0.00921790515579238,
4.1496827676577));
#46594=CARTESIAN_POINT('Ctrl Pts',(-21.2438243046325,1.45282351897305,3.88706262669794));
#46595=CARTESIAN_POINT('Ctrl Pts',(-21.3100833134625,2.46889741289712,3.06991124842487));
#46596=CARTESIAN_POINT('Ctrl Pts',(-21.3763423222925,3.48497130682118,2.2527598701518));
#46597=CARTESIAN_POINT('Ctrl Pts',(-21.4426013311225,4.05507767054045,0.881077254565418));
#46598=CARTESIAN_POINT('Ctrl Pts',(-21.5088603399525,3.91754167653988,-0.415543886543193));
#46599=CARTESIAN_POINT('Ctrl Pts',(-21.5751193487825,3.78000568253931,-1.7121650276518));
#46600=CARTESIAN_POINT('Ctrl Pts',(-21.6413783576125,2.93482733081889,-2.93372469428265));
#46601=CARTESIAN_POINT('Ctrl Pts',(-21.7076373664425,1.76993756462108,-3.51953555564859));
#46602=CARTESIAN_POINT('Ctrl Pts',(-21.7738963752725,0.605047798423272,
-4.10534641701454));
#46603=CARTESIAN_POINT('Ctrl Pts',(-21.8401553841025,-0.879553382251932,
-4.05540847311559));
#46604=CARTESIAN_POINT('Ctrl Pts',(-21.9064143929325,-2.00244443517383,
-3.39264289164551));
#46605=CARTESIAN_POINT('Ctrl Pts',(-21.9726734017624,-3.12533548809572,
-2.72987731017544));
#46606=CARTESIAN_POINT('Ctrl Pts',(-22.0389324105924,-3.8865164132643,-1.45428409113424));
#46607=CARTESIAN_POINT('Ctrl Pts',(-22.1051914194224,-3.93661049742035,
-0.151351584294707));
#46608=CARTESIAN_POINT('Ctrl Pts',(-22.10773977227,-3.93853713961222,-0.101240183255385));
#46609=CARTESIAN_POINT('Ctrl Pts',(-22.1102881251175,-3.93941193644936,
-0.0510883417224217));
#46610=CARTESIAN_POINT('Ctrl Pts',(-22.112836477965,-3.93925214816407,-0.000930796536843803));
#46611=CARTESIAN_POINT('Ctrl Pts',(-22.296163522035,-3.93941472965677,-0.000577549300834287));
#46612=CARTESIAN_POINT('Ctrl Pts',(-22.2945955047568,-3.93947787457297,
-0.0314363685343833));
#46613=CARTESIAN_POINT('Ctrl Pts',(-22.2930274874786,-3.93914674633027,
-0.0622937972973192));
#46614=CARTESIAN_POINT('Ctrl Pts',(-22.2914594702004,-3.93841720487129,
-0.0931418037587124));
#46615=CARTESIAN_POINT('Ctrl Pts',(-22.2252004613704,-3.90758929586465,
-1.39667229475164));
#46616=CARTESIAN_POINT('Ctrl Pts',(-22.1589414525405,-3.16534818758786,
-2.68337816896259));
#46617=CARTESIAN_POINT('Ctrl Pts',(-22.0926824437105,-2.05237735636058,
-3.36267046029439));
#46618=CARTESIAN_POINT('Ctrl Pts',(-22.0264234348805,-0.939406525133289,
-4.04196275162618));
#46619=CARTESIAN_POINT('Ctrl Pts',(-21.9601644260505,0.544294029044505,
-4.11384146007883));
#46620=CARTESIAN_POINT('Ctrl Pts',(-21.8939054172205,1.71771614846726,-3.54531475321241));
#46621=CARTESIAN_POINT('Ctrl Pts',(-21.8276464083905,2.89113826789002,-2.97678804634599));
#46622=CARTESIAN_POINT('Ctrl Pts',(-21.7613873995605,3.75428195255775,-1.76785592416049));
#46623=CARTESIAN_POINT('Ctrl Pts',(-21.6951283907305,3.91097029556221,-0.473409766869109));
#46624=CARTESIAN_POINT('Ctrl Pts',(-21.6288693819005,4.06765863856667,0.821036390422279));
#46625=CARTESIAN_POINT('Ctrl Pts',(-21.5626103730705,3.51789163990787,2.20099658281955));
#46626=CARTESIAN_POINT('Ctrl Pts',(-21.4963513642405,2.51400850188269,3.03307875075606));
#46627=CARTESIAN_POINT('Ctrl Pts',(-21.4300923554105,1.51012536385751,3.86516091869257));
#46628=CARTESIAN_POINT('Ctrl Pts',(-21.3638333465805,0.0521260864659473,
4.14936506216831));
#46629=CARTESIAN_POINT('Ctrl Pts',(-21.2975743377506,-1.19077787552372,
3.75524346893355));
#46630=CARTESIAN_POINT('Ctrl Pts',(-21.2313153289206,-2.43368183751338,
3.36112187569878));
#46631=CARTESIAN_POINT('Ctrl Pts',(-21.1650563200905,-3.46149048410115,
2.28867454575351));
#46632=CARTESIAN_POINT('Ctrl Pts',(-21.0987973112606,-3.80244684589627,
1.03014729183));
#46633=CARTESIAN_POINT('Ctrl Pts',(-21.081252714852,-3.89272802978727,0.696904263763043));
#46634=CARTESIAN_POINT('Ctrl Pts',(-21.0637081184435,-3.93485212301176,
0.350614663720363));
#46635=CARTESIAN_POINT('Ctrl Pts',(-21.046163522035,-3.9317665782605,0.00358829654485505));
#46636=CARTESIAN_POINT('Origin',(-20.1,0.,0.));
#46637=CARTESIAN_POINT('',(-19.612836477965,-3.92668363390084,-0.000828347603293866));
#46638=CARTESIAN_POINT('',(-19.796163522035,-3.92682791432394,-0.00113809054688487));
#46639=CARTESIAN_POINT('',(-20.1,-3.933,-4.81653586104654E-16));
#46640=CARTESIAN_POINT('Ctrl Pts',(-19.612836477965,-3.92668363390084,-0.000828347603293866));
#46641=CARTESIAN_POINT('Ctrl Pts',(-19.6485133524909,-3.92535470355143,
0.707150422160364));
#46642=CARTESIAN_POINT('Ctrl Pts',(-19.6841902270168,-3.7427691911929,1.41576831419161));
#46643=CARTESIAN_POINT('Ctrl Pts',(-19.7198671015427,-3.38301464948758,
2.01866822195352));
#46644=CARTESIAN_POINT('Ctrl Pts',(-19.7861261103727,-2.71487934693509,
3.13837253582242));
#46645=CARTESIAN_POINT('Ctrl Pts',(-19.8523851192027,-1.43565559653748,
3.89343614948163));
#46646=CARTESIAN_POINT('Ctrl Pts',(-19.9186441280327,-0.132498138932822,
3.93729015340666));
#46647=CARTESIAN_POINT('Ctrl Pts',(-19.9849031368627,1.17065931867184,3.98114415733169));
#46648=CARTESIAN_POINT('Ctrl Pts',(-20.0511621456927,2.49775048348358,3.31378855152255));
#46649=CARTESIAN_POINT('Ctrl Pts',(-20.1174211545226,3.23964980691583,2.24153488430273));
#46650=CARTESIAN_POINT('Ctrl Pts',(-20.1836801633526,3.98154913034808,1.1692812170829));
#46651=CARTESIAN_POINT('Ctrl Pts',(-20.2499391721826,4.13825661240085,-0.307870511547617));
#46652=CARTESIAN_POINT('Ctrl Pts',(-20.3161981810126,3.63784461652941,-1.51191800536888));
#46653=CARTESIAN_POINT('Ctrl Pts',(-20.3824571898426,3.13743262065797,-2.71596549919015));
#46654=CARTESIAN_POINT('Ctrl Pts',(-20.4487161986726,1.97990114686232,-3.64690875820217));
#46655=CARTESIAN_POINT('Ctrl Pts',(-20.5149752075026,0.696549033280147,
-3.8774513476293));
#46656=CARTESIAN_POINT('Ctrl Pts',(-20.5812342163326,-0.586803080302027,
-4.10799393705643));
#46657=CARTESIAN_POINT('Ctrl Pts',(-20.6474932251626,-1.99597583367073,
-3.63813585689868));
#46658=CARTESIAN_POINT('Ctrl Pts',(-20.7137522339926,-2.8841688040767,-2.68353867468395));
#46659=CARTESIAN_POINT('Ctrl Pts',(-20.7634469819834,-3.55032011860643,
-1.96758370885252));
#46660=CARTESIAN_POINT('Ctrl Pts',(-20.8131417299742,-3.92341450991201,
-0.97895760594279));
#46661=CARTESIAN_POINT('Ctrl Pts',(-20.862836477965,-3.93234356276048,0.0036216422929447));
#46662=CARTESIAN_POINT('Ctrl Pts',(-21.046163522035,-3.9317665782605,0.00358829654485505));
#46663=CARTESIAN_POINT('Ctrl Pts',(-20.9974491096135,-3.92319923957353,
-0.959966816269948));
#46664=CARTESIAN_POINT('Ctrl Pts',(-20.9487346971921,-3.56608662401112,
-1.92920206092837));
#46665=CARTESIAN_POINT('Ctrl Pts',(-20.9000202847706,-2.92352288274049,
-2.6406096667939));
#46666=CARTESIAN_POINT('Ctrl Pts',(-20.8337612759406,-2.0495384807871,-3.60823219359254));
#46667=CARTESIAN_POINT('Ctrl Pts',(-20.7675022671106,-0.64746559987786,
-4.09887006928808));
#46668=CARTESIAN_POINT('Ctrl Pts',(-20.7012432582806,0.639154129026382,
-3.88732394561629));
#46669=CARTESIAN_POINT('Ctrl Pts',(-20.6349842494506,1.92577385793062,-3.6757778219445));
#46670=CARTESIAN_POINT('Ctrl Pts',(-20.5687252406206,3.09694043482986,-2.7620476989054));
#46671=CARTESIAN_POINT('Ctrl Pts',(-20.5024662317906,3.61509660473914,-1.56552930251614));
#46672=CARTESIAN_POINT('Ctrl Pts',(-20.4362072229606,4.13325277464841,-0.369010906126889));
#46673=CARTESIAN_POINT('Ctrl Pts',(-20.3699482141306,3.99839853756772,1.11029576361251));
#46674=CARTESIAN_POINT('Ctrl Pts',(-20.3036892053006,3.27243104370014,2.19339930765503));
#46675=CARTESIAN_POINT('Ctrl Pts',(-20.2374301964706,2.54646354983257,3.27650285169755));
#46676=CARTESIAN_POINT('Ctrl Pts',(-20.1711711876407,1.2293827991781,3.96340327004319));
#46677=CARTESIAN_POINT('Ctrl Pts',(-20.1049121788107,-0.074280369672471,
3.93881808228536));
#46678=CARTESIAN_POINT('Ctrl Pts',(-20.0386531699807,-1.37794353852305,
3.91423289452753));
#46679=CARTESIAN_POINT('Ctrl Pts',(-19.9723941611507,-2.66818912556973,
3.17816210066622));
#46680=CARTESIAN_POINT('Ctrl Pts',(-19.9061351523207,-3.35280344433398,
2.06845703902532));
#46681=CARTESIAN_POINT('Ctrl Pts',(-19.8694779422255,-3.73156025582722,
1.45452253703641));
#46682=CARTESIAN_POINT('Ctrl Pts',(-19.8328207321302,-3.92494801200659,
0.726227639740267));
#46683=CARTESIAN_POINT('Ctrl Pts',(-19.796163522035,-3.92682791432394,-0.00113809054688487));
#46684=CARTESIAN_POINT('Origin',(-20.1,0.,0.));
#46685=CARTESIAN_POINT('',(-18.362836477965,-3.93539198680633,-0.00329798213515642));
#46686=CARTESIAN_POINT('',(-18.546163522035,-3.93595275298544,-0.00314060659151173));
#46687=CARTESIAN_POINT('',(-20.1,-3.933,-4.81653586104654E-16));
#46688=CARTESIAN_POINT('Ctrl Pts',(-18.362836477965,-3.93539198680633,-0.00329798213515642));
#46689=CARTESIAN_POINT('Ctrl Pts',(-18.4176259661776,-3.9256864189977,1.07786343746756));
#46690=CARTESIAN_POINT('Ctrl Pts',(-18.4724154543902,-3.46255938905757,
2.1663295974234));
#46691=CARTESIAN_POINT('Ctrl Pts',(-18.5272049426028,-2.6696961456285,2.89698671044328));
#46692=CARTESIAN_POINT('Ctrl Pts',(-18.5934639514328,-1.71085651486767,
3.78059810530474));
#46693=CARTESIAN_POINT('Ctrl Pts',(-18.6597229602628,-0.269778218465152,
4.1409143621431));
#46694=CARTESIAN_POINT('Ctrl Pts',(-18.7259819690928,0.992093901389918,
3.8125528451441));
#46695=CARTESIAN_POINT('Ctrl Pts',(-18.7922409779228,2.25396602124499,3.48419132814511));
#46696=CARTESIAN_POINT('Ctrl Pts',(-18.8584999867528,3.33663196455261,2.46715203730877));
#46697=CARTESIAN_POINT('Ctrl Pts',(-18.9247589955828,3.74315564656476,1.22824888183212));
#46698=CARTESIAN_POINT('Ctrl Pts',(-18.9910180044128,4.14967932857691,-0.0106542736445235));
#46699=CARTESIAN_POINT('Ctrl Pts',(-19.0572770132428,3.88006074929359,-1.47142129376147));
#46700=CARTESIAN_POINT('Ctrl Pts',(-19.1235360220728,3.05805294831981,-2.48357034817677));
#46701=CARTESIAN_POINT('Ctrl Pts',(-19.1897950309028,2.23604514734603,-3.49571940259206));
#46702=CARTESIAN_POINT('Ctrl Pts',(-19.2560540397328,0.861648124681792,
-4.0592504913057));
#46703=CARTESIAN_POINT('Ctrl Pts',(-19.3223130485627,-0.434299513895741,
-3.91550679233807));
#46704=CARTESIAN_POINT('Ctrl Pts',(-19.3885720573927,-1.73024715247327,
-3.77176309337043));
#46705=CARTESIAN_POINT('Ctrl Pts',(-19.4548310662227,-2.9477454069641,-2.92074460672151));
#46706=CARTESIAN_POINT('Ctrl Pts',(-19.5210900750527,-3.5279711068558,-1.75306285635774));
#46707=CARTESIAN_POINT('Ctrl Pts',(-19.5516722093568,-3.79577680745584,
-1.21411425533504));
#46708=CARTESIAN_POINT('Ctrl Pts',(-19.5822543436609,-3.92782278992184,
-0.607706111115191));
#46709=CARTESIAN_POINT('Ctrl Pts',(-19.612836477965,-3.92668363390084,-0.000828347603293866));
#46710=CARTESIAN_POINT('Ctrl Pts',(-19.796163522035,-3.92682791432394,-0.00113809054688487));
#46711=CARTESIAN_POINT('Ctrl Pts',(-19.7665617233002,-3.92834599193799,
-0.588507775762331));
#46712=CARTESIAN_POINT('Ctrl Pts',(-19.7369599245655,-3.80498088204029,
-1.17527154672688));
#46713=CARTESIAN_POINT('Ctrl Pts',(-19.7073581258307,-3.55349992886683,
-1.70071858759768));
#46714=CARTESIAN_POINT('Ctrl Pts',(-19.6410991170007,-2.9905990441536,-2.87684982315929));
#46715=CARTESIAN_POINT('Ctrl Pts',(-19.5748401081707,-1.78581422424533,
-3.74577296486201));
#46716=CARTESIAN_POINT('Ctrl Pts',(-19.5085810993407,-0.492133262158209,
-3.90865837735552));
#46717=CARTESIAN_POINT('Ctrl Pts',(-19.4423220905107,0.801547699928912,
-4.07154378984904));
#46718=CARTESIAN_POINT('Ctrl Pts',(-19.3760630816808,2.18412480419487,-3.52839147313334));
#46719=CARTESIAN_POINT('Ctrl Pts',(-19.3098040728508,3.02100484455689,-2.52850453584661));
#46720=CARTESIAN_POINT('Ctrl Pts',(-19.2435450640208,3.8578848849189,-1.52861759855989));
#46721=CARTESIAN_POINT('Ctrl Pts',(-19.1772860551908,4.14906786137697,-0.0719960407021211));
#46722=CARTESIAN_POINT('Ctrl Pts',(-19.1110270463608,3.76090282736967,1.17278104601673));
#46723=CARTESIAN_POINT('Ctrl Pts',(-19.0447680375308,3.37273779336236,2.4175581327356));
#46724=CARTESIAN_POINT('Ctrl Pts',(-18.9785090287008,2.3052247488897,3.45049074831555));
#46725=CARTESIAN_POINT('Ctrl Pts',(-18.9122500198708,1.04834470371331,3.79747005787655));
#46726=CARTESIAN_POINT('Ctrl Pts',(-18.8459910110408,-0.208535341463058,
4.14444936743754));
#46727=CARTESIAN_POINT('Ctrl Pts',(-18.7797320022108,-1.65478238734316,
3.80547537097956));
#46728=CARTESIAN_POINT('Ctrl Pts',(-18.7134729933808,-2.62657917083836,
2.93613475815557));
#46729=CARTESIAN_POINT('Ctrl Pts',(-18.6577031695989,-3.44453489224753,
2.20441580189885));
#46730=CARTESIAN_POINT('Ctrl Pts',(-18.6019333458169,-3.92636673554791,
1.0969590749087));
#46731=CARTESIAN_POINT('Ctrl Pts',(-18.546163522035,-3.93595275298544,-0.00314060659151173));
#46732=CARTESIAN_POINT('Origin',(-20.1,0.,0.));
#46733=CARTESIAN_POINT('',(-17.112836477965,-3.93744710033063,0.002522420057968));
#46734=CARTESIAN_POINT('',(-17.296163522035,-3.93695989693636,0.00276125700748165));
#46735=CARTESIAN_POINT('',(-20.1,-3.933,-4.81653586104654E-16));
#46736=CARTESIAN_POINT('Ctrl Pts',(-17.112836477965,-3.93744710033063,0.002522420057968));
#46737=CARTESIAN_POINT('Ctrl Pts',(-17.1204795710344,-3.93856978775161,
0.153138791280183));
#46738=CARTESIAN_POINT('Ctrl Pts',(-17.1281226641037,-3.93067892709947,
0.303636406391696));
#46739=CARTESIAN_POINT('Ctrl Pts',(-17.135765757173,-3.913382153674,0.453045118553371));
#46740=CARTESIAN_POINT('Ctrl Pts',(-17.202024766003,-3.76343408255482,1.74828947690608));
#46741=CARTESIAN_POINT('Ctrl Pts',(-17.268283774833,-2.90659489979499,2.96169852217127));
#46742=CARTESIAN_POINT('Ctrl Pts',(-17.334542783663,-1.73614792488526,3.5363257840275));
#46743=CARTESIAN_POINT('Ctrl Pts',(-17.4008017924929,-0.565700949975524,
4.11095304588373));
#46744=CARTESIAN_POINT('Ctrl Pts',(-17.467060801323,0.918353817084128,4.04679852433096));
#46745=CARTESIAN_POINT('Ctrl Pts',(-17.5333198101529,2.03484570423632,3.37330880791163));
#46746=CARTESIAN_POINT('Ctrl Pts',(-17.5995788189829,3.15133759138853,2.6998190914923));
#46747=CARTESIAN_POINT('Ctrl Pts',(-17.6658378278129,3.90026659863329,1.41699418020642));
#46748=CARTESIAN_POINT('Ctrl Pts',(-17.7320968366429,3.93787952146319,0.113641664316406));
#46749=CARTESIAN_POINT('Ctrl Pts',(-17.7983558454729,3.97549244429308,-1.18971085157359));
#46750=CARTESIAN_POINT('Ctrl Pts',(-17.8646148543029,3.30178928270808,-2.51359097206773));
#46751=CARTESIAN_POINT('Ctrl Pts',(-17.9308738631329,2.22599508740998,-3.25034696552659));
#46752=CARTESIAN_POINT('Ctrl Pts',(-17.9971328719629,1.15020089211187,-3.98710295898546));
#46753=CARTESIAN_POINT('Ctrl Pts',(-18.0633918807929,-0.327684336899324,
-4.13673482540907));
#46754=CARTESIAN_POINT('Ctrl Pts',(-18.1296508896229,-1.52932164152444,
-3.63056260167998));
#46755=CARTESIAN_POINT('Ctrl Pts',(-18.1959098984529,-2.73095894614955,
-3.1243903779509));
#46756=CARTESIAN_POINT('Ctrl Pts',(-18.2621689072829,-3.65634832638855,
-1.96241406406912));
#46757=CARTESIAN_POINT('Ctrl Pts',(-18.3284279161129,-3.8807425339485,-0.677972640685939));
#46758=CARTESIAN_POINT('Ctrl Pts',(-18.3398974367302,-3.91958546316641,
-0.455634159512376));
#46759=CARTESIAN_POINT('Ctrl Pts',(-18.3513669573476,-3.93742373073598,
-0.229626126408842));
#46760=CARTESIAN_POINT('Ctrl Pts',(-18.362836477965,-3.93539198680633,-0.00329798213515642));
#46761=CARTESIAN_POINT('Ctrl Pts',(-18.546163522035,-3.93595275298544,-0.00314060659151173));
#46762=CARTESIAN_POINT('Ctrl Pts',(-18.5356743369869,-3.93775569055916,
-0.210047287445732));
#46763=CARTESIAN_POINT('Ctrl Pts',(-18.5251851519389,-3.92285337434481,
-0.4166937197063));
#46764=CARTESIAN_POINT('Ctrl Pts',(-18.5146959668909,-3.89034016437652,
-0.62053111545171));
#46765=CARTESIAN_POINT('Ctrl Pts',(-18.4484369580609,-3.68495785330915,
-1.90814914704498));
#46766=CARTESIAN_POINT('Ctrl Pts',(-18.3821779492309,-2.7768467100641,-3.08367798104153));
#46767=CARTESIAN_POINT('Ctrl Pts',(-18.3159189404009,-1.58282338906351,
-3.60755811801555));
#46768=CARTESIAN_POINT('Ctrl Pts',(-18.2496599315709,-0.388800068062912,
-4.13143825498958));
#46769=CARTESIAN_POINT('Ctrl Pts',(-18.1834009227409,1.09113543069324,-4.00366969494108));
#46770=CARTESIAN_POINT('Ctrl Pts',(-18.1171419139109,2.17770308165872,-3.28289731004049));
#46771=CARTESIAN_POINT('Ctrl Pts',(-18.0508829050809,3.2642707326242,-2.56212492513991));
#46772=CARTESIAN_POINT('Ctrl Pts',(-17.9846238962509,3.95747053579902,-1.24834871538727));
#46773=CARTESIAN_POINT('Ctrl Pts',(-17.9183648874209,3.93912863407312,0.0554172380767894));
#46774=CARTESIAN_POINT('Ctrl Pts',(-17.8521058785909,3.92078673234721,1.35918319154085));
#46775=CARTESIAN_POINT('Ctrl Pts',(-17.7858468697609,3.19090312572055,2.65293888871631));
#46776=CARTESIAN_POINT('Ctrl Pts',(-17.7195878609309,2.08448928314013,3.34285953427781));
#46777=CARTESIAN_POINT('Ctrl Pts',(-17.6533288521009,0.978075440559705,
4.0327801798393));
#46778=CARTESIAN_POINT('Ctrl Pts',(-17.587069843271,-0.504868637974483,
4.11886577378683));
#46779=CARTESIAN_POINT('Ctrl Pts',(-17.520810834441,-1.68368202029562,3.5616036177215));
#46780=CARTESIAN_POINT('Ctrl Pts',(-17.454551825611,-2.86249540261677,3.00434146165616));
#46781=CARTESIAN_POINT('Ctrl Pts',(-17.388292816781,-3.73717808872487,1.80373155557796));
#46782=CARTESIAN_POINT('Ctrl Pts',(-17.322033807951,-3.90625682929457,0.510845463029787));
#46783=CARTESIAN_POINT('Ctrl Pts',(-17.3134103793123,-3.92826196458659,
0.34257987690214));
#46784=CARTESIAN_POINT('Ctrl Pts',(-17.3047869506736,-3.93831536149175,
0.172751288119817));
#46785=CARTESIAN_POINT('Ctrl Pts',(-17.296163522035,-3.93695989693636,0.00276125700748165));
#46786=CARTESIAN_POINT('Origin',(-20.1,0.,0.));
#46787=CARTESIAN_POINT('',(-15.862836477965,-3.92749965338984,0.00198301116285243));
#46788=CARTESIAN_POINT('',(-16.046163522035,-3.92722756002595,0.00170206837946952));
#46789=CARTESIAN_POINT('',(-20.1,-3.933,-4.81653586104654E-16));
#46790=CARTESIAN_POINT('Ctrl Pts',(-15.862836477965,-3.92749965338984,0.00198301116285243));
#46791=CARTESIAN_POINT('Ctrl Pts',(-15.8895921847211,-3.929911697341,0.532649718284621));
#46792=CARTESIAN_POINT('Ctrl Pts',(-15.9163478914771,-3.82991474772018,
1.06244554991683));
#46793=CARTESIAN_POINT('Ctrl Pts',(-15.9431035982331,-3.62319942873785,
1.54668685901589));
#46794=CARTESIAN_POINT('Ctrl Pts',(-16.0093626070631,-3.11128052221676,
2.74588333205284));
#46795=CARTESIAN_POINT('Ctrl Pts',(-16.0756216158931,-1.94488189277277,
3.66570417872142));
#46796=CARTESIAN_POINT('Ctrl Pts',(-16.1418806247231,-0.659379616892197,
3.88394644908117));
#46797=CARTESIAN_POINT('Ctrl Pts',(-16.2081396335531,0.626122658988377,
4.10218871944093));
#46798=CARTESIAN_POINT('Ctrl Pts',(-16.2743986423831,2.03072858130552,3.61885241349186));
#46799=CARTESIAN_POINT('Ctrl Pts',(-16.3406576512131,2.90973762197645,2.65579150308084));
#46800=CARTESIAN_POINT('Ctrl Pts',(-16.4069166600431,3.78874666264738,1.69273059266982));
#46801=CARTESIAN_POINT('Ctrl Pts',(-16.4731756688731,4.14215882167208,0.249945077796819));
#46802=CARTESIAN_POINT('Ctrl Pts',(-16.5394346777031,3.80775845969318,-1.0103396865036));
#46803=CARTESIAN_POINT('Ctrl Pts',(-16.605693686533,3.47335809771428,-2.27062445080401));
#46804=CARTESIAN_POINT('Ctrl Pts',(-16.671952695363,2.45114521473181,-3.34840846453186));
#46805=CARTESIAN_POINT('Ctrl Pts',(-16.738211704193,1.21030936065731,-3.74899482213246));
#46806=CARTESIAN_POINT('Ctrl Pts',(-16.804470713023,-0.0305264934171873,
-4.14958117973306));
#46807=CARTESIAN_POINT('Ctrl Pts',(-16.870729721853,-1.4899853185837,-3.87296988120641));
#46808=CARTESIAN_POINT('Ctrl Pts',(-16.936988730683,-2.4981862514277,-3.04612439622297));
#46809=CARTESIAN_POINT('Ctrl Pts',(-16.9956046464437,-3.39008943550714,
-2.31465699049648));
#46810=CARTESIAN_POINT('Ctrl Pts',(-17.0542205622044,-3.92883705846707,
-1.15257492700707));
#46811=CARTESIAN_POINT('Ctrl Pts',(-17.112836477965,-3.93744710033063,0.002522420057968));
#46812=CARTESIAN_POINT('Ctrl Pts',(-17.296163522035,-3.93695989693636,0.00276125700748165));
#46813=CARTESIAN_POINT('Ctrl Pts',(-17.2385279418436,-3.92790050891893,
-1.13338475642016));
#46814=CARTESIAN_POINT('Ctrl Pts',(-17.1808923616523,-3.40920089730388,
-2.27674248904084));
#46815=CARTESIAN_POINT('Ctrl Pts',(-17.123256781461,-2.54294257060525,-3.00886164266523));
#46816=CARTESIAN_POINT('Ctrl Pts',(-17.056997772631,-1.54707477631489,-3.85052037679398));
#46817=CARTESIAN_POINT('Ctrl Pts',(-16.990738763801,-0.0918643927028295,
-4.14867556603334));
#46818=CARTESIAN_POINT('Ctrl Pts',(-16.924479754971,1.15475729573842,-3.76647596650864));
#46819=CARTESIAN_POINT('Ctrl Pts',(-16.858220746141,2.40137898417968,-3.38427636698394));
#46820=CARTESIAN_POINT('Ctrl Pts',(-16.791961737311,3.43941197745014,-2.32172197869517));
#46821=CARTESIAN_POINT('Ctrl Pts',(-16.725702728481,3.7924062321702,-1.06651801778504));
#46822=CARTESIAN_POINT('Ctrl Pts',(-16.6594437196511,4.14540048689025,0.188685943125091));
#46823=CARTESIAN_POINT('Ctrl Pts',(-16.5931847108211,3.81335600305992,1.63653947665657));
#46824=CARTESIAN_POINT('Ctrl Pts',(-16.5269257019911,2.94867920387608,2.612488330913));
#46825=CARTESIAN_POINT('Ctrl Pts',(-16.4606666931611,2.08400240469223,3.58843718516944));
#46826=CARTESIAN_POINT('Ctrl Pts',(-16.3944076843311,0.686693290154852,
4.09248136015081));
#46827=CARTESIAN_POINT('Ctrl Pts',(-16.3281486755011,-0.601893685968137,
3.89326737738197));
#46828=CARTESIAN_POINT('Ctrl Pts',(-16.2618896666711,-1.89048066209112,
3.69405339461314));
#46829=CARTESIAN_POINT('Ctrl Pts',(-16.1956306578411,-3.07034549979972,
2.79158125409412));
#46830=CARTESIAN_POINT('Ctrl Pts',(-16.1293716490111,-3.59993725883069,
1.60008076770775));
#46831=CARTESIAN_POINT('Ctrl Pts',(-16.1016356066857,-3.82162453884031,
1.10131828235401));
#46832=CARTESIAN_POINT('Ctrl Pts',(-16.0738995643604,-3.92936691994989,
0.551910450100659));
#46833=CARTESIAN_POINT('Ctrl Pts',(-16.046163522035,-3.92722756002595,0.00170206837946952));
#46834=CARTESIAN_POINT('Origin',(-20.1,0.,0.));
#46835=CARTESIAN_POINT('',(-14.612836477965,-3.92993428904087,-0.00292452251886177));
#46836=CARTESIAN_POINT('',(-14.796163522035,-3.93066717675506,-0.00339337507098336));
#46837=CARTESIAN_POINT('',(-20.1,-3.933,-4.81653586104654E-16));
#46838=CARTESIAN_POINT('Ctrl Pts',(-14.612836477965,-3.92993428904087,-0.00292452251886177));
#46839=CARTESIAN_POINT('Ctrl Pts',(-14.6587047984078,-3.92274597267032,
0.905157682402563));
#46840=CARTESIAN_POINT('Ctrl Pts',(-14.7045731188505,-3.60989172825119,
1.81749520012196));
#46841=CARTESIAN_POINT('Ctrl Pts',(-14.7504414392932,-3.03423748762575,
2.51256698125943));
#46842=CARTESIAN_POINT('Ctrl Pts',(-14.8167004481232,-2.20267707633405,
3.51663180943119));
#46843=CARTESIAN_POINT('Ctrl Pts',(-14.8829594569532,-0.822726637212052,
4.06732386343745));
#46844=CARTESIAN_POINT('Ctrl Pts',(-14.9492184657832,0.471837982743719,
3.91125962200143));
#46845=CARTESIAN_POINT('Ctrl Pts',(-15.0154774746132,1.76640260269949,3.75519538056541));
#46846=CARTESIAN_POINT('Ctrl Pts',(-15.0817364834432,2.97558140348904,2.89237484368711));
#46847=CARTESIAN_POINT('Ctrl Pts',(-15.1479954922732,3.54456962503122,1.71914580902439));
#46848=CARTESIAN_POINT('Ctrl Pts',(-15.2142545011032,4.1135578465734,0.545916774361676));
#46849=CARTESIAN_POINT('Ctrl Pts',(-15.2805135099332,4.04235548886822,-0.937720758085456));
#46850=CARTESIAN_POINT('Ctrl Pts',(-15.3467725187632,3.36354093984507,-2.05095209846013));
#46851=CARTESIAN_POINT('Ctrl Pts',(-15.4130315275932,2.68472639082192,-3.1641834388348));
#46852=CARTESIAN_POINT('Ctrl Pts',(-15.4792905364232,1.39829965048081,-3.907008587137));
#46853=CARTESIAN_POINT('Ctrl Pts',(-15.5455495452532,0.0947746782110898,
-3.93839117418686));
#46854=CARTESIAN_POINT('Ctrl Pts',(-15.6118085540831,-1.20875029405863,
-3.96977376123672));
#46855=CARTESIAN_POINT('Ctrl Pts',(-15.6780675629131,-2.52937349825695,
-3.28971378703422));
#46856=CARTESIAN_POINT('Ctrl Pts',(-15.7443265717431,-3.26096550855702,
-2.21039775023031));
#46857=CARTESIAN_POINT('Ctrl Pts',(-15.7838298738171,-3.69713714299747,
-1.56691472523465));
#46858=CARTESIAN_POINT('Ctrl Pts',(-15.8233331758911,-3.92393840562737,
-0.781516652037125));
#46859=CARTESIAN_POINT('Ctrl Pts',(-15.862836477965,-3.92749965338984,0.00198301116285243));
#46860=CARTESIAN_POINT('Ctrl Pts',(-16.046163522035,-3.92722756002595,0.00170206837946952));
#46861=CARTESIAN_POINT('Ctrl Pts',(-16.0076405555304,-3.9242561739239,-0.762489837983766));
#46862=CARTESIAN_POINT('Ctrl Pts',(-15.9691175890257,-3.70931400904017,
-1.5282260691143));
#46863=CARTESIAN_POINT('Ctrl Pts',(-15.9305946225211,-3.29328759331302,
-2.16195612127992));
#46864=CARTESIAN_POINT('Ctrl Pts',(-15.8643356136911,-2.57772748841107,
-3.25196369162747));
#46865=CARTESIAN_POINT('Ctrl Pts',(-15.7980766048612,-1.26728859825383,
-3.95145000006882));
#46866=CARTESIAN_POINT('Ctrl Pts',(-15.7318175960312,0.0365514847583181,
-3.93935038839483));
#46867=CARTESIAN_POINT('Ctrl Pts',(-15.6655585872012,1.34039156777047,-3.92725077672083));
#46868=CARTESIAN_POINT('Ctrl Pts',(-15.5992995783712,2.63763284363753,-3.2035652449315));
#46869=CARTESIAN_POINT('Ctrl Pts',(-15.5330405695412,3.33284158193514,-2.10047074141391));
#46870=CARTESIAN_POINT('Ctrl Pts',(-15.4667815607112,4.02805032023276,-0.997376237896311));
#46871=CARTESIAN_POINT('Ctrl Pts',(-15.4005225518812,4.12122652096094,0.485127237349519));
#46872=CARTESIAN_POINT('Ctrl Pts',(-15.3342635430512,3.56962055023412,1.66660105852033));
#46873=CARTESIAN_POINT('Ctrl Pts',(-15.2680045342212,3.01801457950731,2.84807487969113));
#46874=CARTESIAN_POINT('Ctrl Pts',(-15.2017455253912,1.82162643732546,3.72851904678691));
#46875=CARTESIAN_POINT('Ctrl Pts',(-15.1354865165612,0.529555795411518,
3.90377691175494));
#46876=CARTESIAN_POINT('Ctrl Pts',(-15.0692275077312,-0.762514846502421,
4.07903477672298));
#46877=CARTESIAN_POINT('Ctrl Pts',(-15.0029684989012,-2.15026798814847,
3.5491063395633));
#46878=CARTESIAN_POINT('Ctrl Pts',(-14.9367094900712,-2.99666853050174,
2.55730054859198));
#46879=CARTESIAN_POINT('Ctrl Pts',(-14.8898608340592,-3.59511889306143,
1.85604091382695));
#46880=CARTESIAN_POINT('Ctrl Pts',(-14.8430121780471,-3.92293383932689,
0.923877483478437));
#46881=CARTESIAN_POINT('Ctrl Pts',(-14.796163522035,-3.93066717675506,-0.00339337507098336));
#46882=CARTESIAN_POINT('Origin',(-28.5777734492731,0.,0.));
#46883=CARTESIAN_POINT('',(-14.2027734492731,-3.22023791762178,-0.00239639078269415));
#46884=CARTESIAN_POINT('',(-13.9562265507269,-3.22274745212571,-5.48329643912382E-7));
#46885=CARTESIAN_POINT('',(-28.5777734492731,-3.22275,-1.83004677902795E-13));
#46886=CARTESIAN_POINT('',(-13.9553333333333,-1.03523973309624,-3.05194958305651));
#46887=CARTESIAN_POINT('Ctrl Pts',(-14.2027734492731,-3.22023791762178,
-0.00239639078269425));
#46888=CARTESIAN_POINT('Ctrl Pts',(-14.1823827608858,-3.22285639546545,
-0.333182212003909));
#46889=CARTESIAN_POINT('Ctrl Pts',(-14.0999027222393,-3.03322933916847,
-1.66841872358004));
#46890=CARTESIAN_POINT('Ctrl Pts',(-14.0174226835927,-1.98323022307269,
-2.73145967097912));
#46891=CARTESIAN_POINT('Ctrl Pts',(-13.9553333333333,-1.03598926702581,
-3.05747757600544));
#46892=CARTESIAN_POINT('',(-13.9553333333333,-3.22271751746272,-0.0144694553766564));
#46893=CARTESIAN_POINT('Origin',(-13.9553333333333,0.,0.));
#46894=CARTESIAN_POINT('Ctrl Pts',(-13.9562265507269,-3.22274745212571,
-5.48329644236558E-7));
#46895=CARTESIAN_POINT('Ctrl Pts',(-13.9559288115957,-3.22274914287197,
-0.00482335248839003));
#46896=CARTESIAN_POINT('Ctrl Pts',(-13.9556310724645,-3.2227391724512,-0.00964633599337804));
#46897=CARTESIAN_POINT('Ctrl Pts',(-13.9553333333333,-3.22271751746272,
-0.0144694553766564));
#46898=CARTESIAN_POINT('Origin',(-28.5777734492731,0.,0.));
#46899=CARTESIAN_POINT('',(-15.4527734492731,-3.21824294634175,0.00162490445582779));
#46900=CARTESIAN_POINT('',(-15.2062265507269,-3.22083845509468,-0.00278057450064706));
#46901=CARTESIAN_POINT('',(-28.5777734492731,-3.22275,-1.83004677902795E-13));
#46902=CARTESIAN_POINT('Ctrl Pts',(-15.4527734492731,-3.21824294634175,
0.00162490445582791));
#46903=CARTESIAN_POINT('Ctrl Pts',(-15.4132701471991,-3.21532481483233,
-0.640384640313474));
#46904=CARTESIAN_POINT('Ctrl Pts',(-15.3075078362952,-2.71776457270222,
-2.36340351127251));
#46905=CARTESIAN_POINT('Ctrl Pts',(-15.1354865165612,0.0916700791133597,
-3.81013263943217));
#46906=CARTESIAN_POINT('Ctrl Pts',(-14.9367094900712,3.25401315877339,-1.98409164271898));
#46907=CARTESIAN_POINT('Ctrl Pts',(-14.7379324635813,3.42904549919622,1.66304249739848));
#46908=CARTESIAN_POINT('Ctrl Pts',(-14.5391554370913,0.456596238902905,
3.78406071648658));
#46909=CARTESIAN_POINT('Ctrl Pts',(-14.3607690989886,-2.58767128823935,
2.56919539238608));
#46910=CARTESIAN_POINT('Ctrl Pts',(-14.2486417697158,-3.21434772016868,
0.74169766614858));
#46911=CARTESIAN_POINT('Ctrl Pts',(-14.2027734492731,-3.22023791762178,
-0.00239639078269425));
#46912=CARTESIAN_POINT('Ctrl Pts',(-15.2062265507269,-3.22083845509468,
-0.00278057450064713));
#46913=CARTESIAN_POINT('Ctrl Pts',(-15.186816197909,-3.22346391822557,-0.317588440328601));
#46914=CARTESIAN_POINT('Ctrl Pts',(-15.1011468362611,-3.03633781573977,
-1.70398423664175));
#46915=CARTESIAN_POINT('Ctrl Pts',(-14.9492184657832,-1.04956382363505,
-3.66415224416977));
#46916=CARTESIAN_POINT('Ctrl Pts',(-14.7504414392933,2.51414376359986,-2.86419653732846));
#46917=CARTESIAN_POINT('Ctrl Pts',(-14.5516644128032,3.76833505696647,0.563263663837553));
#46918=CARTESIAN_POINT('Ctrl Pts',(-14.3528873863133,1.56631945652084,3.47714249206992));
#46919=CARTESIAN_POINT('Ctrl Pts',(-14.1544080989545,-2.07437419278699,
3.19251685865474));
#46920=CARTESIAN_POINT('Ctrl Pts',(-14.0221878204257,-3.22237288338974,
1.0684457944476));
#46921=CARTESIAN_POINT('Ctrl Pts',(-13.9562265507269,-3.22274745212571,
-5.48329644236558E-7));
#46922=CARTESIAN_POINT('Origin',(-28.5777734492731,0.,0.));
#46923=CARTESIAN_POINT('',(-16.7027734492731,-3.2263940103205,0.00206690293443917));
#46924=CARTESIAN_POINT('',(-16.4562265507269,-3.21801998959411,0.00139469638163969));
#46925=CARTESIAN_POINT('',(-28.5777734492731,-3.22275,-1.83004677902795E-13));
#46926=CARTESIAN_POINT('Ctrl Pts',(-16.7027734492731,-3.2263940103205,0.002066902934439));
#46927=CARTESIAN_POINT('Ctrl Pts',(-16.6441575335124,-3.21933883299632,
-0.944434489197185));
#46928=CARTESIAN_POINT('Ctrl Pts',(-16.5192826089217,-2.27886282222011,
-2.97304725088416));
#46929=CARTESIAN_POINT('Ctrl Pts',(-16.3281486755011,1.17088524590524,-3.62687816153355));
#46930=CARTESIAN_POINT('Ctrl Pts',(-16.1293716490111,3.68372778490734,-0.977428557993123));
#46931=CARTESIAN_POINT('Ctrl Pts',(-15.9305946225211,2.81495659078308,2.56928160070777));
#46932=CARTESIAN_POINT('Ctrl Pts',(-15.7318175960312,-0.637899043196787,
3.75743726813516));
#46933=CARTESIAN_POINT('Ctrl Pts',(-15.5725438716151,-2.93536387380584,
1.94565869403867));
#46934=CARTESIAN_POINT('Ctrl Pts',(-15.4795291560291,-3.22021940569686,
0.436459923621029));
#46935=CARTESIAN_POINT('Ctrl Pts',(-15.4527734492731,-3.21824294634175,
0.00162490445582791));
#46936=CARTESIAN_POINT('Ctrl Pts',(-16.4562265507269,-3.21801998959411,
0.00139469638163962));
#46937=CARTESIAN_POINT('Ctrl Pts',(-16.4177035842223,-3.21558519819808,
-0.624793827959028));
#46938=CARTESIAN_POINT('Ctrl Pts',(-16.3129216088877,-2.73652383299444,
-2.3314605700088));
#46939=CARTESIAN_POINT('Ctrl Pts',(-16.1418806247231,0.0353578955585694,
-3.81103610176739));
#46940=CARTESIAN_POINT('Ctrl Pts',(-15.9431035982331,3.22428567725235,-2.0320448374088));
#46941=CARTESIAN_POINT('Ctrl Pts',(-15.7443265717431,3.45333495329863,1.6123015202179));
#46942=CARTESIAN_POINT('Ctrl Pts',(-15.5455495452532,0.512328175864222,
3.77664281656251));
#46943=CARTESIAN_POINT('Ctrl Pts',(-15.3661828715811,-2.56597725945458,
2.60115883494905));
#46944=CARTESIAN_POINT('Ctrl Pts',(-15.253075206739,-3.21450166048588,0.757036908181897));
#46945=CARTESIAN_POINT('Ctrl Pts',(-15.2062265507269,-3.22083845509468,
-0.00278057450064713));
#46946=CARTESIAN_POINT('Origin',(-28.5777734492731,0.,0.));
#46947=CARTESIAN_POINT('',(-17.9527734492731,-3.22471002427666,-0.0027024083209955));
#46948=CARTESIAN_POINT('',(-17.7062265507269,-3.22599478969022,0.00226260895499958));
#46949=CARTESIAN_POINT('',(-28.5777734492731,-3.22275,-1.83004677902795E-13));
#46950=CARTESIAN_POINT('Ctrl Pts',(-17.9527734492731,-3.22471002427666,
-0.00270240832099557));
#46951=CARTESIAN_POINT('Ctrl Pts',(-17.9413039286557,-3.22637486097873,
-0.188158555526165));
#46952=CARTESIAN_POINT('Ctrl Pts',(-17.8635753992083,-3.12731663875485,
-1.44321058791824));
#46953=CARTESIAN_POINT('Ctrl Pts',(-17.719587860931,-1.47950656459142,-3.51230314164857));
#46954=CARTESIAN_POINT('Ctrl Pts',(-17.520810834441,2.15348704471131,-3.14447240364953));
#46955=CARTESIAN_POINT('Ctrl Pts',(-17.322033807951,3.80960974798971,0.109939997816874));
#46956=CARTESIAN_POINT('Ctrl Pts',(-17.123256781461,1.96856401336108,3.2634289244733));
#46957=CARTESIAN_POINT('Ctrl Pts',(-16.924479754971,-1.67959578872999,3.42113600634526));
#46958=CARTESIAN_POINT('Ctrl Pts',(-16.7843186442417,-3.16479457102735,
1.31787827406947));
#46959=CARTESIAN_POINT('Ctrl Pts',(-16.7104165423424,-3.22731395460883,
0.125483864632017));
#46960=CARTESIAN_POINT('Ctrl Pts',(-16.7027734492731,-3.2263940103205,0.002066902934439));
#46961=CARTESIAN_POINT('Ctrl Pts',(-17.7062265507269,-3.22599478969022,
0.00226260895499947));
#46962=CARTESIAN_POINT('Ctrl Pts',(-17.6485909705356,-3.21857141243789,
-0.928709820430633));
#46963=CARTESIAN_POINT('Ctrl Pts',(-17.5246963815143,-2.30492056053424,
-2.94264957100572));
#46964=CARTESIAN_POINT('Ctrl Pts',(-17.334542783663,1.11714296776071,-3.64378942704172));
#46965=CARTESIAN_POINT('Ctrl Pts',(-17.135765757173,3.66887510281969,-1.03177786727233));
#46966=CARTESIAN_POINT('Ctrl Pts',(-16.936988730683,2.85263073953649,2.52739068741007));
#46967=CARTESIAN_POINT('Ctrl Pts',(-16.738211704193,-0.582287604380603,
3.76645122510734));
#46968=CARTESIAN_POINT('Ctrl Pts',(-16.5779576442077,-2.92058117340316,
1.97790330423196));
#46969=CARTESIAN_POINT('Ctrl Pts',(-16.4839625930523,-3.21977300820459,
0.452242411152104));
#46970=CARTESIAN_POINT('Ctrl Pts',(-16.4562265507269,-3.21801998959411,
0.00139469638163962));
#46971=CARTESIAN_POINT('Origin',(-28.5777734492731,0.,0.));
#46972=CARTESIAN_POINT('',(-19.2027734492731,-3.21757428963995,-0.000678758514853295));
#46973=CARTESIAN_POINT('',(-18.9562265507269,-3.22516952318429,-0.00257345280792048));
#46974=CARTESIAN_POINT('',(-28.5777734492731,-3.22275,-1.83004677902795E-13));
#46975=CARTESIAN_POINT('Ctrl Pts',(-19.2027734492731,-3.21757428963995,
-0.000678758514853252));
#46976=CARTESIAN_POINT('Ctrl Pts',(-19.172191314969,-3.21850772850764,-0.497962082277344));
#46977=CARTESIAN_POINT('Ctrl Pts',(-19.0753501718349,-2.87588199447191,
-2.07143695563862));
#46978=CARTESIAN_POINT('Ctrl Pts',(-18.9122500198708,-0.420152939479476,
-3.78796576074431));
#46979=CARTESIAN_POINT('Ctrl Pts',(-18.7134729933808,2.95844202985016,-2.40267223202429));
#46980=CARTESIAN_POINT('Ctrl Pts',(-18.5146959668909,3.62122866324853,1.18824074591766));
#46981=CARTESIAN_POINT('Ctrl Pts',(-18.3159189404009,0.959778114968857,
3.68836536418065));
#46982=CARTESIAN_POINT('Ctrl Pts',(-18.1286114345283,-2.37833073469481,
2.85373001603029));
#46983=CARTESIAN_POINT('Ctrl Pts',(-18.0075629374857,-3.21675715912152,
0.883214948664705));
#46984=CARTESIAN_POINT('Ctrl Pts',(-17.9527734492731,-3.22471002427666,
-0.00270240832099557));
#46985=CARTESIAN_POINT('Ctrl Pts',(-18.9562265507269,-3.2251695231843,-0.00257345280792092));
#46986=CARTESIAN_POINT('Ctrl Pts',(-18.9457373656789,-3.22664687306115,
-0.172115406970832));
#46987=CARTESIAN_POINT('Ctrl Pts',(-18.8689891718008,-3.13729927908916,
-1.41107459021403));
#46988=CARTESIAN_POINT('Ctrl Pts',(-18.7259819690928,-1.53126558554944,
-3.49004799470226));
#46989=CARTESIAN_POINT('Ctrl Pts',(-18.5272049426028,2.10676807472235,-3.17596246694));
#46990=CARTESIAN_POINT('Ctrl Pts',(-18.3284279161128,3.81081816296161,0.0536121173318595));
#46991=CARTESIAN_POINT('Ctrl Pts',(-18.1296508896229,2.01659055559616,3.23397151708182));
#46992=CARTESIAN_POINT('Ctrl Pts',(-17.9308738631329,-1.62883890977077,
3.44559039419421));
#46993=CARTESIAN_POINT('Ctrl Pts',(-17.7897324168342,-3.1555709823932,1.34996225449272));
#46994=CARTESIAN_POINT('Ctrl Pts',(-17.7148499793656,-3.22710547450993,
0.14155459287759));
#46995=CARTESIAN_POINT('Ctrl Pts',(-17.7062265507269,-3.22599478969022,
0.00226260895499947));
#46996=CARTESIAN_POINT('Origin',(-28.5777734492731,0.,0.));
#46997=CARTESIAN_POINT('',(-20.4527734492731,-3.22221210701407,0.00296761955232107));
#46998=CARTESIAN_POINT('',(-20.2062265507269,-3.21769251484553,-0.000932565804893093));
#46999=CARTESIAN_POINT('',(-28.5777734492731,-3.22275,-1.83004677902795E-13));
#47000=CARTESIAN_POINT('Ctrl Pts',(-20.4527734492731,-3.22221210701407,
0.00296761955232077));
#47001=CARTESIAN_POINT('Ctrl Pts',(-20.4030787012823,-3.21489552804955,
-0.802170257958906));
#47002=CARTESIAN_POINT('Ctrl Pts',(-20.2871249444615,-2.50155693228504,
-2.69237598717909));
#47003=CARTESIAN_POINT('Ctrl Pts',(-20.1049121788107,0.673860123029691,
-3.75114990807958));
#47004=CARTESIAN_POINT('Ctrl Pts',(-19.9061351523207,3.51934796221725,-1.4626698257142));
#47005=CARTESIAN_POINT('Ctrl Pts',(-19.7073581258307,3.13412367710237,2.16852066508976));
#47006=CARTESIAN_POINT('Ctrl Pts',(-19.5085810993407,-0.128182235481189,
3.80903956563999));
#47007=CARTESIAN_POINT('Ctrl Pts',(-19.3403862071549,-2.78901177056585,
2.2384811989213));
#47008=CARTESIAN_POINT('Ctrl Pts',(-19.238450323799,-3.21648534728463,0.579448009920417));
#47009=CARTESIAN_POINT('Ctrl Pts',(-19.2027734492731,-3.21757428963995,
-0.000678758514853252));
#47010=CARTESIAN_POINT('Ctrl Pts',(-20.2062265507269,-3.21769251484553,
-0.00093256580489396));
#47011=CARTESIAN_POINT('Ctrl Pts',(-20.1766247519921,-3.21893644686449,
-0.482230723198207));
#47012=CARTESIAN_POINT('Ctrl Pts',(-20.0807639444274,-2.89158218271902,
-2.03923190959996));
#47013=CARTESIAN_POINT('Ctrl Pts',(-19.9186441280327,-0.476102850960359,
-3.7813404214166));
#47014=CARTESIAN_POINT('Ctrl Pts',(-19.7198671015427,2.92260070569343,-2.44614276413548));
#47015=CARTESIAN_POINT('Ctrl Pts',(-19.5210900750527,3.63839775937779,1.13457968101029));
#47016=CARTESIAN_POINT('Ctrl Pts',(-19.3223130485627,1.01419664261627,3.67377387388617));
#47017=CARTESIAN_POINT('Ctrl Pts',(-19.1340252071208,-2.35341883760494,
2.8844660712419));
#47018=CARTESIAN_POINT('Ctrl Pts',(-19.0119963745089,-3.21731461911702,
0.898862155774589));
#47019=CARTESIAN_POINT('Ctrl Pts',(-18.9562265507269,-3.2251695231843,-0.00257345280792092));
#47020=CARTESIAN_POINT('Origin',(-28.5777734492731,0.,0.));
#47021=CARTESIAN_POINT('',(-21.7027734492731,-3.2278730893709,-0.000762706468288871));
#47022=CARTESIAN_POINT('',(-21.4562265507269,-3.22173931860895,0.00294029562399406));
#47023=CARTESIAN_POINT('',(-28.5777734492731,-3.22275,-1.83004677902795E-13));
#47024=CARTESIAN_POINT('Ctrl Pts',(-21.7027734492731,-3.2278730893709,-0.000762706468289505));
#47025=CARTESIAN_POINT('Ctrl Pts',(-21.7002250964256,-3.22800402191512,
-0.0418624340926581));
#47026=CARTESIAN_POINT('Ctrl Pts',(-21.631417734748,-3.20864937647278,-1.15145847964987));
#47027=CARTESIAN_POINT('Ctrl Pts',(-21.4963513642405,-1.93721818400033,
-3.28213326926849));
#47028=CARTESIAN_POINT('Ctrl Pts',(-21.2975743377506,1.71228483279679,-3.40489261991708));
#47029=CARTESIAN_POINT('Ctrl Pts',(-21.0987973112606,3.78993436216897,-0.402008244909776));
#47030=CARTESIAN_POINT('Ctrl Pts',(-20.9000202847706,2.38847724265994,2.96991406583087));
#47031=CARTESIAN_POINT('Ctrl Pts',(-20.7012432582806,-1.20556852363392,
3.6154968722977));
#47032=CARTESIAN_POINT('Ctrl Pts',(-20.5521609797814,-3.07107543849641,
1.61045897788706));
#47033=CARTESIAN_POINT('Ctrl Pts',(-20.4693377101123,-3.22465087020975,
0.271336297406685));
#47034=CARTESIAN_POINT('Ctrl Pts',(-20.4527734492731,-3.22221210701407,
0.00296761955232077));
#47035=CARTESIAN_POINT('Ctrl Pts',(-21.4562265507269,-3.22173931860895,
0.00294029562399399));
#47036=CARTESIAN_POINT('Ctrl Pts',(-21.4075121383054,-3.21471913280839,
-0.786608964437968));
#47037=CARTESIAN_POINT('Ctrl Pts',(-21.292538717054,-2.52408530047148,-2.66105030950266));
#47038=CARTESIAN_POINT('Ctrl Pts',(-21.1113062869725,0.618334760982468,
-3.76070092288226));
#47039=CARTESIAN_POINT('Ctrl Pts',(-20.9125292604826,3.49734092856599,-1.51453482522831));
#47040=CARTESIAN_POINT('Ctrl Pts',(-20.7137522339926,3.16583712036473,2.12195302366768));
#47041=CARTESIAN_POINT('Ctrl Pts',(-20.5149752075026,-0.0718608118791213,
3.81051772482967));
#47042=CARTESIAN_POINT('Ctrl Pts',(-20.3457999797474,-2.77125860116402,
2.2705412322501));
#47043=CARTESIAN_POINT('Ctrl Pts',(-20.2428837608221,-3.21615209908324,
0.59508012356279));
#47044=CARTESIAN_POINT('Ctrl Pts',(-20.2062265507269,-3.21769251484553,
-0.00093256580489396));
#47045=CARTESIAN_POINT('Origin',(-28.5777734492731,0.,0.));
#47046=CARTESIAN_POINT('',(-22.9527734492731,-3.21991554799802,-0.0025677011159218));
#47047=CARTESIAN_POINT('',(-22.7062265507269,-3.22800631070464,-0.000473251210255654));
#47048=CARTESIAN_POINT('',(-28.5777734492731,-3.22275,-1.83004677902795E-13));
#47049=CARTESIAN_POINT('Ctrl Pts',(-22.9527734492731,-3.21991554799802,
-0.00256770111592211));
#47050=CARTESIAN_POINT('Ctrl Pts',(-22.9311124827388,-3.22253028735674,
-0.35414605530089));
#47051=CARTESIAN_POINT('Ctrl Pts',(-22.8431925073746,-3.00720843641272,
-1.77805734035436));
#47052=CARTESIAN_POINT('Ctrl Pts',(-22.6890135231804,-0.924408668548408,
-3.69738843419269));
#47053=CARTESIAN_POINT('Ctrl Pts',(-22.4902364966904,2.60945901488757,-2.7777575280647));
#47054=CARTESIAN_POINT('Ctrl Pts',(-22.2914594702004,3.74787990632693,0.691815984784808));
#47055=CARTESIAN_POINT('Ctrl Pts',(-22.0926824437105,1.44579953705816,3.52631205824809));
#47056=CARTESIAN_POINT('Ctrl Pts',(-21.896453770068,-2.13697629406559,3.12886460489886));
#47057=CARTESIAN_POINT('Ctrl Pts',(-21.7664841052555,-3.22459968149505,
1.02676007562483));
#47058=CARTESIAN_POINT('Ctrl Pts',(-21.7027734492731,-3.2278730893709,-0.000762706468289505));
#47059=CARTESIAN_POINT('Ctrl Pts',(-22.7062265507269,-3.22800631070464,
-0.000473251210255806));
#47060=CARTESIAN_POINT('Ctrl Pts',(-22.7046585334487,-3.22805805244852,
-0.025759358427327));
#47061=CARTESIAN_POINT('Ctrl Pts',(-22.6368315073406,-3.21632122210707,
-1.11949996844933));
#47062=CARTESIAN_POINT('Ctrl Pts',(-22.5027454724024,-1.9855246223874,-3.2531371345379));
#47063=CARTESIAN_POINT('Ctrl Pts',(-22.3039684459124,1.66176444014233,-3.4298321060602));
#47064=CARTESIAN_POINT('Ctrl Pts',(-22.1051914194224,3.78357703340158,-0.45798924048176));
#47065=CARTESIAN_POINT('Ctrl Pts',(-21.9064143929325,2.43211891370082,2.93428132400969));
#47066=CARTESIAN_POINT('Ctrl Pts',(-21.7076373664425,-1.15199029393737,
3.63292274535707));
#47067=CARTESIAN_POINT('Ctrl Pts',(-21.557574752374,-3.05939350818334,1.64267923939091));
#47068=CARTESIAN_POINT('Ctrl Pts',(-21.4737711471354,-3.2242676530476,0.287298094966756));
#47069=CARTESIAN_POINT('Ctrl Pts',(-21.4562265507269,-3.22173931860895,
0.00294029562399399));
#47070=CARTESIAN_POINT('Origin',(-28.5777734492731,0.,0.));
#47071=CARTESIAN_POINT('',(-24.2027734492731,-3.21858419309814,0.00190193480539803));
#47072=CARTESIAN_POINT('',(-23.9562265507269,-3.22031942372998,-0.00269217174386716));
#47073=CARTESIAN_POINT('',(-28.5777734492731,-3.22275,-1.83004677902795E-13));
#47074=CARTESIAN_POINT('Ctrl Pts',(-24.2027734492731,-3.21858419309814,
0.00190193480539787));
#47075=CARTESIAN_POINT('Ctrl Pts',(-24.1619998690521,-3.21503940788334,
-0.660581282227665));
#47076=CARTESIAN_POINT('Ctrl Pts',(-24.0549672800012,-2.69295281648875,
-2.40476065474808));
#47077=CARTESIAN_POINT('Ctrl Pts',(-23.8816756821203,0.16465828588852,-3.80763393731814));
#47078=CARTESIAN_POINT('Ctrl Pts',(-23.6828986556303,3.29137222988386,-1.92148011273296));
#47079=CARTESIAN_POINT('Ctrl Pts',(-23.4841216291403,3.39665395902081,1.72857147389278));
#47080=CARTESIAN_POINT('Ctrl Pts',(-23.2853446026503,0.383854227871474,
3.79181560291581));
#47081=CARTESIAN_POINT('Ctrl Pts',(-23.1082285426946,-2.61461116784304,
2.52870393023895));
#47082=CARTESIAN_POINT('Ctrl Pts',(-22.9973714915688,-3.21453202753838,
0.721301489366681));
#47083=CARTESIAN_POINT('Ctrl Pts',(-22.9527734492731,-3.21991554799802,
-0.00256770111592211));
#47084=CARTESIAN_POINT('Ctrl Pts',(-23.9562265507269,-3.22031942372998,
-0.00269217174386771));
#47085=CARTESIAN_POINT('Ctrl Pts',(-23.935545919762,-3.22295957829101,-0.338252521270422));
#47086=CARTESIAN_POINT('Ctrl Pts',(-23.8486062799671,-3.02010243966437,
-1.74580737059892));
#47087=CARTESIAN_POINT('Ctrl Pts',(-23.6954076313422,-0.978964290720696,
-3.68331844135819));
#47088=CARTESIAN_POINT('Ctrl Pts',(-23.4966306048523,2.56811106183178,-2.81602834885952));
#47089=CARTESIAN_POINT('Ctrl Pts',(-23.2978535783623,3.75769675477037,0.636337094806224));
#47090=CARTESIAN_POINT('Ctrl Pts',(-23.0990765518723,1.49776930770217,3.50455359875708));
#47091=CARTESIAN_POINT('Ctrl Pts',(-22.9018675426605,-2.10841635961811,
3.15839155315196));
#47092=CARTESIAN_POINT('Ctrl Pts',(-22.7709175422787,-3.22587162458688,
1.04274442956557));
#47093=CARTESIAN_POINT('Ctrl Pts',(-22.7062265507269,-3.22800631070464,
-0.000473251210255806));
#47094=CARTESIAN_POINT('Origin',(-28.5777734492731,0.,0.));
#47095=CARTESIAN_POINT('',(-25.4527734492731,-3.22681880944319,0.00198271668292594));
#47096=CARTESIAN_POINT('',(-25.2062265507269,-3.2183080224723,0.00170933992184319));
#47097=CARTESIAN_POINT('',(-28.5777734492731,-3.22275,-1.83004677902795E-13));
#47098=CARTESIAN_POINT('Ctrl Pts',(-25.4527734492731,-3.22681880944319,
0.00198271668292602));
#47099=CARTESIAN_POINT('Ctrl Pts',(-25.3928872553654,-3.22038563950992,
-0.964597122860873));
#47100=CARTESIAN_POINT('Ctrl Pts',(-25.2667420526278,-2.244579208324,-3.01256650610898));
#47101=CARTESIAN_POINT('Ctrl Pts',(-25.0743378410601,1.24018106922513,-3.60361128581411));
#47102=CARTESIAN_POINT('Ctrl Pts',(-24.8755608145702,3.70175213266751,-0.906781358690897));
#47103=CARTESIAN_POINT('Ctrl Pts',(-24.6767837880802,2.76524014159366,2.62277736241376));
#47104=CARTESIAN_POINT('Ctrl Pts',(-24.4780067615902,-0.709761474991402,
3.74450018637222));
#47105=CARTESIAN_POINT('Ctrl Pts',(-24.3200033153212,-2.95404409032814,
1.90388762973689));
#47106=CARTESIAN_POINT('Ctrl Pts',(-24.2282588778821,-3.22079985260207,
0.415985482065448));
#47107=CARTESIAN_POINT('Ctrl Pts',(-24.2027734492731,-3.21858419309814,
0.00190193480539787));
#47108=CARTESIAN_POINT('Ctrl Pts',(-25.2062265507269,-3.2183080224723,0.00170933992184336));
#47109=CARTESIAN_POINT('Ctrl Pts',(-25.1664333060753,-3.21525215568242,
-0.644987807253467));
#47110=CARTESIAN_POINT('Ctrl Pts',(-25.0603810525937,-2.71217295639817,
-2.37289324999516));
#47111=CARTESIAN_POINT('Ctrl Pts',(-24.8880697902821,0.108362070287417,
-3.80963202337103));
#47112=CARTESIAN_POINT('Ctrl Pts',(-24.6892927637921,3.26260339792463,-1.96993487649339));
#47113=CARTESIAN_POINT('Ctrl Pts',(-24.4905157373022,3.42183734109356,1.67817626036435));
#47114=CARTESIAN_POINT('Ctrl Pts',(-24.2917387108122,0.439863865693541,
3.78572376365049));
#47115=CARTESIAN_POINT('Ctrl Pts',(-24.1136423152871,-2.59364198095809,
2.56033371879188));
#47116=CARTESIAN_POINT('Ctrl Pts',(-24.001804928592,-3.21450074428982,0.73685472279883));
#47117=CARTESIAN_POINT('Ctrl Pts',(-23.9562265507269,-3.22031942372998,
-0.00269217174386771));
#47118=CARTESIAN_POINT('Origin',(-13.9553333333333,5.160062080289E-16,2.1385152528819E-16));
#47119=CARTESIAN_POINT('',(-13.9553333333333,3.88062570733445,0.639713310456302));
#47120=CARTESIAN_POINT('Ctrl Pts',(-13.9553333333333,-1.03598926702577,
-3.05747757600545));
#47121=CARTESIAN_POINT('Ctrl Pts',(-13.9553333333333,-0.97444439476585,
-3.08634227761202));
#47122=CARTESIAN_POINT('Ctrl Pts',(-13.9553333333333,-0.912020754771081,
-3.11307510025756));
#47123=CARTESIAN_POINT('Ctrl Pts',(-13.9553333333333,-0.848797833127659,
-3.13759945495693));
#47124=CARTESIAN_POINT('Ctrl Pts',(-13.9553333333333,-0.753122772179508,
-3.17471208862814));
#47125=CARTESIAN_POINT('Ctrl Pts',(-13.9553333333333,-0.655618687658207,
-3.20676979988523));
#47126=CARTESIAN_POINT('Ctrl Pts',(-13.9553333333333,-0.55665830230821,
-3.23392646990319));
#47127=CARTESIAN_POINT('Ctrl Pts',(-13.9553333333333,-0.494205049156755,
-3.25106486706469));
#47128=CARTESIAN_POINT('Ctrl Pts',(-13.9553333333333,-0.431171105772932,
-3.26625041147114));
#47129=CARTESIAN_POINT('Ctrl Pts',(-13.9553333333333,-0.367644747143531,
-3.27951281571112));
#47130=CARTESIAN_POINT('Ctrl Pts',(-13.9553333333333,-0.327047912649835,
-3.28798822090568));
#47131=CARTESIAN_POINT('Ctrl Pts',(-13.9553333333333,-0.286249902435637,
-3.29567809271961));
#47132=CARTESIAN_POINT('Ctrl Pts',(-13.9553333333333,-0.245273098295,-3.3025886978361));
#47133=CARTESIAN_POINT('Ctrl Pts',(-13.9553333333333,-0.226865840120677,
-3.30569302222615));
#47134=CARTESIAN_POINT('Ctrl Pts',(-13.9553333333333,-0.20842389272401,
-3.30863977526898));
#47135=CARTESIAN_POINT('Ctrl Pts',(-13.9553333333333,-0.189961491201516,
-3.31142788908956));
#47136=CARTESIAN_POINT('Ctrl Pts',(-13.9553333333333,-0.0850514468879583,
-3.3272709604317));
#47137=CARTESIAN_POINT('Ctrl Pts',(-13.9553333333333,0.0206223431908923,
-3.33801358018381));
#47138=CARTESIAN_POINT('Ctrl Pts',(-13.9553333333333,0.126670272884673,
-3.34381218349164));
#47139=CARTESIAN_POINT('Ctrl Pts',(-13.9553333333333,0.227783133662497,
-3.34934094176786));
#47140=CARTESIAN_POINT('Ctrl Pts',(-13.9553333333333,0.329236905662223,
-3.35037480537384));
#47141=CARTESIAN_POINT('Ctrl Pts',(-13.9553333333333,0.430711103724674,
-3.34701090757602));
#47142=CARTESIAN_POINT('Ctrl Pts',(-13.9553333333333,0.475106065376996,
-3.34553920228947));
#47143=CARTESIAN_POINT('Ctrl Pts',(-13.9553333333333,0.519505098103338,
-3.34322525460124));
#47144=CARTESIAN_POINT('Ctrl Pts',(-13.9553333333333,0.563881915333782,
-3.34007494530072));
#47145=CARTESIAN_POINT('Ctrl Pts',(-13.9553333333333,0.58584474718944,-3.33851580433977));
#47146=CARTESIAN_POINT('Ctrl Pts',(-13.9553333333333,0.607802140900022,
-3.33675178165321));
#47147=CARTESIAN_POINT('Ctrl Pts',(-13.9553333333333,0.629750923720838,
-3.33478346606831));
#47148=CARTESIAN_POINT('Ctrl Pts',(-13.9553333333333,0.645395419510362,
-3.33338050422156));
#47149=CARTESIAN_POINT('Ctrl Pts',(-13.9553333333333,0.6610330550259,-3.33187393535576));
#47150=CARTESIAN_POINT('Ctrl Pts',(-13.9553333333333,0.676654075413203,
-3.33026504772646));
#47151=CARTESIAN_POINT('Ctrl Pts',(-13.9553333333333,0.787358794894414,
-3.31886301064675));
#47152=CARTESIAN_POINT('Ctrl Pts',(-13.9553333333333,0.897351501643973,
-3.30231524241035));
#47153=CARTESIAN_POINT('Ctrl Pts',(-13.9553333333333,1.00622074539013,-3.28078416772688));
#47154=CARTESIAN_POINT('Ctrl Pts',(-13.9553333333333,1.11680331542352,-3.25891424843516));
#47155=CARTESIAN_POINT('Ctrl Pts',(-13.9553333333333,1.22622766989774,-3.23190302698969));
#47156=CARTESIAN_POINT('Ctrl Pts',(-13.9553333333333,1.33407670763527,-3.19986895694082));
#47157=CARTESIAN_POINT('Ctrl Pts',(-13.9553333333333,1.44167031624772,-3.16791075622427));
#47158=CARTESIAN_POINT('Ctrl Pts',(-13.9553333333333,1.54769701641018,-3.13095340796043));
#47159=CARTESIAN_POINT('Ctrl Pts',(-13.9553333333333,1.65174263467817,-3.08906346075735));
#47160=CARTESIAN_POINT('Ctrl Pts',(-13.9553333333333,1.71930029668252,-3.06186397901429));
#47161=CARTESIAN_POINT('Ctrl Pts',(-13.9553333333333,1.78602270026487,-3.03258387425711));
#47162=CARTESIAN_POINT('Ctrl Pts',(-13.9553333333333,1.85179353602905,-3.00122997196956));
#47163=CARTESIAN_POINT('Ctrl Pts',(-13.9553333333333,1.87027794232932,-2.99241818993504));
#47164=CARTESIAN_POINT('Ctrl Pts',(-13.9553333333333,1.88868716769718,-2.98344255502655));
#47165=CARTESIAN_POINT('Ctrl Pts',(-13.9553333333333,1.90701857443447,-2.97430309205569));
#47166=CARTESIAN_POINT('Ctrl Pts',(-13.9553333333333,1.92415095587783,-2.96576142539321));
#47167=CARTESIAN_POINT('Ctrl Pts',(-13.9553333333333,1.94121695803161,-2.95707572927031));
#47168=CARTESIAN_POINT('Ctrl Pts',(-13.9553333333333,1.95819482658923,-2.94825646251065));
#47169=CARTESIAN_POINT('Ctrl Pts',(-13.9553333333333,2.06098978668038,-2.89485893669543));
#47170=CARTESIAN_POINT('Ctrl Pts',(-13.9553333333333,2.16071563092277,-2.83649011388479));
#47171=CARTESIAN_POINT('Ctrl Pts',(-13.9553333333333,2.25694248996472,-2.7732788016416));
#47172=CARTESIAN_POINT('Ctrl Pts',(-13.9553333333333,2.30934153235369,-2.73885793139112));
#47173=CARTESIAN_POINT('Ctrl Pts',(-13.9553333333333,2.36070308712004,-2.70300025428149));
#47174=CARTESIAN_POINT('Ctrl Pts',(-13.9553333333333,2.41095698484776,-2.66572010901368));
#47175=CARTESIAN_POINT('Ctrl Pts',(-13.9553333333333,2.50006598058015,-2.59961585728836));
#47176=CARTESIAN_POINT('Ctrl Pts',(-13.9553333333333,2.58569399841725,-2.529041984421));
#47177=CARTESIAN_POINT('Ctrl Pts',(-13.9553333333333,2.66776425450739,-2.45437987478522));
#47178=CARTESIAN_POINT('Ctrl Pts',(-13.9553333333333,2.75139660323382,-2.37829667622846));
#47179=CARTESIAN_POINT('Ctrl Pts',(-13.9553333333333,2.83133495883862,-2.29796765658672));
#47180=CARTESIAN_POINT('Ctrl Pts',(-13.9553333333333,2.90746923279272,-2.21375050651505));
#47181=CARTESIAN_POINT('Ctrl Pts',(-13.9553333333333,2.93145580090933,-2.187217378899));
#47182=CARTESIAN_POINT('Ctrl Pts',(-13.9553333333333,2.95506453274937,-2.1602980072191));
#47183=CARTESIAN_POINT('Ctrl Pts',(-13.9553333333333,2.97829128499789,-2.13300278094868));
#47184=CARTESIAN_POINT('Ctrl Pts',(-13.9553333333333,2.98871016252315,-2.12075889870061));
#47185=CARTESIAN_POINT('Ctrl Pts',(-13.9553333333333,2.99905384204844,-2.10843736379202));
#47186=CARTESIAN_POINT('Ctrl Pts',(-13.9553333333333,3.00931636832518,-2.09604582041943));
#47187=CARTESIAN_POINT('Ctrl Pts',(-13.9553333333333,3.08191587225961,-2.00838515309711));
#47188=CARTESIAN_POINT('Ctrl Pts',(-13.9553333333333,3.15031706995574,-1.91739553524079));
#47189=CARTESIAN_POINT('Ctrl Pts',(-13.9553333333333,3.21445896366597,-1.82349417167357));
#47190=CARTESIAN_POINT('Ctrl Pts',(-13.9553333333333,3.28071257870846,-1.72650132606391));
#47191=CARTESIAN_POINT('Ctrl Pts',(-13.9553333333333,3.34242236519139,-1.62640143226605));
#47192=CARTESIAN_POINT('Ctrl Pts',(-13.9553333333333,3.39949212600865,-1.52360685487494));
#47193=CARTESIAN_POINT('Ctrl Pts',(-13.9553333333333,3.45713807462249,-1.41977444273214));
#47194=CARTESIAN_POINT('Ctrl Pts',(-13.9553333333333,3.51005033110595,-1.31319198625781));
#47195=CARTESIAN_POINT('Ctrl Pts',(-13.9553333333333,3.55809281339713,-1.2042455082145));
#47196=CARTESIAN_POINT('Ctrl Pts',(-13.9553333333333,3.5898550154717,-1.13221800493205));
#47197=CARTESIAN_POINT('Ctrl Pts',(-13.9553333333333,3.61948792025525,-1.05915642697356));
#47198=CARTESIAN_POINT('Ctrl Pts',(-13.9553333333333,3.64694183534205,-0.985165363120071));
#47199=CARTESIAN_POINT('Ctrl Pts',(-13.9553333333333,3.66035272037872,-0.949021678405428));
#47200=CARTESIAN_POINT('Ctrl Pts',(-13.9553333333333,3.67324352307887,-0.912656128563678));
#47201=CARTESIAN_POINT('Ctrl Pts',(-13.9553333333333,3.685607658247,-0.876080550583037));
#47202=CARTESIAN_POINT('Ctrl Pts',(-13.9553333333333,3.69331037373375,-0.853294381787787));
#47203=CARTESIAN_POINT('Ctrl Pts',(-13.9553333333333,3.70081038899666,-0.830420968477908));
#47204=CARTESIAN_POINT('Ctrl Pts',(-13.9553333333333,3.70809603678459,-0.807495459346133));
#47205=CARTESIAN_POINT('Ctrl Pts',(-13.9553333333333,3.74524699475371,-0.69059375740188));
#47206=CARTESIAN_POINT('Ctrl Pts',(-13.9553333333333,3.77687334741109,-0.572212458485722));
#47207=CARTESIAN_POINT('Ctrl Pts',(-13.9553333333333,3.80287284700866,-0.452783927385374));
#47208=CARTESIAN_POINT('Ctrl Pts',(-13.9553333333333,3.82890220860145,-0.33321822540557));
#47209=CARTESIAN_POINT('Ctrl Pts',(-13.9553333333333,3.84929223191143,-0.212602085015147));
#47210=CARTESIAN_POINT('Ctrl Pts',(-13.9553333333333,3.86389824005303,-0.0913379545200216));
#47211=CARTESIAN_POINT('Ctrl Pts',(-13.9553333333333,3.87847911324018,0.0297174968913304));
#47212=CARTESIAN_POINT('Ctrl Pts',(-13.9553333333333,3.88729629975811,0.15141952707811));
#47213=CARTESIAN_POINT('Ctrl Pts',(-13.9553333333333,3.89015735625761,0.273386919606757));
#47214=CARTESIAN_POINT('Ctrl Pts',(-13.9553333333333,3.8930184127571,0.395354312135403));
#47215=CARTESIAN_POINT('Ctrl Pts',(-13.9553333333333,3.88992381340402,0.517587896581017));
#47216=CARTESIAN_POINT('Ctrl Pts',(-13.9553333333333,3.88062570733445,0.639713310456302));
#47217=CARTESIAN_POINT('',(-13.9553333333333,-3.933,-4.81653586104654E-16));
#47218=CARTESIAN_POINT('Origin',(-13.9553333333333,0.,0.));
#47219=CARTESIAN_POINT('',(-13.9553333333333,1.83776796987408,3.48100466478169));
#47220=CARTESIAN_POINT('Origin',(-13.9553333333333,0.,0.));
#47221=CARTESIAN_POINT('Ctrl Pts',(-13.9553333333333,1.83875391880586,3.48426281672735));
#47222=CARTESIAN_POINT('Ctrl Pts',(-13.9553333333333,1.76308895516893,3.51647153040244));
#47223=CARTESIAN_POINT('Ctrl Pts',(-13.9553333333333,1.68643718119151,3.54609006161243));
#47224=CARTESIAN_POINT('Ctrl Pts',(-13.9553333333333,1.60886810215454,3.57300966796364));
#47225=CARTESIAN_POINT('Ctrl Pts',(-13.9553333333333,1.49409022882316,3.61284223019423));
#47226=CARTESIAN_POINT('Ctrl Pts',(-13.9553333333333,1.37730380720653,3.64676788490432));
#47227=CARTESIAN_POINT('Ctrl Pts',(-13.9553333333333,1.25894917601004,3.67487673179449));
#47228=CARTESIAN_POINT('Ctrl Pts',(-13.9553333333333,1.19042394189699,3.69115125603004));
#47229=CARTESIAN_POINT('Ctrl Pts',(-13.9553333333333,1.12137289144904,3.7054748768118));
#47230=CARTESIAN_POINT('Ctrl Pts',(-13.9553333333333,1.05188174504114,3.7178572191697));
#47231=CARTESIAN_POINT('Ctrl Pts',(-13.9553333333333,0.99900121609365,3.7272797837314));
#47232=CARTESIAN_POINT('Ctrl Pts',(-13.9553333333333,0.945865841074519,
3.73557809047345));
#47233=CARTESIAN_POINT('Ctrl Pts',(-13.9553333333333,0.892513862605538,
3.74275424069541));
#47234=CARTESIAN_POINT('Ctrl Pts',(-13.9553333333333,0.870373911505189,
3.74573219239584));
#47235=CARTESIAN_POINT('Ctrl Pts',(-13.9553333333333,0.848195262249248,
3.74851695984359));
#47236=CARTESIAN_POINT('Ctrl Pts',(-13.9553333333333,0.825998844565343,
3.75110673049074));
#47237=CARTESIAN_POINT('Ctrl Pts',(-13.9553333333333,0.70366659282493,3.76537986587987));
#47238=CARTESIAN_POINT('Ctrl Pts',(-13.9553333333333,0.580670158678774,
3.77375230856627));
#47239=CARTESIAN_POINT('Ctrl Pts',(-13.9553333333333,0.457468363331996,
3.77631420882323));
#47240=CARTESIAN_POINT('Ctrl Pts',(-13.9553333333333,0.349666792403565,
3.77855587154807));
#47241=CARTESIAN_POINT('Ctrl Pts',(-13.9553333333333,0.241707527928521,
3.77634785611784));
#47242=CARTESIAN_POINT('Ctrl Pts',(-13.9553333333333,0.133905126459,3.76971649396968));
#47243=CARTESIAN_POINT('Ctrl Pts',(-13.9553333333333,0.0867415758160847,
3.76681527302986));
#47244=CARTESIAN_POINT('Ctrl Pts',(-13.9553333333333,0.039608186703455,
3.76306699939609));
#47245=CARTESIAN_POINT('Ctrl Pts',(-13.9553333333333,-0.0074678918743757,
3.75847207198772));
#47246=CARTESIAN_POINT('Ctrl Pts',(-13.9553333333333,-0.0364097747536519,
3.75564715846669));
#47247=CARTESIAN_POINT('Ctrl Pts',(-13.9553333333333,-0.0653299851271169,
3.75250221724033));
#47248=CARTESIAN_POINT('Ctrl Pts',(-13.9553333333333,-0.0942220930405801,
3.74903714231532));
#47249=CARTESIAN_POINT('Ctrl Pts',(-13.9553333333333,-0.116528637892405,
3.74636188409391));
#47250=CARTESIAN_POINT('Ctrl Pts',(-13.9553333333333,-0.138821572577901,
3.74349527660291));
#47251=CARTESIAN_POINT('Ctrl Pts',(-13.9553333333333,-0.161073145138907,
3.74044087441143));
#47252=CARTESIAN_POINT('Ctrl Pts',(-13.9553333333333,-0.278854314400997,
3.72427343004213));
#47253=CARTESIAN_POINT('Ctrl Pts',(-13.9553333333333,-0.395616864311933,
3.70283345101575));
#47254=CARTESIAN_POINT('Ctrl Pts',(-13.9553333333333,-0.510952667895199,
3.67619809061088));
#47255=CARTESIAN_POINT('Ctrl Pts',(-13.9553333333333,-0.625434416051205,
3.64975996361839));
#47256=CARTESIAN_POINT('Ctrl Pts',(-13.9553333333333,-0.738511305521624,
3.61820279633032));
#47257=CARTESIAN_POINT('Ctrl Pts',(-13.9553333333333,-0.849764871990641,
3.58155482781478));
#47258=CARTESIAN_POINT('Ctrl Pts',(-13.9553333333333,-0.957731897995734,
3.54598947656061));
#47259=CARTESIAN_POINT('Ctrl Pts',(-13.9553333333333,-1.06398233874069,
3.5056292399093));
#47260=CARTESIAN_POINT('Ctrl Pts',(-13.9553333333333,-1.16810511106794,
3.46046090716126));
#47261=CARTESIAN_POINT('Ctrl Pts',(-13.9553333333333,-1.23784694811165,
3.43020698257164));
#47262=CARTESIAN_POINT('Ctrl Pts',(-13.9553333333333,-1.30663363739179,
3.39779517970804));
#47263=CARTESIAN_POINT('Ctrl Pts',(-13.9553333333333,-1.37433213984351,
3.36321258891611));
#47264=CARTESIAN_POINT('Ctrl Pts',(-13.9553333333333,-1.40712864407733,
3.34645907082858));
#47265=CARTESIAN_POINT('Ctrl Pts',(-13.9553333333333,-1.43966963403488,
3.32919598381487));
#47266=CARTESIAN_POINT('Ctrl Pts',(-13.9553333333333,-1.47193922015119,
3.31142128892406));
#47267=CARTESIAN_POINT('Ctrl Pts',(-13.9553333333333,-1.48558859579644,
3.30390295613014));
#47268=CARTESIAN_POINT('Ctrl Pts',(-13.9553333333333,-1.49918555024823,
3.29629517051011));
#47269=CARTESIAN_POINT('Ctrl Pts',(-13.9553333333333,-1.51272211910769,
3.28860190887891));
#47270=CARTESIAN_POINT('Ctrl Pts',(-13.9553333333333,-1.60994673400505,
3.23334607505838));
#47271=CARTESIAN_POINT('Ctrl Pts',(-13.9553333333333,-1.70416783551671,
3.17362426881821));
#47272=CARTESIAN_POINT('Ctrl Pts',(-13.9553333333333,-1.79501394372711,
3.10946096733353));
#47273=CARTESIAN_POINT('Ctrl Pts',(-13.9553333333333,-1.84679517267689,
3.07288862901545));
#47274=CARTESIAN_POINT('Ctrl Pts',(-13.9553333333333,-1.8974793779626,3.03487255871099));
#47275=CARTESIAN_POINT('Ctrl Pts',(-13.9553333333333,-1.94699263852852,
2.99541163692221));
#47276=CARTESIAN_POINT('Ctrl Pts',(-13.9553333333333,-2.03553331123934,
2.9248467716511));
#47277=CARTESIAN_POINT('Ctrl Pts',(-13.9553333333333,-2.12033217628919,
2.84966300167236));
#47278=CARTESIAN_POINT('Ctrl Pts',(-13.9553333333333,-2.2012244629001,2.77024331980942));
#47279=CARTESIAN_POINT('Ctrl Pts',(-13.9553333333333,-2.28247472756623,
2.6904721767077));
#47280=CARTESIAN_POINT('Ctrl Pts',(-13.9553333333333,-2.35978409856056,
2.606426642024));
#47281=CARTESIAN_POINT('Ctrl Pts',(-13.9553333333333,-2.43293781738034,
2.51847398269812));
#47282=CARTESIAN_POINT('Ctrl Pts',(-13.9553333333333,-2.45500011328369,
2.49194850146709));
#47283=CARTESIAN_POINT('Ctrl Pts',(-13.9553333333333,-2.47668408288072,
2.46506755442072));
#47284=CARTESIAN_POINT('Ctrl Pts',(-13.9553333333333,-2.49798291570529,
2.43784103819821));
#47285=CARTESIAN_POINT('Ctrl Pts',(-13.9553333333333,-2.50883358180945,
2.42397052054389));
#47286=CARTESIAN_POINT('Ctrl Pts',(-13.9553333333333,-2.51958518129152,
2.41000901037187));
#47287=CARTESIAN_POINT('Ctrl Pts',(-13.9553333333333,-2.53022550926122,
2.39597302308478));
#47288=CARTESIAN_POINT('Ctrl Pts',(-13.9553333333333,-2.59749517874235,
2.30723551157832));
#47289=CARTESIAN_POINT('Ctrl Pts',(-13.9553333333333,-2.66042616738569,
2.21539127565337));
#47290=CARTESIAN_POINT('Ctrl Pts',(-13.9553333333333,-2.71889127549631,
2.12082239717396));
#47291=CARTESIAN_POINT('Ctrl Pts',(-13.9553333333333,-2.77741263197492,
2.02616253545261));
#47292=CARTESIAN_POINT('Ctrl Pts',(-13.9553333333333,-2.83145977799374,
1.92877187196212));
#47293=CARTESIAN_POINT('Ctrl Pts',(-13.9553333333333,-2.88085709477908,
1.82901312880459));
#47294=CARTESIAN_POINT('Ctrl Pts',(-13.9553333333333,-2.92964767956841,
1.73047969149956));
#47295=CARTESIAN_POINT('Ctrl Pts',(-13.9553333333333,-2.97390210276449,
1.62963512353767));
#47296=CARTESIAN_POINT('Ctrl Pts',(-13.9553333333333,-3.01340139041157,
1.52682226668093));
#47297=CARTESIAN_POINT('Ctrl Pts',(-13.9553333333333,-3.03691137670684,
1.46562802750184));
#47298=CARTESIAN_POINT('Ctrl Pts',(-13.9553333333333,-3.05873583260475,
1.4037364305582));
#47299=CARTESIAN_POINT('Ctrl Pts',(-13.9553333333333,-3.07881973126231,
1.34122049792282));
#47300=CARTESIAN_POINT('Ctrl Pts',(-13.9553333333333,-3.08803506168237,
1.31253558043859));
#47301=CARTESIAN_POINT('Ctrl Pts',(-13.9553333333333,-3.0968838486815,1.28371923382974));
#47302=CARTESIAN_POINT('Ctrl Pts',(-13.9553333333333,-3.10536029103769,
1.25477861820457));
#47303=CARTESIAN_POINT('Ctrl Pts',(-13.9553333333333,-3.10926402172898,
1.24145034147085));
#47304=CARTESIAN_POINT('Ctrl Pts',(-13.9553333333333,-3.11308820868124,
1.22809751314922));
#47305=CARTESIAN_POINT('Ctrl Pts',(-13.9553333333333,-3.11682997167633,
1.21472968520499));
#47306=CARTESIAN_POINT('Ctrl Pts',(-13.9553333333333,-3.14582478574141,
1.11114277010499));
#47307=CARTESIAN_POINT('Ctrl Pts',(-13.9553333333333,-3.16991857070316,
1.00650635296175));
#47308=CARTESIAN_POINT('Ctrl Pts',(-13.9553333333333,-3.18895492093138,
0.901150303424905));
#47309=CARTESIAN_POINT('Ctrl Pts',(-13.9553333333333,-3.20772681944474,
0.797257853140867));
#47310=CARTESIAN_POINT('Ctrl Pts',(-13.9553333333333,-3.22158089463548,
0.692664846008168));
#47311=CARTESIAN_POINT('Ctrl Pts',(-13.9553333333333,-3.23031744579328,
0.587688020009249));
#47312=CARTESIAN_POINT('Ctrl Pts',(-13.9553333333333,-3.2387841631479,0.485953468414905));
#47313=CARTESIAN_POINT('Ctrl Pts',(-13.9553333333333,-3.24244450620772,
0.383857830419708));
#47314=CARTESIAN_POINT('Ctrl Pts',(-13.9553333333333,-3.24107000631815,
0.281699843730534));
#47315=CARTESIAN_POINT('Ctrl Pts',(-13.9553333333333,-3.23974122264024,
0.182939657345128));
#47316=CARTESIAN_POINT('Ctrl Pts',(-13.9553333333333,-3.23370683694308,
0.0841207460689442));
#47317=CARTESIAN_POINT('Ctrl Pts',(-13.9553333333333,-3.22271751746272,
-0.0144694553766564));
#47318=CARTESIAN_POINT('Ctrl Pts',(-26.6770630286919,-1.43290239521325,
2.88667772504866));
#47319=CARTESIAN_POINT('Ctrl Pts',(-26.6108040198619,-2.39432226019554,
2.40944370083299));
#47320=CARTESIAN_POINT('Ctrl Pts',(-26.478286002202,-3.78590739708692,0.426683950034108));
#47321=CARTESIAN_POINT('Ctrl Pts',(-26.2795089757119,-2.40485858874901,
-2.95981954148459));
#47322=CARTESIAN_POINT('Ctrl Pts',(-26.080731949222,1.18722242799118,-3.6205134943868));
#47323=CARTESIAN_POINT('Ctrl Pts',(-25.881954922732,3.68771187601412,-0.961936478150598));
#47324=CARTESIAN_POINT('Ctrl Pts',(-25.683177896242,2.80382800818523,2.58188775682714));
#47325=CARTESIAN_POINT('Ctrl Pts',(-25.4844008697521,-0.654391852565681,
3.75444098441731));
#47326=CARTESIAN_POINT('Ctrl Pts',(-25.2856238432621,-3.51165133563114,
1.48105475903402));
#47327=CARTESIAN_POINT('Ctrl Pts',(-25.0868468167721,-3.14538674562905,
-2.15222056121083));
#47328=CARTESIAN_POINT('Ctrl Pts',(-24.8880697902821,0.108362070287417,
-3.80963202337103));
#47329=CARTESIAN_POINT('Ctrl Pts',(-24.6892927637921,3.26260339792463,-1.96993487649339));
#47330=CARTESIAN_POINT('Ctrl Pts',(-24.4905157373022,3.42183734109356,1.67817626036435));
#47331=CARTESIAN_POINT('Ctrl Pts',(-24.2917387108122,0.439863865693541,
3.78572376365049));
#47332=CARTESIAN_POINT('Ctrl Pts',(-24.0929616843222,-2.94589400020572,
2.41804089343147));
#47333=CARTESIAN_POINT('Ctrl Pts',(-23.8941846578322,-3.62736475341514,
-1.16937531657263));
#47334=CARTESIAN_POINT('Ctrl Pts',(-23.6954076313422,-0.978964290720696,
-3.68331844135819));
#47335=CARTESIAN_POINT('Ctrl Pts',(-23.4966306048523,2.56811106183178,-2.81602834885952));
#47336=CARTESIAN_POINT('Ctrl Pts',(-23.2978535783623,3.75769675477037,0.636337094806224));
#47337=CARTESIAN_POINT('Ctrl Pts',(-23.0990765518723,1.49776930770217,3.50455359875708));
#47338=CARTESIAN_POINT('Ctrl Pts',(-22.9002995253823,-2.13708929630228,
3.15563920390215));
#47339=CARTESIAN_POINT('Ctrl Pts',(-22.7015224988924,-3.81012990972458,
-0.0901078773958003));
#47340=CARTESIAN_POINT('Ctrl Pts',(-22.5027454724024,-1.9855246223874,-3.2531371345379));
#47341=CARTESIAN_POINT('Ctrl Pts',(-22.3039684459124,1.66176444014233,-3.4298321060602));
#47342=CARTESIAN_POINT('Ctrl Pts',(-22.1051914194224,3.78357703340158,-0.45798924048176));
#47343=CARTESIAN_POINT('Ctrl Pts',(-21.9064143929325,2.43211891370082,2.93428132400969));
#47344=CARTESIAN_POINT('Ctrl Pts',(-21.7076373664425,-1.15199029393737,
3.63292274535707));
#47345=CARTESIAN_POINT('Ctrl Pts',(-21.5088603399525,-3.67858855159617,
0.996591980611707));
#47346=CARTESIAN_POINT('Ctrl Pts',(-21.3100833134625,-2.8282940543877,-2.5545962593447));
#47347=CARTESIAN_POINT('Ctrl Pts',(-21.1113062869725,0.618334760982468,
-3.76070092288226));
#47348=CARTESIAN_POINT('Ctrl Pts',(-20.9125292604826,3.49734092856599,-1.51453482522831));
#47349=CARTESIAN_POINT('Ctrl Pts',(-20.7137522339926,3.16583712036473,2.12195302366768));
#47350=CARTESIAN_POINT('Ctrl Pts',(-20.5149752075026,-0.0718608118791213,
3.81051772482967));
#47351=CARTESIAN_POINT('Ctrl Pts',(-20.3161981810126,-3.24359152557454,
2.00108053877585));
#47352=CARTESIAN_POINT('Ctrl Pts',(-20.1174211545227,-3.43775066054039,
-1.64532054733392));
#47353=CARTESIAN_POINT('Ctrl Pts',(-19.9186441280327,-0.476102850960359,
-3.7813404214166));
#47354=CARTESIAN_POINT('Ctrl Pts',(-19.7198671015427,2.92260070569343,-2.44614276413548));
#47355=CARTESIAN_POINT('Ctrl Pts',(-19.5210900750527,3.63839775937779,1.13457968101029));
#47356=CARTESIAN_POINT('Ctrl Pts',(-19.3223130485627,1.01419664261627,3.67377387388617));
#47357=CARTESIAN_POINT('Ctrl Pts',(-19.1235360220728,-2.54102278309695,
2.84049511943538));
#47358=CARTESIAN_POINT('Ctrl Pts',(-18.9247589955828,-3.76361889362955,
-0.600318361016281));
#47359=CARTESIAN_POINT('Ctrl Pts',(-18.7259819690928,-1.53126558554944,
-3.49004799470226));
#47360=CARTESIAN_POINT('Ctrl Pts',(-18.5272049426028,2.10676807472235,-3.17596246694));
#47361=CARTESIAN_POINT('Ctrl Pts',(-18.3284279161128,3.81081816296161,0.0536121173318595));
#47362=CARTESIAN_POINT('Ctrl Pts',(-18.1296508896229,2.01659055559616,3.23397151708182));
#47363=CARTESIAN_POINT('Ctrl Pts',(-17.9308738631329,-1.62883890977077,
3.44559039419421));
#47364=CARTESIAN_POINT('Ctrl Pts',(-17.7320968366429,-3.77901711469435,
0.4942055163807));
#47365=CARTESIAN_POINT('Ctrl Pts',(-17.5333198101529,-2.46011047524903,
-2.91085301505003));
#47366=CARTESIAN_POINT('Ctrl Pts',(-17.334542783663,1.11714296776071,-3.64378942704172));
#47367=CARTESIAN_POINT('Ctrl Pts',(-17.135765757173,3.66887510281969,-1.03177786727233));
#47368=CARTESIAN_POINT('Ctrl Pts',(-16.936988730683,2.85263073953649,2.52739068741007));
#47369=CARTESIAN_POINT('Ctrl Pts',(-16.738211704193,-0.582287604380603,
3.76645122510734));
#47370=CARTESIAN_POINT('Ctrl Pts',(-16.539434677703,-3.48267616710018,1.54795992773304));
#47371=CARTESIAN_POINT('Ctrl Pts',(-16.3406576512131,-3.18601276291149,
-2.09153228748111));
#47372=CARTESIAN_POINT('Ctrl Pts',(-16.1418806247231,0.0353578955585694,
-3.81103610176739));
#47373=CARTESIAN_POINT('Ctrl Pts',(-15.9431035982331,3.22428567725235,-2.0320448374088));
#47374=CARTESIAN_POINT('Ctrl Pts',(-15.7443265717431,3.45333495329863,1.6123015202179));
#47375=CARTESIAN_POINT('Ctrl Pts',(-15.5455495452532,0.512328175864222,
3.77664281656251));
#47376=CARTESIAN_POINT('Ctrl Pts',(-15.3467725187632,-2.89909931249566,
2.47395260233185));
#47377=CARTESIAN_POINT('Ctrl Pts',(-15.1479954922732,-3.64897975376042,
-1.09954652417408));
#47378=CARTESIAN_POINT('Ctrl Pts',(-14.9492184657832,-1.04956382363505,
-3.66415224416977));
#47379=CARTESIAN_POINT('Ctrl Pts',(-14.7504414392933,2.51414376359986,-2.86419653732846));
#47380=CARTESIAN_POINT('Ctrl Pts',(-14.5516644128032,3.76833505696647,0.563263663837553));
#47381=CARTESIAN_POINT('Ctrl Pts',(-14.3528873863133,1.56631945652084,3.47714249206992));
#47382=CARTESIAN_POINT('Ctrl Pts',(-14.1541103598233,-2.07983560379109,
3.19208989123696));
#47383=CARTESIAN_POINT('Ctrl Pts',(-14.0215923421633,-3.22753662896723,
1.05886984177777));
#47384=CARTESIAN_POINT('Ctrl Pts',(-13.9553333333333,-3.22271751746272,
-0.0144694553766564));
#47385=CARTESIAN_POINT('Ctrl Pts',(-26.5403753524613,-1.53816642191923,
3.09873914818272));
#47386=CARTESIAN_POINT('Ctrl Pts',(-26.4741163436313,-2.57021421430345,
2.58644650780599));
#47387=CARTESIAN_POINT('Ctrl Pts',(-26.3415983259713,-4.06402812511743,
0.45802905132047));
#47388=CARTESIAN_POINT('Ctrl Pts',(-26.1428212994813,-2.58152456373508,
-3.17725411644275));
#47389=CARTESIAN_POINT('Ctrl Pts',(-25.9440442729914,1.27443828706397,-3.88648403811378));
#47390=CARTESIAN_POINT('Ctrl Pts',(-25.7452672465014,3.95861895433119,-1.03260235704353));
#47391=CARTESIAN_POINT('Ctrl Pts',(-25.5464902200114,3.00980311669128,2.77155866720764));
#47392=CARTESIAN_POINT('Ctrl Pts',(-25.3477131935214,-0.702464855775631,
4.03025012352547));
#47393=CARTESIAN_POINT('Ctrl Pts',(-25.1489361670314,-3.76962463598353,
1.58985615976362));
#47394=CARTESIAN_POINT('Ctrl Pts',(-24.9501591405415,-3.37645347808664,
-2.31032721480376));
#47395=CARTESIAN_POINT('Ctrl Pts',(-24.7513821140515,0.116322576110241,
-4.08949561239689));
#47396=CARTESIAN_POINT('Ctrl Pts',(-24.5526050875615,3.50228111244131,-2.11465043991279));
#47397=CARTESIAN_POINT('Ctrl Pts',(-24.3538280610715,3.6732127163178,1.80145862159038));
#47398=CARTESIAN_POINT('Ctrl Pts',(-24.1550510345815,0.472177191332509,
4.06383100158214));
#47399=CARTESIAN_POINT('Ctrl Pts',(-23.9562740080916,-3.16230557558347,
2.59567526827282));
#47400=CARTESIAN_POINT('Ctrl Pts',(-23.7574969816016,-3.8938386050546,-1.2552800892663));
#47401=CARTESIAN_POINT('Ctrl Pts',(-23.5587199551116,-1.05088106857445,
-3.95390276871574));
#47402=CARTESIAN_POINT('Ctrl Pts',(-23.3599429286216,2.75676990719324,-3.02289972007743));
#47403=CARTESIAN_POINT('Ctrl Pts',(-23.1611659021316,4.03374506962317,0.683083757499677));
#47404=CARTESIAN_POINT('Ctrl Pts',(-22.9623888756417,1.60779859436684,3.76200548441552));
#47405=CARTESIAN_POINT('Ctrl Pts',(-22.7636118491517,-2.2940843753185,3.38745910352944));
#47406=CARTESIAN_POINT('Ctrl Pts',(-22.5648348226617,-4.09003007453019,
-0.0967273917774301));
#47407=CARTESIAN_POINT('Ctrl Pts',(-22.3660577961717,-2.13138544136196,
-3.49211943741645));
#47408=CARTESIAN_POINT('Ctrl Pts',(-22.1672807696818,1.78384115450232,-3.68179479355063));
#47409=CARTESIAN_POINT('Ctrl Pts',(-21.9685037431918,4.06152656800954,-0.49163409431284));
#47410=CARTESIAN_POINT('Ctrl Pts',(-21.7697267167018,2.61078748955023,3.1498398077454));
#47411=CARTESIAN_POINT('Ctrl Pts',(-21.5709496902119,-1.23661792626678,
3.89980489878606));
#47412=CARTESIAN_POINT('Ctrl Pts',(-21.3721726637218,-3.94882541129375,
1.06980372567722));
#47413=CARTESIAN_POINT('Ctrl Pts',(-21.1733956372319,-3.03606649015725,
-2.74226227886213));
#47414=CARTESIAN_POINT('Ctrl Pts',(-20.9746186107419,0.66375893433211,-4.03696993024938));
#47415=CARTESIAN_POINT('Ctrl Pts',(-20.7758415842519,3.75426295628702,-1.62579574210764));
#47416=CARTESIAN_POINT('Ctrl Pts',(-20.5770645577619,3.39840618040549,2.27783616022909));
#47417=CARTESIAN_POINT('Ctrl Pts',(-20.378287531272,-0.0771398584115342,
4.09044637934939));
#47418=CARTESIAN_POINT('Ctrl Pts',(-20.179510504782,-3.48187258792183,2.14808412811888));
#47419=CARTESIAN_POINT('Ctrl Pts',(-19.980733478292,-3.69029506171422,-1.76618925870813));
#47420=CARTESIAN_POINT('Ctrl Pts',(-19.781956451802,-0.51107836875259,-4.05912564979931));
#47421=CARTESIAN_POINT('Ctrl Pts',(-19.583179425312,3.1373011066159,-2.62584156156287));
#47422=CARTESIAN_POINT('Ctrl Pts',(-19.3844023988221,3.90568211886354,1.21792829305873));
#47423=CARTESIAN_POINT('Ctrl Pts',(-19.1856253723321,1.08870166321652,3.94365703722262));
#47424=CARTESIAN_POINT('Ctrl Pts',(-18.9868483458421,-2.72769166647238,
3.04916387113078));
#47425=CARTESIAN_POINT('Ctrl Pts',(-18.7880713193521,-4.0401022612711,-0.644419011693669));
#47426=CARTESIAN_POINT('Ctrl Pts',(-18.5892942928622,-1.64375557930598,
-3.74643426814753));
#47427=CARTESIAN_POINT('Ctrl Pts',(-18.3905172663722,2.26153569296468,-3.40927535625753));
#47428=CARTESIAN_POINT('Ctrl Pts',(-18.1917402398822,4.09076888829903,0.057550576343037));
#47429=CARTESIAN_POINT('Ctrl Pts',(-17.9929632133922,2.16473354342874,3.47154587335181));
#47430=CARTESIAN_POINT('Ctrl Pts',(-17.7941861869023,-1.74849684535007,
3.69871071870759));
#47431=CARTESIAN_POINT('Ctrl Pts',(-17.5954091604123,-4.05663166807388,
0.530510894087064));
#47432=CARTESIAN_POINT('Ctrl Pts',(-17.3966321339223,-2.64083537014167,
-3.12469040588489));
#47433=CARTESIAN_POINT('Ctrl Pts',(-17.1978551074323,1.19921064214355,-3.91146986978538));
#47434=CARTESIAN_POINT('Ctrl Pts',(-16.9990780809423,3.93839839211999,-1.10757444165036));
#47435=CARTESIAN_POINT('Ctrl Pts',(-16.8003010544524,3.06219099943418,2.71305812833607));
#47436=CARTESIAN_POINT('Ctrl Pts',(-16.6015240279624,-0.625063677714576,
4.04314266178228));
#47437=CARTESIAN_POINT('Ctrl Pts',(-16.4027470014724,-3.73852089056956,
1.66167632301373));
#47438=CARTESIAN_POINT('Ctrl Pts',(-16.2039699749824,-3.42006396813043,
-2.24518065271611));
#47439=CARTESIAN_POINT('Ctrl Pts',(-16.0051929484924,0.0379553610068489,
-4.09100283734831));
#47440=CARTESIAN_POINT('Ctrl Pts',(-15.8064159220025,3.46114849133643,-2.18132312931992));
#47441=CARTESIAN_POINT('Ctrl Pts',(-15.6076388955125,3.70702420942879,1.73074458434373));
#47442=CARTESIAN_POINT('Ctrl Pts',(-15.4088618690225,0.549964882290692,
4.05408294900256));
#47443=CARTESIAN_POINT('Ctrl Pts',(-15.2100848425325,-3.11207325159528,
2.65569436902244));
#47444=CARTESIAN_POINT('Ctrl Pts',(-15.0113078160426,-3.91704148883227,
-1.18032152676447));
#47445=CARTESIAN_POINT('Ctrl Pts',(-14.8125307895526,-1.12666699181305,
-3.93332858233041));
#47446=CARTESIAN_POINT('Ctrl Pts',(-14.6137537630626,2.69883805761343,-3.07460644508194));
#47447=CARTESIAN_POINT('Ctrl Pts',(-14.4149767365726,4.0451648838959,0.604642198447279));
#47448=CARTESIAN_POINT('Ctrl Pts',(-14.2161997100826,1.68138458143942,3.73258070012128));
#47449=CARTESIAN_POINT('Ctrl Pts',(-14.0174226835927,-2.23262470601667,
3.42658753509713));
#47450=CARTESIAN_POINT('Ctrl Pts',(-13.8849046659327,-3.46463826480867,
1.13665664964091));
#47451=CARTESIAN_POINT('Ctrl Pts',(-13.8186456571027,-3.45946513122715,
-0.015532412031805));
#47452=CARTESIAN_POINT('Ctrl Pts',(-26.4036876762306,-1.64343044862521,
3.31080057131678));
#47453=CARTESIAN_POINT('Ctrl Pts',(-26.3374286674006,-2.74610616841136,
2.76344931477899));
#47454=CARTESIAN_POINT('Ctrl Pts',(-26.2049106497407,-4.34214885314794,
0.489374152606833));
#47455=CARTESIAN_POINT('Ctrl Pts',(-26.0061336232507,-2.75819053872115,
-3.39468869140092));
#47456=CARTESIAN_POINT('Ctrl Pts',(-25.8073565967607,1.36165414613677,-4.15245458184075));
#47457=CARTESIAN_POINT('Ctrl Pts',(-25.6085795702707,4.22952603264826,-1.10326823593646));
#47458=CARTESIAN_POINT('Ctrl Pts',(-25.4098025437808,3.21577822519734,2.96122957758815));
#47459=CARTESIAN_POINT('Ctrl Pts',(-25.2110255172908,-0.750537858985583,
4.30605926263362));
#47460=CARTESIAN_POINT('Ctrl Pts',(-25.0122484908008,-4.02759793633592,
1.69865756049324));
#47461=CARTESIAN_POINT('Ctrl Pts',(-24.8134714643108,-3.60752021054423,
-2.4684338683967));
#47462=CARTESIAN_POINT('Ctrl Pts',(-24.6146944378208,0.124283081933059,
-4.36935920142275));
#47463=CARTESIAN_POINT('Ctrl Pts',(-24.4159174113308,3.74195882695799,-2.25936600333218));
#47464=CARTESIAN_POINT('Ctrl Pts',(-24.2171403848409,3.92458809154204,1.92474098281642));
#47465=CARTESIAN_POINT('Ctrl Pts',(-24.0183633583509,0.504490516971484,
4.3419382395138));
#47466=CARTESIAN_POINT('Ctrl Pts',(-23.8195863318609,-3.37871715096123,
2.77330964311416));
#47467=CARTESIAN_POINT('Ctrl Pts',(-23.620809305371,-4.16031245669405,-1.34118486195997));
#47468=CARTESIAN_POINT('Ctrl Pts',(-23.4220322788809,-1.1227978464282,-4.22448709607329));
#47469=CARTESIAN_POINT('Ctrl Pts',(-23.223255252391,2.9454287525547,-3.22977109129534));
#47470=CARTESIAN_POINT('Ctrl Pts',(-23.024478225901,4.30979338447599,0.729830420193126));
#47471=CARTESIAN_POINT('Ctrl Pts',(-22.825701199411,1.71782788103149,4.01945737007395));
#47472=CARTESIAN_POINT('Ctrl Pts',(-22.6269241729211,-2.45107945433472,
3.61927900315673));
#47473=CARTESIAN_POINT('Ctrl Pts',(-22.4281471464311,-4.36993023933581,
-0.103346906159059));
#47474=CARTESIAN_POINT('Ctrl Pts',(-22.2293701199411,-2.27724626033652,
-3.73110174029499));
#47475=CARTESIAN_POINT('Ctrl Pts',(-22.0305930934511,1.90591786886231,-3.93375748104105));
#47476=CARTESIAN_POINT('Ctrl Pts',(-21.8318160669612,4.33947610261751,-0.525278948143918));
#47477=CARTESIAN_POINT('Ctrl Pts',(-21.6330390404711,2.78945606539964,3.36539829148111));
#47478=CARTESIAN_POINT('Ctrl Pts',(-21.4342620139812,-1.32124555859619,
4.16668705221506));
#47479=CARTESIAN_POINT('Ctrl Pts',(-21.2354849874912,-4.21906227099134,
1.14301547074272));
#47480=CARTESIAN_POINT('Ctrl Pts',(-21.0367079610012,-3.2438389259268,-2.92992829837957));
#47481=CARTESIAN_POINT('Ctrl Pts',(-20.8379309345113,0.709183107681748,
-4.3132389376165));
#47482=CARTESIAN_POINT('Ctrl Pts',(-20.6391539080213,4.01118498400806,-1.73705665898696));
#47483=CARTESIAN_POINT('Ctrl Pts',(-20.4403768815313,3.63097524044626,2.4337192967905));
#47484=CARTESIAN_POINT('Ctrl Pts',(-20.2415998550413,-0.0824189049439472,
4.37037503386911));
#47485=CARTESIAN_POINT('Ctrl Pts',(-20.0428228285513,-3.72015365026912,
2.2950877174619));
#47486=CARTESIAN_POINT('Ctrl Pts',(-19.8440458020614,-3.94283946288805,
-1.88705797008235));
#47487=CARTESIAN_POINT('Ctrl Pts',(-19.6452687755714,-0.546053886544821,
-4.33691087818202));
#47488=CARTESIAN_POINT('Ctrl Pts',(-19.4464917490814,3.35200150753837,-2.80554035899026));
#47489=CARTESIAN_POINT('Ctrl Pts',(-19.2477147225914,4.17296647834929,1.30127690510718));
#47490=CARTESIAN_POINT('Ctrl Pts',(-19.0489376961014,1.16320668381677,4.21354020055907));
#47491=CARTESIAN_POINT('Ctrl Pts',(-18.8501606696115,-2.91436054984781,
3.25783262282619));
#47492=CARTESIAN_POINT('Ctrl Pts',(-18.6513836431215,-4.31658562891265,
-0.688519662371059));
#47493=CARTESIAN_POINT('Ctrl Pts',(-18.4526066166315,-1.75624557306252,
-4.00282054159279));
#47494=CARTESIAN_POINT('Ctrl Pts',(-18.2538295901415,2.41630331120702,-3.64258824557506));
#47495=CARTESIAN_POINT('Ctrl Pts',(-18.0550525636516,4.37071961363644,0.0614890353542112));
#47496=CARTESIAN_POINT('Ctrl Pts',(-17.8562755371616,2.31287653126131,3.70912022962179));
#47497=CARTESIAN_POINT('Ctrl Pts',(-17.6574985106716,-1.86815478092937,
3.95183104322097));
#47498=CARTESIAN_POINT('Ctrl Pts',(-17.4587214841817,-4.33424622145341,
0.566816271793429));
#47499=CARTESIAN_POINT('Ctrl Pts',(-17.2599444576916,-2.82156026503431,
-3.33852779671976));
#47500=CARTESIAN_POINT('Ctrl Pts',(-17.0611674312017,1.28127831652639,-4.17915031252904));
#47501=CARTESIAN_POINT('Ctrl Pts',(-16.8623904047117,4.20792168142029,-1.18337101602838));
#47502=CARTESIAN_POINT('Ctrl Pts',(-16.6636133782217,3.27175125933188,2.89872556926209));
#47503=CARTESIAN_POINT('Ctrl Pts',(-16.4648363517317,-0.667839751048547,
4.31983409845722));
#47504=CARTESIAN_POINT('Ctrl Pts',(-16.2660593252418,-3.99436561403894,
1.77539271829442));
#47505=CARTESIAN_POINT('Ctrl Pts',(-16.0672822987518,-3.65411517334937,
-2.39882901795111));
#47506=CARTESIAN_POINT('Ctrl Pts',(-15.8685052722618,0.040552826455128,
-4.37096957292924));
#47507=CARTESIAN_POINT('Ctrl Pts',(-15.6697282457718,3.69801130542051,-2.33060142123105));
#47508=CARTESIAN_POINT('Ctrl Pts',(-15.4709512192819,3.96071346555895,1.84918764846957));
#47509=CARTESIAN_POINT('Ctrl Pts',(-15.2721741927919,0.587601588717162,
4.33152308144261));
#47510=CARTESIAN_POINT('Ctrl Pts',(-15.0733971663019,-3.32504719069491,
2.83743613571303));
#47511=CARTESIAN_POINT('Ctrl Pts',(-14.8746201398119,-4.18510322390412,
-1.26109652935485));
#47512=CARTESIAN_POINT('Ctrl Pts',(-14.6758431133219,-1.20377015999105,
-4.20250492049104));
#47513=CARTESIAN_POINT('Ctrl Pts',(-14.477066086832,2.883532351627,-3.28501635283543));
#47514=CARTESIAN_POINT('Ctrl Pts',(-14.278289060342,4.32199471082533,0.646020733057002));
#47515=CARTESIAN_POINT('Ctrl Pts',(-14.079512033852,1.796449706358,3.98801890817264));
#47516=CARTESIAN_POINT('Ctrl Pts',(-13.880735007362,-2.38541380824225,3.6610851789573));
#47517=CARTESIAN_POINT('Ctrl Pts',(-13.748216989702,-3.7017399006501,1.21444345750405));
#47518=CARTESIAN_POINT('Ctrl Pts',(-13.681957980872,-3.69621274499157,-0.0165953686869537));
#47519=CARTESIAN_POINT('Ctrl Pts',(-26.267,-1.7486944753312,3.52286199445084));
#47520=CARTESIAN_POINT('Ctrl Pts',(-26.20074099117,-2.92199812251927,2.94045212175199));
#47521=CARTESIAN_POINT('Ctrl Pts',(-26.06822297351,-4.62026958117845,0.520719253893197));
#47522=CARTESIAN_POINT('Ctrl Pts',(-25.86944594702,-2.93485651370723,-3.6121232663591));
#47523=CARTESIAN_POINT('Ctrl Pts',(-25.6706689205301,1.44887000520957,-4.41842512556771));
#47524=CARTESIAN_POINT('Ctrl Pts',(-25.4718918940401,4.50043311096533,-1.1739341148294));
#47525=CARTESIAN_POINT('Ctrl Pts',(-25.2731148675501,3.42175333370339,3.15090048796866));
#47526=CARTESIAN_POINT('Ctrl Pts',(-25.0743378410601,-0.798610862195538,
4.58186840174178));
#47527=CARTESIAN_POINT('Ctrl Pts',(-24.8755608145702,-4.2855712366883,1.80745896122284));
#47528=CARTESIAN_POINT('Ctrl Pts',(-24.6767837880802,-3.83858694300183,
-2.62654052198963));
#47529=CARTESIAN_POINT('Ctrl Pts',(-24.4780067615902,0.132243587755882,
-4.64922279044861));
#47530=CARTESIAN_POINT('Ctrl Pts',(-24.2792297351002,3.98163654147467,-2.40408156675157));
#47531=CARTESIAN_POINT('Ctrl Pts',(-24.0804527086102,4.17596346676628,2.04802334404246));
#47532=CARTESIAN_POINT('Ctrl Pts',(-23.8816756821203,0.536803842610455,
4.62004547744546));
#47533=CARTESIAN_POINT('Ctrl Pts',(-23.6828986556303,-3.59512872633899,
2.9509440179555));
#47534=CARTESIAN_POINT('Ctrl Pts',(-23.4841216291403,-4.42678630833351,
-1.42708963465364));
#47535=CARTESIAN_POINT('Ctrl Pts',(-23.2853446026503,-1.19471462428195,
-4.49507142343084));
#47536=CARTESIAN_POINT('Ctrl Pts',(-23.0865675761604,3.13408759791616,-3.43664246251325));
#47537=CARTESIAN_POINT('Ctrl Pts',(-22.8877905496704,4.58584169932879,0.776577082886578));
#47538=CARTESIAN_POINT('Ctrl Pts',(-22.6890135231804,1.82785716769616,4.27690925573239));
#47539=CARTESIAN_POINT('Ctrl Pts',(-22.4902364966904,-2.60807453335094,
3.85109890278403));
#47540=CARTESIAN_POINT('Ctrl Pts',(-22.2914594702004,-4.64983040414143,
-0.109966420540693));
#47541=CARTESIAN_POINT('Ctrl Pts',(-22.0926824437105,-2.42310707931108,
-3.97008404317354));
#47542=CARTESIAN_POINT('Ctrl Pts',(-21.8939054172205,2.02799458322229,-4.18572016853148));
#47543=CARTESIAN_POINT('Ctrl Pts',(-21.6951283907305,4.61742563722547,-0.558923801975));
#47544=CARTESIAN_POINT('Ctrl Pts',(-21.4963513642405,2.96812464124906,3.58095677521683));
#47545=CARTESIAN_POINT('Ctrl Pts',(-21.2975743377506,-1.40587319092561,
4.43356920564406));
#47546=CARTESIAN_POINT('Ctrl Pts',(-21.0987973112605,-4.48929913068892,
1.21622721580824));
#47547=CARTESIAN_POINT('Ctrl Pts',(-20.9000202847706,-3.45161136169635,
-3.11759431789701));
#47548=CARTESIAN_POINT('Ctrl Pts',(-20.7012432582806,0.754607281031384,
-4.58950794498361));
#47549=CARTESIAN_POINT('Ctrl Pts',(-20.5024662317907,4.2681070117291,-1.84831757586629));
#47550=CARTESIAN_POINT('Ctrl Pts',(-20.3036892053006,3.86354430048703,2.58960243335191));
#47551=CARTESIAN_POINT('Ctrl Pts',(-20.1049121788107,-0.0876979514763586,
4.65030368838883));
#47552=CARTESIAN_POINT('Ctrl Pts',(-19.9061351523207,-3.95843471261642,
2.44209130680492));
#47553=CARTESIAN_POINT('Ctrl Pts',(-19.7073581258307,-4.19538386406187,
-2.00792668145656));
#47554=CARTESIAN_POINT('Ctrl Pts',(-19.5085810993407,-0.581029404337056,
-4.61469610656473));
#47555=CARTESIAN_POINT('Ctrl Pts',(-19.3098040728508,3.56670190846084,-2.98523915641764));
#47556=CARTESIAN_POINT('Ctrl Pts',(-19.1110270463608,4.44025083783504,1.38462551715563));
#47557=CARTESIAN_POINT('Ctrl Pts',(-18.9122500198708,1.23771170441702,4.48342336389552));
#47558=CARTESIAN_POINT('Ctrl Pts',(-18.7134729933808,-3.10102943322324,
3.46650137452159));
#47559=CARTESIAN_POINT('Ctrl Pts',(-18.5146959668909,-4.59306899655421,
-0.732620313048447));
#47560=CARTESIAN_POINT('Ctrl Pts',(-18.3159189404009,-1.86873556681905,
-4.25920681503806));
#47561=CARTESIAN_POINT('Ctrl Pts',(-18.1171419139109,2.57107092944934,-3.87590113489259));
#47562=CARTESIAN_POINT('Ctrl Pts',(-17.9183648874209,4.65067033897386,0.0654274943653892));
#47563=CARTESIAN_POINT('Ctrl Pts',(-17.7195878609309,2.46101951909389,3.94669458589177));
#47564=CARTESIAN_POINT('Ctrl Pts',(-17.520810834441,-1.98781271650867,4.20495136773435));
#47565=CARTESIAN_POINT('Ctrl Pts',(-17.322033807951,-4.61186077483295,0.60312164949979));
#47566=CARTESIAN_POINT('Ctrl Pts',(-17.123256781461,-3.00228515992694,-3.55236518755462));
#47567=CARTESIAN_POINT('Ctrl Pts',(-16.924479754971,1.36334599090922,-4.4468307552727));
#47568=CARTESIAN_POINT('Ctrl Pts',(-16.725702728481,4.4774449707206,-1.25916759040641));
#47569=CARTESIAN_POINT('Ctrl Pts',(-16.5269257019911,3.48131151922957,3.0843930101881));
#47570=CARTESIAN_POINT('Ctrl Pts',(-16.3281486755011,-0.710615824382518,
4.59652553513216));
#47571=CARTESIAN_POINT('Ctrl Pts',(-16.1293716490111,-4.25021033750832,
1.88910911357511));
#47572=CARTESIAN_POINT('Ctrl Pts',(-15.9305946225211,-3.8881663785683,-2.55247738318612));
#47573=CARTESIAN_POINT('Ctrl Pts',(-15.7318175960312,0.0431502919034069,
-4.65093630851017));
#47574=CARTESIAN_POINT('Ctrl Pts',(-15.5330405695412,3.93487411950459,-2.47987971314217));
#47575=CARTESIAN_POINT('Ctrl Pts',(-15.3342635430512,4.21440272168911,1.9676307125954));
#47576=CARTESIAN_POINT('Ctrl Pts',(-15.1354865165612,0.625238295143632,
4.60896321388266));
#47577=CARTESIAN_POINT('Ctrl Pts',(-14.9367094900712,-3.53802112979453,
3.01917790240362));
#47578=CARTESIAN_POINT('Ctrl Pts',(-14.7379324635813,-4.45316495897597,
-1.34187153194524));
#47579=CARTESIAN_POINT('Ctrl Pts',(-14.5391554370913,-1.28087332816905,
-4.47168125865167));
#47580=CARTESIAN_POINT('Ctrl Pts',(-14.3403784106013,3.06822664564056,-3.49542626058891));
#47581=CARTESIAN_POINT('Ctrl Pts',(-14.1416013841113,4.59882453775476,0.687399267666724));
#47582=CARTESIAN_POINT('Ctrl Pts',(-13.9428243576214,1.91151483127657,4.24345711622401));
#47583=CARTESIAN_POINT('Ctrl Pts',(-13.7440473311314,-2.53820291046783,
3.89558282281748));
#47584=CARTESIAN_POINT('Ctrl Pts',(-13.6115293134714,-3.93884153649153,
1.29223026536719));
#47585=CARTESIAN_POINT('Ctrl Pts',(-13.5452703046414,-3.932960358756,-0.0176583253421023));
#47586=CARTESIAN_POINT('Ctrl Pts',(-14.796163522035,-3.93066717675506,-0.00339337507098336));
#47587=CARTESIAN_POINT('Ctrl Pts',(-14.7767531692171,-3.93387125603329,
-0.387580586707519));
#47588=CARTESIAN_POINT('Ctrl Pts',(-14.7573428163992,-3.88212968630794,
-0.770927932742981));
#47589=CARTESIAN_POINT('Ctrl Pts',(-14.7379324635813,-3.77192571564458,
-1.13666491400483));
#47590=CARTESIAN_POINT('Ctrl Pts',(-14.6716734547513,-3.39573441537366,
-2.38514144084738));
#47591=CARTESIAN_POINT('Ctrl Pts',(-14.6054144459213,-2.33830387177135,
-3.42841134974953));
#47592=CARTESIAN_POINT('Ctrl Pts',(-14.5391554370913,-1.08473860433526,
-3.78733713785681));
#47593=CARTESIAN_POINT('Ctrl Pts',(-14.4728964282613,0.168826663100827,
-4.14626292596409));
#47594=CARTESIAN_POINT('Ctrl Pts',(-14.4066374194313,1.61852665437069,-3.8208445932765));
#47595=CARTESIAN_POINT('Ctrl Pts',(-14.3403784106013,2.59847629869133,-2.9609978388901));
#47596=CARTESIAN_POINT('Ctrl Pts',(-14.2741194017713,3.57842594301196,-2.1011510845037));
#47597=CARTESIAN_POINT('Ctrl Pts',(-14.2078603929413,4.08862524038336,-0.706875908418483));
#47598=CARTESIAN_POINT('Ctrl Pts',(-14.1416013841113,3.89583993798937,0.582937987716999));
#47599=CARTESIAN_POINT('Ctrl Pts',(-14.079512033852,3.71518655399588,1.79158430133742));
#47600=CARTESIAN_POINT('Ctrl Pts',(-14.0174226835927,2.9172418482862,2.90850308409889));
#47601=CARTESIAN_POINT('Ctrl Pts',(-13.9553333333333,1.83875391880586,3.48426281672735));
#47602=CARTESIAN_POINT('',(-26.267,-1.87158653173891,-2.62360084935066));
#47603=CARTESIAN_POINT('Ctrl Pts',(-26.267,-1.87563364385541,-2.62744043199008));
#47604=CARTESIAN_POINT('Ctrl Pts',(-26.267,-1.93502283818884,-2.59436675243734));
#47605=CARTESIAN_POINT('Ctrl Pts',(-26.267,-1.99319562091243,-2.55933411580012));
#47606=CARTESIAN_POINT('Ctrl Pts',(-26.267,-2.05004339163671,-2.52236226376319));
#47607=CARTESIAN_POINT('Ctrl Pts',(-26.267,-2.13607085868267,-2.46641293202665));
#47608=CARTESIAN_POINT('Ctrl Pts',(-26.267,-2.21906528067624,-2.40602533039299));
#47609=CARTESIAN_POINT('Ctrl Pts',(-26.267,-2.29893371013539,-2.3415918437389));
#47610=CARTESIAN_POINT('Ctrl Pts',(-26.267,-2.34933821690132,-2.30092824066067));
#47611=CARTESIAN_POINT('Ctrl Pts',(-26.267,-2.39849739182093,-2.25865218486351));
#47612=CARTESIAN_POINT('Ctrl Pts',(-26.267,-2.44638375817581,-2.21485267411829));
#47613=CARTESIAN_POINT('Ctrl Pts',(-26.267,-2.4769857683737,-2.1868623884375));
#47614=CARTESIAN_POINT('Ctrl Pts',(-26.267,-2.50706790697913,-2.15824979279682));
#47615=CARTESIAN_POINT('Ctrl Pts',(-26.267,-2.53662217937948,-2.12903671190489));
#47616=CARTESIAN_POINT('Ctrl Pts',(-26.267,-2.54989830294754,-2.11591385553843));
#47617=CARTESIAN_POINT('Ctrl Pts',(-26.267,-2.5630668342312,-2.10267076594302));
#47618=CARTESIAN_POINT('Ctrl Pts',(-26.267,-2.57611858766727,-2.0893183706114));
#47619=CARTESIAN_POINT('Ctrl Pts',(-26.267,-2.65028331647228,-2.01344528708147));
#47620=CARTESIAN_POINT('Ctrl Pts',(-26.267,-2.72075551146666,-1.93397177742404));
#47621=CARTESIAN_POINT('Ctrl Pts',(-26.267,-2.78743443104751,-1.85130541984555));
#47622=CARTESIAN_POINT('Ctrl Pts',(-26.267,-2.8510104455509,-1.77248594314454));
#47623=CARTESIAN_POINT('Ctrl Pts',(-26.267,-2.91113820636111,-1.69076303840862));
#47624=CARTESIAN_POINT('Ctrl Pts',(-26.267,-2.96770924376778,-1.60645353911803));
#47625=CARTESIAN_POINT('Ctrl Pts',(-26.267,-2.9924590726332,-1.56956813317839));
#47626=CARTESIAN_POINT('Ctrl Pts',(-26.267,-3.01652782447795,-1.53218722341775));
#47627=CARTESIAN_POINT('Ctrl Pts',(-26.267,-3.03990490959769,-1.49433557773647));
#47628=CARTESIAN_POINT('Ctrl Pts',(-26.267,-3.05147433099463,-1.47560263317938));
#47629=CARTESIAN_POINT('Ctrl Pts',(-26.267,-3.06287432707377,-1.45675437603992));
#47630=CARTESIAN_POINT('Ctrl Pts',(-26.267,-3.07410352161292,-1.43779372484651));
#47631=CARTESIAN_POINT('Ctrl Pts',(-26.267,-3.08210732291092,-1.42427919501059));
#47632=CARTESIAN_POINT('Ctrl Pts',(-26.267,-3.09002304737044,-1.41070968749839));
#47633=CARTESIAN_POINT('Ctrl Pts',(-26.267,-3.09784603919882,-1.39709387173809));
#47634=CARTESIAN_POINT('Ctrl Pts',(-26.267,-3.15328862986162,-1.30059676215397));
#47635=CARTESIAN_POINT('Ctrl Pts',(-26.267,-3.2041395175185,-1.20167030949908));
#47636=CARTESIAN_POINT('Ctrl Pts',(-26.267,-3.25029005553095,-1.10074331911095));
#47637=CARTESIAN_POINT('Ctrl Pts',(-26.267,-3.29716691060663,-0.998227939975572));
#47638=CARTESIAN_POINT('Ctrl Pts',(-26.267,-3.33919489299649,-0.893647890501421));
#47639=CARTESIAN_POINT('Ctrl Pts',(-26.267,-3.37622637228166,-0.78741086593843));
#47640=CARTESIAN_POINT('Ctrl Pts',(-26.267,-3.41317015926056,-0.681425415708303));
#47641=CARTESIAN_POINT('Ctrl Pts',(-26.267,-3.44514158615419,-0.573790016793496));
#47642=CARTESIAN_POINT('Ctrl Pts',(-26.267,-3.47195261401537,-0.464879656108174));
#47643=CARTESIAN_POINT('Ctrl Pts',(-26.267,-3.48936130848388,-0.394162964325869));
#47644=CARTESIAN_POINT('Ctrl Pts',(-26.267,-3.50459349604628,-0.322908164365236));
#47645=CARTESIAN_POINT('Ctrl Pts',(-26.267,-3.51758674381885,-0.251213629832156));
#47646=CARTESIAN_POINT('Ctrl Pts',(-26.267,-3.52123597647577,-0.231077783789654));
#47647=CARTESIAN_POINT('Ctrl Pts',(-26.267,-3.52470854490799,-0.210907237194771));
#47648=CARTESIAN_POINT('Ctrl Pts',(-26.267,-3.52800293081593,-0.190704140748007));
#47649=CARTESIAN_POINT('Ctrl Pts',(-26.267,-3.5310853921128,-0.171800689660538));
#47650=CARTESIAN_POINT('Ctrl Pts',(-26.267,-3.53401203475742,-0.152866889646329));
#47651=CARTESIAN_POINT('Ctrl Pts',(-26.267,-3.53677862597875,-0.13392654036373));
#47652=CARTESIAN_POINT('Ctrl Pts',(-26.267,-3.5535210675383,-0.0193061770309027));
#47653=CARTESIAN_POINT('Ctrl Pts',(-26.267,-3.56443587029357,0.0957288600444009));
#47654=CARTESIAN_POINT('Ctrl Pts',(-26.267,-3.56937634543034,0.210754462446548));
#47655=CARTESIAN_POINT('Ctrl Pts',(-26.267,-3.57206682834186,0.273395080824828));
#47656=CARTESIAN_POINT('Ctrl Pts',(-26.267,-3.57298480067844,0.336033459704283));
#47657=CARTESIAN_POINT('Ctrl Pts',(-26.267,-3.57210088426465,0.398604262522089));
#47658=CARTESIAN_POINT('Ctrl Pts',(-26.267,-3.57053367028861,0.509544431908386));
#47659=CARTESIAN_POINT('Ctrl Pts',(-26.267,-3.56330522231868,0.620271859661915));
#47660=CARTESIAN_POINT('Ctrl Pts',(-26.267,-3.55068015331886,0.730501366588306));
#47661=CARTESIAN_POINT('Ctrl Pts',(-26.267,-3.53781478472759,0.842828929808865));
#47662=CARTESIAN_POINT('Ctrl Pts',(-26.267,-3.51934530799955,0.954640114197353));
#47663=CARTESIAN_POINT('Ctrl Pts',(-26.267,-3.49549764638492,1.06563656127855));
#47664=CARTESIAN_POINT('Ctrl Pts',(-26.267,-3.4879842997281,1.10060664757351));
#47665=CARTESIAN_POINT('Ctrl Pts',(-26.267,-3.47993672291489,1.13549584598195));
#47666=CARTESIAN_POINT('Ctrl Pts',(-26.267,-3.47136092544872,1.17029472302242));
#47667=CARTESIAN_POINT('Ctrl Pts',(-26.267,-3.46751408660795,1.18590442839879));
#47668=CARTESIAN_POINT('Ctrl Pts',(-26.267,-3.4635602913321,1.20149849192874));
#47669=CARTESIAN_POINT('Ctrl Pts',(-26.267,-3.45950226226653,1.21706761472067));
#47670=CARTESIAN_POINT('Ctrl Pts',(-26.267,-3.43079460214631,1.32720804946344));
#47671=CARTESIAN_POINT('Ctrl Pts',(-26.267,-3.39693213439927,1.43588706906917));
#47672=CARTESIAN_POINT('Ctrl Pts',(-26.267,-3.3582177646934,1.54281137140461));
#47673=CARTESIAN_POINT('Ctrl Pts',(-26.267,-3.31822881808711,1.65325589754548));
#47674=CARTESIAN_POINT('Ctrl Pts',(-26.267,-3.27306321397473,1.76182895533595));
#47675=CARTESIAN_POINT('Ctrl Pts',(-26.267,-3.22299936023802,1.86821150838332));
#47676=CARTESIAN_POINT('Ctrl Pts',(-26.267,-3.17243003712686,1.97566815218736));
#47677=CARTESIAN_POINT('Ctrl Pts',(-26.267,-3.1168627999695,2.0808906344938));
#47678=CARTESIAN_POINT('Ctrl Pts',(-26.267,-3.05653137285161,2.18354294711263));
#47679=CARTESIAN_POINT('Ctrl Pts',(-26.267,-3.01664457625045,2.251409266702));
#47680=CARTESIAN_POINT('Ctrl Pts',(-26.267,-2.97467431085533,2.31815202427033));
#47681=CARTESIAN_POINT('Ctrl Pts',(-26.267,-2.93067640862396,2.38366977677781));
#47682=CARTESIAN_POINT('Ctrl Pts',(-26.267,-2.90918410881585,2.41567419308474));
#47683=CARTESIAN_POINT('Ctrl Pts',(-26.267,-2.88720784447261,2.44738623633731));
#47684=CARTESIAN_POINT('Ctrl Pts',(-26.267,-2.86475337266313,2.47879364579308));
#47685=CARTESIAN_POINT('Ctrl Pts',(-26.267,-2.8507640646594,2.49836070255592));
#47686=CARTESIAN_POINT('Ctrl Pts',(-26.267,-2.83658549398819,2.5178142532328));
#47687=CARTESIAN_POINT('Ctrl Pts',(-26.267,-2.82223936577275,2.53712428807426));
#47688=CARTESIAN_POINT('Ctrl Pts',(-26.267,-2.74908754426023,2.63558738563692));
#47689=CARTESIAN_POINT('Ctrl Pts',(-26.267,-2.6715065446943,2.73043209404712));
#47690=CARTESIAN_POINT('Ctrl Pts',(-26.267,-2.58978746881353,2.82132277898767));
#47691=CARTESIAN_POINT('Ctrl Pts',(-26.267,-2.50797450479922,2.91231788944545));
#47692=CARTESIAN_POINT('Ctrl Pts',(-26.267,-2.42201356354227,2.99935071595012));
#47693=CARTESIAN_POINT('Ctrl Pts',(-26.267,-2.33214667543519,3.08206867663245));
#47694=CARTESIAN_POINT('Ctrl Pts',(-26.267,-2.24243448349077,3.16464424726023));
#47695=CARTESIAN_POINT('Ctrl Pts',(-26.267,-2.14882937383503,3.2429206277689));
#47696=CARTESIAN_POINT('Ctrl Pts',(-26.267,-2.05152823317363,3.31651888350284));
#47697=CARTESIAN_POINT('Ctrl Pts',(-26.267,-1.95422709251222,3.39011713923678));
#47698=CARTESIAN_POINT('Ctrl Pts',(-26.267,-1.85322952476273,3.45903813975137));
#47699=CARTESIAN_POINT('Ctrl Pts',(-26.267,-1.74869447533123,3.52286199445082));
#47700=CARTESIAN_POINT('Ctrl Pts',(-26.267,-1.87563364385542,-2.62744043199007));
#47701=CARTESIAN_POINT('Ctrl Pts',(-26.2049106497406,-1.05751970818542,
-3.20557823490714));
#47702=CARTESIAN_POINT('Ctrl Pts',(-26.0765622906514,1.23967409930297,-3.56474568943846));
#47703=CARTESIAN_POINT('Ctrl Pts',(-25.881954922732,3.68771187601412,-0.961936478150598));
#47704=CARTESIAN_POINT('Ctrl Pts',(-25.683177896242,2.80382800818523,2.58188775682714));
#47705=CARTESIAN_POINT('Ctrl Pts',(-25.4844008697521,-0.654391852565681,
3.75444098441731));
#47706=CARTESIAN_POINT('Ctrl Pts',(-25.3254170879137,-2.93965552881964,
1.93616476772919));
#47707=CARTESIAN_POINT('Ctrl Pts',(-25.2326923149053,-3.2203404239648,0.431815865334146));
#47708=CARTESIAN_POINT('Ctrl Pts',(-25.2062265507269,-3.2183080224723,0.00170933992184336));
#47709=CARTESIAN_POINT('Origin',(-26.267,-5.160062080289E-16,2.1385152528819E-16));
#47710=CARTESIAN_POINT('',(-26.267,-3.933,-4.81653586104654E-16));
#47711=CARTESIAN_POINT('Origin',(-26.267,0.,0.));
#47712=CARTESIAN_POINT('Origin',(-26.267,0.,0.));
#47713=CARTESIAN_POINT('',(-26.267,1.87158653173906,-2.62360084935056));
#47714=CARTESIAN_POINT('Ctrl Pts',(-26.267,1.75283089415088,3.52826931739087));
#47715=CARTESIAN_POINT('Ctrl Pts',(-26.267,1.82318529142576,3.48569183564302));
#47716=CARTESIAN_POINT('Ctrl Pts',(-26.267,1.89201450465608,3.44079991594677));
#47717=CARTESIAN_POINT('Ctrl Pts',(-26.267,1.95918967345583,3.39358641303125));
#47718=CARTESIAN_POINT('Ctrl Pts',(-26.267,2.05858783056501,3.32372525355339));
#47719=CARTESIAN_POINT('Ctrl Pts',(-26.267,2.15436645871861,3.2487822944279));
#47720=CARTESIAN_POINT('Ctrl Pts',(-26.267,2.2463413446018,3.16916750603609));
#47721=CARTESIAN_POINT('Ctrl Pts',(-26.267,2.29959316990593,3.12307195764421));
#47722=CARTESIAN_POINT('Ctrl Pts',(-26.267,2.35156916978231,3.07540964020356));
#47723=CARTESIAN_POINT('Ctrl Pts',(-26.267,2.40222706109326,3.02625573708493));
#47724=CARTESIAN_POINT('Ctrl Pts',(-26.267,2.44077608680837,2.98885119800362));
#47725=CARTESIAN_POINT('Ctrl Pts',(-26.267,2.47856173650469,2.95058285557362));
#47726=CARTESIAN_POINT('Ctrl Pts',(-26.267,2.51556336696653,2.91148297010551));
#47727=CARTESIAN_POINT('Ctrl Pts',(-26.267,2.5309182697087,2.89525733542134));
#47728=CARTESIAN_POINT('Ctrl Pts',(-26.267,2.54613902333768,2.87888740355848));
#47729=CARTESIAN_POINT('Ctrl Pts',(-26.267,2.56121192590708,2.86238909910956));
#47730=CARTESIAN_POINT('Ctrl Pts',(-26.267,2.6442839721244,2.7714611638046));
#47731=CARTESIAN_POINT('Ctrl Pts',(-26.267,2.72295590508143,2.67654596393466));
#47732=CARTESIAN_POINT('Ctrl Pts',(-26.267,2.79703275170125,2.57806849708916));
#47733=CARTESIAN_POINT('Ctrl Pts',(-26.267,2.8618499924936,2.49190071359935));
#47734=CARTESIAN_POINT('Ctrl Pts',(-26.267,2.92314859484406,2.40300461939636));
#47735=CARTESIAN_POINT('Ctrl Pts',(-26.267,2.98076610429264,2.31165085214935));
#47736=CARTESIAN_POINT('Ctrl Pts',(-26.267,3.0059737646764,2.27168357897878));
#47737=CARTESIAN_POINT('Ctrl Pts',(-26.267,3.03047643909033,2.23124577127131));
#47738=CARTESIAN_POINT('Ctrl Pts',(-26.267,3.05425858581036,2.19035969246717));
#47739=CARTESIAN_POINT('Ctrl Pts',(-26.267,3.06887962712138,2.16522331372566));
#47740=CARTESIAN_POINT('Ctrl Pts',(-26.267,3.08322830871726,2.13991749966683));
#47741=CARTESIAN_POINT('Ctrl Pts',(-26.267,3.09730078700632,2.11444740602352));
#47742=CARTESIAN_POINT('Ctrl Pts',(-26.267,3.10816559861413,2.09478294015024));
#47743=CARTESIAN_POINT('Ctrl Pts',(-26.267,3.11886718250786,2.07501769605134));
#47744=CARTESIAN_POINT('Ctrl Pts',(-26.267,3.12939220522335,2.05517627074448));
#47745=CARTESIAN_POINT('Ctrl Pts',(-26.267,3.18510294740167,1.95015221905346));
#47746=CARTESIAN_POINT('Ctrl Pts',(-26.267,3.23593990370189,1.84287352231398));
#47747=CARTESIAN_POINT('Ctrl Pts',(-26.267,3.28172717922646,1.73371644648934));
#47748=CARTESIAN_POINT('Ctrl Pts',(-26.267,3.32717541816672,1.62536763544387));
#47749=CARTESIAN_POINT('Ctrl Pts',(-26.267,3.36764871242685,1.51516729601585));
#47750=CARTESIAN_POINT('Ctrl Pts',(-26.267,3.40292543327883,1.40347149798005));
#47751=CARTESIAN_POINT('Ctrl Pts',(-26.267,3.43716006905266,1.29507522783728));
#47752=CARTESIAN_POINT('Ctrl Pts',(-26.267,3.46650062833312,1.18526981387765));
#47753=CARTESIAN_POINT('Ctrl Pts',(-26.267,3.49069615978602,1.07438111431325));
#47754=CARTESIAN_POINT('Ctrl Pts',(-26.267,3.50690239180499,1.000107565211));
#47755=CARTESIAN_POINT('Ctrl Pts',(-26.267,3.52079939350193,0.92534803949904));
#47756=CARTESIAN_POINT('Ctrl Pts',(-26.267,3.53229894330973,0.850202948550371));
#47757=CARTESIAN_POINT('Ctrl Pts',(-26.267,3.53786991304331,0.813798825406446));
#47758=CARTESIAN_POINT('Ctrl Pts',(-26.267,3.54287805976906,0.777304254618612));
#47759=CARTESIAN_POINT('Ctrl Pts',(-26.267,3.5473124432343,0.740730938484744));
#47760=CARTESIAN_POINT('Ctrl Pts',(-26.267,3.54918812804797,0.725260915606478));
#47761=CARTESIAN_POINT('Ctrl Pts',(-26.267,3.55096058609398,0.709781155383269));
#47762=CARTESIAN_POINT('Ctrl Pts',(-26.267,3.55262839016636,0.694300444279272));
#47763=CARTESIAN_POINT('Ctrl Pts',(-26.267,3.56460695007169,0.58311434729857));
#47764=CARTESIAN_POINT('Ctrl Pts',(-26.267,3.57120627580917,0.471755619772827));
#47765=CARTESIAN_POINT('Ctrl Pts',(-26.267,3.57222914249298,0.360540007381168));
#47766=CARTESIAN_POINT('Ctrl Pts',(-26.267,3.57281215830709,0.297149086719328));
#47767=CARTESIAN_POINT('Ctrl Pts',(-26.267,3.57158257655703,0.233804656091378));
#47768=CARTESIAN_POINT('Ctrl Pts',(-26.267,3.56849629185414,0.1705660434067));
#47769=CARTESIAN_POINT('Ctrl Pts',(-26.267,3.56297727258772,0.0574801957330568));
#47770=CARTESIAN_POINT('Ctrl Pts',(-26.267,3.55152347402166,-0.0552685595518794));
#47771=CARTESIAN_POINT('Ctrl Pts',(-26.267,3.53434939023894,-0.167322691080499));
#47772=CARTESIAN_POINT('Ctrl Pts',(-26.267,3.51709931727261,-0.279872622098812));
#47773=CARTESIAN_POINT('Ctrl Pts',(-26.267,3.49407768877409,-0.391722571953211));
#47774=CARTESIAN_POINT('Ctrl Pts',(-26.267,3.46545702485941,-0.502483636464418));
#47775=CARTESIAN_POINT('Ctrl Pts',(-26.267,3.45682536428132,-0.53588789001278));
#47776=CARTESIAN_POINT('Ctrl Pts',(-26.267,3.44768416297063,-0.569192875179334));
#47777=CARTESIAN_POINT('Ctrl Pts',(-26.267,3.4380374717033,-0.602387281756488));
#47778=CARTESIAN_POINT('Ctrl Pts',(-26.267,3.43312300749121,-0.619298025414007));
#47779=CARTESIAN_POINT('Ctrl Pts',(-26.267,3.42807681352333,-0.636181555219225));
#47780=CARTESIAN_POINT('Ctrl Pts',(-26.267,3.42290515904448,-0.653018316007086));
#47781=CARTESIAN_POINT('Ctrl Pts',(-26.267,3.39020902314041,-0.759463365875591));
#47782=CARTESIAN_POINT('Ctrl Pts',(-26.267,3.35245638616911,-0.864203255159293));
#47783=CARTESIAN_POINT('Ctrl Pts',(-26.267,3.30988295914673,-0.966911473140547));
#47784=CARTESIAN_POINT('Ctrl Pts',(-26.267,3.26726860350859,-1.06971843123938));
#47785=CARTESIAN_POINT('Ctrl Pts',(-26.267,3.21982359879886,-1.17049056087227));
#47786=CARTESIAN_POINT('Ctrl Pts',(-26.267,3.16773965001191,-1.26887337505142));
#47787=CARTESIAN_POINT('Ctrl Pts',(-26.267,3.11629546913592,-1.36604771389475));
#47788=CARTESIAN_POINT('Ctrl Pts',(-26.267,3.06032498942971,-1.46089169808994));
#47789=CARTESIAN_POINT('Ctrl Pts',(-26.267,2.99997844698005,-1.55302727802699));
#47790=CARTESIAN_POINT('Ctrl Pts',(-26.267,2.96406011993936,-1.60786647440717));
#47791=CARTESIAN_POINT('Ctrl Pts',(-26.267,2.92659089603249,-1.66174543872833));
#47792=CARTESIAN_POINT('Ctrl Pts',(-26.267,2.88759787269679,-1.71457684344143));
#47793=CARTESIAN_POINT('Ctrl Pts',(-26.267,2.86970645321483,-1.73881781638177));
#47794=CARTESIAN_POINT('Ctrl Pts',(-26.267,2.85149418486337,-1.76283816019293));
#47795=CARTESIAN_POINT('Ctrl Pts',(-26.267,2.83296348753158,-1.7866289832168));
#47796=CARTESIAN_POINT('Ctrl Pts',(-26.267,2.82442940049083,-1.79758555710183));
#47797=CARTESIAN_POINT('Ctrl Pts',(-26.267,2.81582890705879,-1.80849193308911));
#47798=CARTESIAN_POINT('Ctrl Pts',(-26.267,2.80716807563418,-1.81934019128409));
#47799=CARTESIAN_POINT('Ctrl Pts',(-26.267,2.74005470260851,-1.90340408344692));
#47800=CARTESIAN_POINT('Ctrl Pts',(-26.267,2.66922556996508,-1.98410424668023));
#47801=CARTESIAN_POINT('Ctrl Pts',(-26.267,2.5948569520778,-2.0611209847473));
#47802=CARTESIAN_POINT('Ctrl Pts',(-26.267,2.52152149137489,-2.13706777693517));
#47803=CARTESIAN_POINT('Ctrl Pts',(-26.267,2.44474361560077,-2.20943329052733));
#47804=CARTESIAN_POINT('Ctrl Pts',(-26.267,2.36466364179145,-2.27787037127922));
#47805=CARTESIAN_POINT('Ctrl Pts',(-26.267,2.28705702719922,-2.34419369653874));
#47806=CARTESIAN_POINT('Ctrl Pts',(-26.267,2.20634859789478,-2.40682779771474));
#47807=CARTESIAN_POINT('Ctrl Pts',(-26.267,2.12264725251138,-2.465412696323));
#47808=CARTESIAN_POINT('Ctrl Pts',(-26.267,2.04172880706709,-2.5220497658967));
#47809=CARTESIAN_POINT('Ctrl Pts',(-26.267,1.95801272086933,-2.57490258924474));
#47810=CARTESIAN_POINT('Ctrl Pts',(-26.267,1.87158653173909,-2.62360084935053));
#47811=CARTESIAN_POINT('Origin',(-26.267,0.,0.));
#47812=CARTESIAN_POINT('Origin',(-28.5777734492731,0.,0.));
#47813=CARTESIAN_POINT('Ctrl Pts',(-26.267,1.87158653173906,-2.62360084935056));
#47814=CARTESIAN_POINT('Ctrl Pts',(-26.20074099117,2.74538756344498,-2.00026127284245));
#47815=CARTESIAN_POINT('Ctrl Pts',(-26.06822297351,3.80572572838508,0.177707626592857));
#47816=CARTESIAN_POINT('Ctrl Pts',(-25.86944594702,1.90626263650645,3.30303297573159));
#47817=CARTESIAN_POINT('Ctrl Pts',(-25.6706689205301,-1.74511074991996,
3.38706745932803));
#47818=CARTESIAN_POINT('Ctrl Pts',(-25.5317780879477,-3.17634659584044,
1.27640733554319));
#47819=CARTESIAN_POINT('Ctrl Pts',(-25.4591462641954,-3.22750339797143,
0.104841723461124));
#47820=CARTESIAN_POINT('Ctrl Pts',(-25.4527734492731,-3.22681880944319,
0.00198271668292602));
#47821=CARTESIAN_POINT('Ctrl Pts',(-26.6770630286919,2.28405859260867,-3.20180657528379));
#47822=CARTESIAN_POINT('Ctrl Pts',(-26.6108040198619,3.35043341463937,-2.44109148587059));
#47823=CARTESIAN_POINT('Ctrl Pts',(-26.478286002202,4.64445560150136,0.21687195574883));
#47824=CARTESIAN_POINT('Ctrl Pts',(-26.279508975712,2.32637683636025,4.03097624499334));
#47825=CARTESIAN_POINT('Ctrl Pts',(-26.080731949222,-2.12970927916688,4.13353077884949));
#47826=CARTESIAN_POINT('Ctrl Pts',(-25.881954922732,-4.62948555759545,0.447081669639946));
#47827=CARTESIAN_POINT('Ctrl Pts',(-25.683177896242,-2.88011351910651,-3.65260393366682));
#47828=CARTESIAN_POINT('Ctrl Pts',(-25.4844008697521,1.51350000628727,-4.39779790151484));
#47829=CARTESIAN_POINT('Ctrl Pts',(-25.2856238432621,4.51756764805872,-1.10662356178153));
#47830=CARTESIAN_POINT('Ctrl Pts',(-25.0868468167721,3.37466122935008,3.20080160309462));
#47831=CARTESIAN_POINT('Ctrl Pts',(-24.8880697902821,-0.866183191727884,
4.56973678783709));
#47832=CARTESIAN_POINT('Ctrl Pts',(-24.6892927637922,-4.31185972195668,
1.74382019235027));
#47833=CARTESIAN_POINT('Ctrl Pts',(-24.4905157373022,-3.79932173433631,
-2.6829517902416));
#47834=CARTESIAN_POINT('Ctrl Pts',(-24.2917387108122,0.200946718919985,
-4.64678435357141));
#47835=CARTESIAN_POINT('Ctrl Pts',(-24.0929616843222,4.01674563032601,-2.34494803611166));
#47836=CARTESIAN_POINT('Ctrl Pts',(-23.8941846578323,4.14523001189322,2.10952497302619));
#47837=CARTESIAN_POINT('Ctrl Pts',(-23.6954076313422,0.468450447046365,
4.62747987472434));
#47838=CARTESIAN_POINT('Ctrl Pts',(-23.4966306048523,-3.63835961735965,
2.89747500715715));
#47839=CARTESIAN_POINT('Ctrl Pts',(-23.2978535783623,-4.40520675631299,
-1.49237231725802));
#47840=CARTESIAN_POINT('Ctrl Pts',(-23.0990765518723,-1.12813568952015,
-4.51224225015275));
#47841=CARTESIAN_POINT('Ctrl Pts',(-22.9002995253823,3.18454807402148,-3.38993727651186));
#47842=CARTESIAN_POINT('Ctrl Pts',(-22.7015224988924,4.57386135182184,0.844282761045225));
#47843=CARTESIAN_POINT('Ctrl Pts',(-22.5027454724023,1.76443397075476,4.30346298195321));
#47844=CARTESIAN_POINT('Ctrl Pts',(-22.3039684459125,-2.6647190678634,3.81212451182053));
#47845=CARTESIAN_POINT('Ctrl Pts',(-22.1051914194224,-4.64769733843289,
-0.178690872093036));
#47846=CARTESIAN_POINT('Ctrl Pts',(-21.9064143929325,-2.36415456292714,
-4.00547052921664));
#47847=CARTESIAN_POINT('Ctrl Pts',(-21.7076373664425,2.08964897909848,-4.15528436091349));
#47848=CARTESIAN_POINT('Ctrl Pts',(-21.5088603399525,4.62518403425973,-0.490605361020961));
#47849=CARTESIAN_POINT('Ctrl Pts',(-21.3100833134625,2.9148649431019,3.62444248573818));
#47850=CARTESIAN_POINT('Ctrl Pts',(-21.1113062869726,-1.47125932928464,
4.41230290861746));
#47851=CARTESIAN_POINT('Ctrl Pts',(-20.9125292604826,-4.50678814936917,
1.14973107607421));
#47852=CARTESIAN_POINT('Ctrl Pts',(-20.7137522339926,-3.40514858703943,
-3.16827777674092));
#47853=CARTESIAN_POINT('Ctrl Pts',(-20.5149752075026,0.822369673066674,
-4.57785201721419));
#47854=CARTESIAN_POINT('Ctrl Pts',(-20.3161981810127,4.29496409445361,-1.78502224017813));
#47855=CARTESIAN_POINT('Ctrl Pts',(-20.1174211545226,3.82484164829531,2.64643294571342));
#47856=CARTESIAN_POINT('Ctrl Pts',(-19.9186441280327,-0.1564318461399,4.64849976314082));
#47857=CARTESIAN_POINT('Ctrl Pts',(-19.7198671015427,-3.99410309733264,
2.38330892216325));
#47858=CARTESIAN_POINT('Ctrl Pts',(-19.5210900750527,-4.16524366145492,
-2.06972612007259));
#47859=CARTESIAN_POINT('Ctrl Pts',(-19.3223130485628,-0.512748897982449,
-4.62278158001935));
#47860=CARTESIAN_POINT('Ctrl Pts',(-19.1235360220728,3.61044217001027,-2.93218831387842));
#47861=CARTESIAN_POINT('Ctrl Pts',(-18.9247589955828,4.41929790786022,1.45011274647242));
#47862=CARTESIAN_POINT('Ctrl Pts',(-18.7259819690928,1.17130007793737,4.50123061898145));
#47863=CARTESIAN_POINT('Ctrl Pts',(-18.5272049426028,-3.1519348112702,3.42028184846639));
#47864=CARTESIAN_POINT('Ctrl Pts',(-18.3284279161129,-4.58173770662756,
-0.800437750187337));
#47865=CARTESIAN_POINT('Ctrl Pts',(-18.1296508896229,-1.80556956591054,
-4.28636669183268));
#47866=CARTESIAN_POINT('Ctrl Pts',(-17.9308738631329,2.62808612112309,-3.83747109256185));
#47867=CARTESIAN_POINT('Ctrl Pts',(-17.7320968366429,4.64919560587807,0.134169268920524));
#47868=CARTESIAN_POINT('Ctrl Pts',(-17.5333198101529,2.40240858414375,3.98264400277819));
#47869=CARTESIAN_POINT('Ctrl Pts',(-17.334542783663,-2.04975571703512,4.1751075674365));
#47870=CARTESIAN_POINT('Ctrl Pts',(-17.135765757173,-4.62027326531467,0.534880431640867));
#47871=CARTESIAN_POINT('Ctrl Pts',(-16.936988730683,-2.94944414375022,-3.59635858267975));
#47872=CARTESIAN_POINT('Ctrl Pts',(-16.738211704193,1.42893233174933,-4.42619247825972));
#47873=CARTESIAN_POINT('Ctrl Pts',(-16.539434677703,4.49557098069678,-1.19284043707613));
#47874=CARTESIAN_POINT('Ctrl Pts',(-16.3406576512131,3.43533450362267,3.1355161075428));
#47875=CARTESIAN_POINT('Ctrl Pts',(-16.1418806247231,-0.778483263328775,
4.58552502538999));
#47876=CARTESIAN_POINT('Ctrl Pts',(-15.9431035982331,-4.27767915166076,
1.82606248538427));
#47877=CARTESIAN_POINT('Ctrl Pts',(-15.7443265717431,-3.84999670245527,
-2.60965381283173));
#47878=CARTESIAN_POINT('Ctrl Pts',(-15.5455495452531,0.111872910139692,
-4.64983373543921));
#47879=CARTESIAN_POINT('Ctrl Pts',(-15.3467725187632,3.97115313116304,-2.42135829053259));
#47880=CARTESIAN_POINT('Ctrl Pts',(-15.1479954922732,4.18476020427858,2.02955430680881));
#47881=CARTESIAN_POINT('Ctrl Pts',(-14.9492184657832,0.557223801909945,
4.61801591744371));
#47882=CARTESIAN_POINT('Ctrl Pts',(-14.7504414392932,-3.58262751545605,
2.96593975542493));
#47883=CARTESIAN_POINT('Ctrl Pts',(-14.5516644128033,-4.43213866584023,
-1.40637305158682));
#47884=CARTESIAN_POINT('Ctrl Pts',(-14.3528873863133,-1.21602745322486,
-4.49244653896489));
#47885=CARTESIAN_POINT('Ctrl Pts',(-14.1541103598233,3.1225857469175,-3.44491792829022));
#47886=CARTESIAN_POINT('Ctrl Pts',(-14.0215923421633,4.09368485114861,-0.652745009784278));
#47887=CARTESIAN_POINT('Ctrl Pts',(-13.9553333333333,3.88062570733445,0.639713310456302));
#47888=CARTESIAN_POINT('Ctrl Pts',(-26.5403753524613,2.14656790565213,-3.00907133330604));
#47889=CARTESIAN_POINT('Ctrl Pts',(-26.4741163436313,3.14875146424124,-2.29414808152788));
#47890=CARTESIAN_POINT('Ctrl Pts',(-26.3415983259713,4.36487897712927,0.203817179363504));
#47891=CARTESIAN_POINT('Ctrl Pts',(-26.1428212994813,2.18633876974231,3.78832848857276));
#47892=CARTESIAN_POINT('Ctrl Pts',(-25.9440442729914,-2.00150976941791,
3.88470967234234));
#47893=CARTESIAN_POINT('Ctrl Pts',(-25.7452672465014,-4.35081006668247,
0.420169240123723));
#47894=CARTESIAN_POINT('Ctrl Pts',(-25.5464902200114,-2.70674284134183,
-3.43273259339334));
#47895=CARTESIAN_POINT('Ctrl Pts',(-25.3477131935214,1.42239369393322,-4.1330690296146));
#47896=CARTESIAN_POINT('Ctrl Pts',(-25.1489361670314,4.24562914292832,-1.04000949408466));
#47897=CARTESIAN_POINT('Ctrl Pts',(-24.9501591405415,3.17152086676461,3.008126856201));
#47898=CARTESIAN_POINT('Ctrl Pts',(-24.7513821140515,-0.814042619482387,
4.29465792068213));
#47899=CARTESIAN_POINT('Ctrl Pts',(-24.5526050875615,-4.05230396574686,
1.63884957690685));
#47900=CARTESIAN_POINT('Ctrl Pts',(-24.3538280610715,-3.57061860171385,
-2.52144941639475));
#47901=CARTESIAN_POINT('Ctrl Pts',(-24.1550510345816,0.188850574576165,
-4.36706754815366));
#47902=CARTESIAN_POINT('Ctrl Pts',(-23.9562740080916,3.77495449684529,-2.20379206165209));
#47903=CARTESIAN_POINT('Ctrl Pts',(-23.7574969816016,3.89570466093576,1.98254047331505));
#47904=CARTESIAN_POINT('Ctrl Pts',(-23.5587199551116,0.440251707321398,
4.34892511745484));
#47905=CARTESIAN_POINT('Ctrl Pts',(-23.3599429286216,-3.41934572480692,
2.72305924108939));
#47906=CARTESIAN_POINT('Ctrl Pts',(-23.1611659021317,-4.14003190262443,
-1.40253780260996));
#47907=CARTESIAN_POINT('Ctrl Pts',(-22.9623888756417,-1.06022668252956,
-4.2406243114994));
#47908=CARTESIAN_POINT('Ctrl Pts',(-22.7636118491517,2.99285172097684,-3.18587736036281));
#47909=CARTESIAN_POINT('Ctrl Pts',(-22.5648348226617,4.29853420332353,0.793460502291752));
#47910=CARTESIAN_POINT('Ctrl Pts',(-22.3660577961718,1.65822249285589,4.0444126740515));
#47911=CARTESIAN_POINT('Ctrl Pts',(-22.1672807696817,-2.50431422694893,
3.58265070603016));
#47912=CARTESIAN_POINT('Ctrl Pts',(-21.9685037431918,-4.3679255751799,-0.167934435793016));
#47913=CARTESIAN_POINT('Ctrl Pts',(-21.7697267167018,-2.2218424366182,-3.76435810923392));
#47914=CARTESIAN_POINT('Ctrl Pts',(-21.5709496902118,1.96386093033125,-3.90515378058136));
#47915=CARTESIAN_POINT('Ctrl Pts',(-21.3721726637218,4.34676747689614,-0.461072988983897));
#47916=CARTESIAN_POINT('Ctrl Pts',(-21.1733956372319,2.73940237628791,3.40626634576907));
#47917=CARTESIAN_POINT('Ctrl Pts',(-20.9746186107419,-1.38269572740107,
4.14670089651087));
#47918=CARTESIAN_POINT('Ctrl Pts',(-20.7758415842519,-4.23549852456288,
1.08052211796066));
#47919=CARTESIAN_POINT('Ctrl Pts',(-20.577064557762,-3.20017301419894,-2.97756082692059));
#47920=CARTESIAN_POINT('Ctrl Pts',(-20.3782875312719,0.772866489721012,
-4.30228464750265));
#47921=CARTESIAN_POINT('Ctrl Pts',(-20.179510504782,4.03642538370816,-1.67757143535682));
#47922=CARTESIAN_POINT('Ctrl Pts',(-19.980733478292,3.59460232456433,2.4871288521722));
#47923=CARTESIAN_POINT('Ctrl Pts',(-19.781956451802,-0.147015309253664,
4.36867969730722));
#47924=CARTESIAN_POINT('Ctrl Pts',(-19.583179425312,-3.75367494877086,2.23984378427304));
#47925=CARTESIAN_POINT('Ctrl Pts',(-19.3844023988221,-3.91451357326538,
-1.94513734333037));
#47926=CARTESIAN_POINT('Ctrl Pts',(-19.1856253723321,-0.481883578481456,
-4.344509640261));
#47927=CARTESIAN_POINT('Ctrl Pts',(-18.9868483458421,3.3931087899569,-2.75568295326037));
#47928=CARTESIAN_POINT('Ctrl Pts',(-18.7880713193521,4.153274826323,1.36282207962083));
#47929=CARTESIAN_POINT('Ctrl Pts',(-18.5892942928622,1.10079275694786,4.23027553404785));
#47930=CARTESIAN_POINT('Ctrl Pts',(-18.3905172663722,-2.9622016389925,3.21439531716091));
#47931=CARTESIAN_POINT('Ctrl Pts',(-18.1917402398822,-4.30593643481365,
-0.752254776031014));
#47932=CARTESIAN_POINT('Ctrl Pts',(-17.9929632133922,-1.69688189880417,
-4.02834550843798));
#47933=CARTESIAN_POINT('Ctrl Pts',(-17.7941861869023,2.46988642898584,-3.60647152959107));
#47934=CARTESIAN_POINT('Ctrl Pts',(-17.5954091604123,4.36933365324861,0.126092845219305));
#47935=CARTESIAN_POINT('Ctrl Pts',(-17.3966321339223,2.25779372721619,3.74290564334323));
#47936=CARTESIAN_POINT('Ctrl Pts',(-17.1978551074323,-1.92636907426674,
3.92378371373942));
#47937=CARTESIAN_POINT('Ctrl Pts',(-16.9990780809424,-4.34215231551471,
0.502682887224133));
#47938=CARTESIAN_POINT('Ctrl Pts',(-16.8003010544524,-2.77190005500552,
-3.37987297514113));
#47939=CARTESIAN_POINT('Ctrl Pts',(-16.6015240279624,1.34291663646797,-4.15975437268433));
#47940=CARTESIAN_POINT('Ctrl Pts',(-16.4027470014724,4.2249565821003,-1.12103647738179));
#47941=CARTESIAN_POINT('Ctrl Pts',(-16.2039699749824,3.22854186600948,2.94677127193112));
#47942=CARTESIAN_POINT('Ctrl Pts',(-16.0051929484924,-0.731621856618111,
4.30949577297171));
#47943=CARTESIAN_POINT('Ctrl Pts',(-15.8064159220025,-4.02018092151693,
1.71614123101997));
#47944=CARTESIAN_POINT('Ctrl Pts',(-15.6076388955125,-3.61824315063571,
-2.45256366785642));
#47945=CARTESIAN_POINT('Ctrl Pts',(-15.4088618690225,0.105138633130912,
-4.36993337010353));
#47946=CARTESIAN_POINT('Ctrl Pts',(-15.2100848425326,3.73210647369982,-2.27560274126138));
#47947=CARTESIAN_POINT('Ctrl Pts',(-15.0113078160425,3.93285530258446,1.90738370367203));
#47948=CARTESIAN_POINT('Ctrl Pts',(-14.8125307895526,0.523681280907598,
4.340030850458));
#47949=CARTESIAN_POINT('Ctrl Pts',(-14.6137537630626,-3.36696846020962,
2.78740270048038));
#47950=CARTESIAN_POINT('Ctrl Pts',(-14.4149767365726,-4.16534262486954,
-1.32171532975536));
#47951=CARTESIAN_POINT('Ctrl Pts',(-14.2161997100827,-1.14282773302373,
-4.22202021857335));
#47952=CARTESIAN_POINT('Ctrl Pts',(-14.0174226835927,2.93461926444034,-3.23754840896076));
#47953=CARTESIAN_POINT('Ctrl Pts',(-13.8849046659327,3.84726230131148,-0.613452515233941));
#47954=CARTESIAN_POINT('Ctrl Pts',(-13.8186456571027,3.64702841869692,0.601205269202682));
#47955=CARTESIAN_POINT('Ctrl Pts',(-26.4036876762306,2.00907721869559,-2.8163360913283));
#47956=CARTESIAN_POINT('Ctrl Pts',(-26.3374286674006,2.94706951384311,-2.14720467718516));
#47957=CARTESIAN_POINT('Ctrl Pts',(-26.2049106497406,4.08530235275718,0.190762402978181));
#47958=CARTESIAN_POINT('Ctrl Pts',(-26.0061336232507,2.04630070312438,3.54568073215218));
#47959=CARTESIAN_POINT('Ctrl Pts',(-25.8073565967607,-1.87331025966893,
3.63588856583518));
#47960=CARTESIAN_POINT('Ctrl Pts',(-25.6085795702707,-4.0721345757695,0.3932568106075));
#47961=CARTESIAN_POINT('Ctrl Pts',(-25.4098025437808,-2.53337216357714,
-3.21286125311987));
#47962=CARTESIAN_POINT('Ctrl Pts',(-25.2110255172908,1.33128738157918,-3.86834015771436));
#47963=CARTESIAN_POINT('Ctrl Pts',(-25.0122484908008,3.97369063779791,-0.973395426387776));
#47964=CARTESIAN_POINT('Ctrl Pts',(-24.8134714643108,2.96838050417913,2.81545210930738));
#47965=CARTESIAN_POINT('Ctrl Pts',(-24.6146944378208,-0.761902047236896,
4.01957905352718));
#47966=CARTESIAN_POINT('Ctrl Pts',(-24.4159174113309,-3.79274820953704,
1.53387896146343));
#47967=CARTESIAN_POINT('Ctrl Pts',(-24.2171403848409,-3.34191546909139,
-2.3599470425479));
#47968=CARTESIAN_POINT('Ctrl Pts',(-24.0183633583509,0.176754430232343,
-4.0873507427359));
#47969=CARTESIAN_POINT('Ctrl Pts',(-23.8195863318609,3.53316336336457,-2.06263608719252));
#47970=CARTESIAN_POINT('Ctrl Pts',(-23.6208093053709,3.64617930997828,1.85555597360391));
#47971=CARTESIAN_POINT('Ctrl Pts',(-23.422032278881,0.412052967596436,4.07037036018533));
#47972=CARTESIAN_POINT('Ctrl Pts',(-23.223255252391,-3.2003318322542,2.54864347502163));
#47973=CARTESIAN_POINT('Ctrl Pts',(-23.024478225901,-3.87485704893586,-1.31270328796191));
#47974=CARTESIAN_POINT('Ctrl Pts',(-22.825701199411,-0.992317675538989,
-3.96900637284604));
#47975=CARTESIAN_POINT('Ctrl Pts',(-22.6269241729211,2.80115536793221,-2.98181744421376));
#47976=CARTESIAN_POINT('Ctrl Pts',(-22.4281471464311,4.02320705482523,0.742638243538281));
#47977=CARTESIAN_POINT('Ctrl Pts',(-22.2293701199411,1.55201101495703,3.7853623661498));
#47978=CARTESIAN_POINT('Ctrl Pts',(-22.0305930934511,-2.34390938603446,
3.35317690023979));
#47979=CARTESIAN_POINT('Ctrl Pts',(-21.8318160669611,-4.08815381192692,
-0.157177999492998));
#47980=CARTESIAN_POINT('Ctrl Pts',(-21.6330390404712,-2.07953031030926,
-3.52324568925121));
#47981=CARTESIAN_POINT('Ctrl Pts',(-21.4342620139812,1.83807288156401,-3.65502320024922));
#47982=CARTESIAN_POINT('Ctrl Pts',(-21.2354849874912,4.06835091953256,-0.431540616946836));
#47983=CARTESIAN_POINT('Ctrl Pts',(-21.0367079610012,2.56393980947392,3.18809020579997));
#47984=CARTESIAN_POINT('Ctrl Pts',(-20.8379309345113,-1.29413212551749,
3.88109888440429));
#47985=CARTESIAN_POINT('Ctrl Pts',(-20.6391539080213,-3.96420889975659,
1.0113131598471));
#47986=CARTESIAN_POINT('Ctrl Pts',(-20.4403768815313,-2.99519744135846,
-2.78684387710026));
#47987=CARTESIAN_POINT('Ctrl Pts',(-20.2415998550413,0.723363306375352,
-4.02671727779112));
#47988=CARTESIAN_POINT('Ctrl Pts',(-20.0428228285513,3.7778866729627,-1.57012063053551));
#47989=CARTESIAN_POINT('Ctrl Pts',(-19.8440458020614,3.36436300083335,2.32782475863098));
#47990=CARTESIAN_POINT('Ctrl Pts',(-19.6452687755714,-0.137598772367427,
4.0888596314736));
#47991=CARTESIAN_POINT('Ctrl Pts',(-19.4464917490814,-3.51324680020908,
2.09637864638283));
#47992=CARTESIAN_POINT('Ctrl Pts',(-19.2477147225914,-3.66378348507584,
-1.82054856658815));
#47993=CARTESIAN_POINT('Ctrl Pts',(-19.0489376961015,-0.451018258980463,
-4.06623770050266));
#47994=CARTESIAN_POINT('Ctrl Pts',(-18.8501606696115,3.17577540990353,-2.57917759264233));
#47995=CARTESIAN_POINT('Ctrl Pts',(-18.6513836431215,3.88725174478577,1.27553141276924));
#47996=CARTESIAN_POINT('Ctrl Pts',(-18.4526066166315,1.03028543595836,3.95932044911425));
#47997=CARTESIAN_POINT('Ctrl Pts',(-18.2538295901415,-2.7724684667148,3.00850878585543));
#47998=CARTESIAN_POINT('Ctrl Pts',(-18.0550525636516,-4.03013516299975,
-0.704071801874699));
#47999=CARTESIAN_POINT('Ctrl Pts',(-17.8562755371616,-1.5881942316978,-3.77032432504327));
#48000=CARTESIAN_POINT('Ctrl Pts',(-17.6574985106716,2.31168673684857,-3.3754719666203));
#48001=CARTESIAN_POINT('Ctrl Pts',(-17.4587214841816,4.08947170061916,0.118016421518091));
#48002=CARTESIAN_POINT('Ctrl Pts',(-17.2599444576917,2.11317887028864,3.50316728390827));
#48003=CARTESIAN_POINT('Ctrl Pts',(-17.0611674312017,-1.80298243149837,
3.67245986004234));
#48004=CARTESIAN_POINT('Ctrl Pts',(-16.8623904047117,-4.06403136571475,
0.470485342807395));
#48005=CARTESIAN_POINT('Ctrl Pts',(-16.6636133782217,-2.59435596626082,
-3.16338736760251));
#48006=CARTESIAN_POINT('Ctrl Pts',(-16.4648363517318,1.2569009411866,-3.89331626710894));
#48007=CARTESIAN_POINT('Ctrl Pts',(-16.2660593252418,3.95434218350383,-1.04923251768746));
#48008=CARTESIAN_POINT('Ctrl Pts',(-16.0672822987518,3.02174922839628,2.75802643631945));
#48009=CARTESIAN_POINT('Ctrl Pts',(-15.8685052722618,-0.684760449907449,
4.03346652055343));
#48010=CARTESIAN_POINT('Ctrl Pts',(-15.6697282457718,-3.76268269137311,
1.60621997665568));
#48011=CARTESIAN_POINT('Ctrl Pts',(-15.4709512192819,-3.38648959881615,
-2.29547352288112));
#48012=CARTESIAN_POINT('Ctrl Pts',(-15.2721741927919,0.0984043561221374,
-4.09003300476785));
#48013=CARTESIAN_POINT('Ctrl Pts',(-15.0733971663019,3.49305981623661,-2.12984719199018));
#48014=CARTESIAN_POINT('Ctrl Pts',(-14.8746201398119,3.68095040089034,1.78521310053525));
#48015=CARTESIAN_POINT('Ctrl Pts',(-14.6758431133219,0.490138759905249,
4.06204578347229));
#48016=CARTESIAN_POINT('Ctrl Pts',(-14.477066086832,-3.15130940496319,2.60886564553584));
#48017=CARTESIAN_POINT('Ctrl Pts',(-14.278289060342,-3.89854658389887,-1.2370576079239));
#48018=CARTESIAN_POINT('Ctrl Pts',(-14.079512033852,-1.0696280128226,-3.95159389818181));
#48019=CARTESIAN_POINT('Ctrl Pts',(-13.880735007362,2.74665278196318,-3.03017888963131));
#48020=CARTESIAN_POINT('Ctrl Pts',(-13.748216989702,3.60083975147436,-0.574160020683605));
#48021=CARTESIAN_POINT('Ctrl Pts',(-13.681957980872,3.41343113005938,0.562697227949063));
#48022=CARTESIAN_POINT('Ctrl Pts',(-26.267,1.87158653173906,-2.62360084935056));
#48023=CARTESIAN_POINT('Ctrl Pts',(-26.20074099117,2.74538756344498,-2.00026127284245));
#48024=CARTESIAN_POINT('Ctrl Pts',(-26.06822297351,3.80572572838508,0.177707626592857));
#48025=CARTESIAN_POINT('Ctrl Pts',(-25.86944594702,1.90626263650645,3.30303297573159));
#48026=CARTESIAN_POINT('Ctrl Pts',(-25.6706689205301,-1.74511074991996,
3.38706745932803));
#48027=CARTESIAN_POINT('Ctrl Pts',(-25.47189189404,-3.79345908485653,0.366344381091274));
#48028=CARTESIAN_POINT('Ctrl Pts',(-25.2731148675501,-2.36000148581246,
-2.99298991284639));
#48029=CARTESIAN_POINT('Ctrl Pts',(-25.0743378410601,1.24018106922513,-3.60361128581411));
#48030=CARTESIAN_POINT('Ctrl Pts',(-24.8755608145702,3.70175213266751,-0.906781358690897));
#48031=CARTESIAN_POINT('Ctrl Pts',(-24.6767837880802,2.76524014159366,2.62277736241376));
#48032=CARTESIAN_POINT('Ctrl Pts',(-24.4780067615902,-0.709761474991402,
3.74450018637222));
#48033=CARTESIAN_POINT('Ctrl Pts',(-24.2792297351002,-3.53319245332722,
1.42890834602001));
#48034=CARTESIAN_POINT('Ctrl Pts',(-24.0804527086102,-3.11321233646892,
-2.19844466870105));
#48035=CARTESIAN_POINT('Ctrl Pts',(-23.8816756821203,0.16465828588852,-3.80763393731814));
#48036=CARTESIAN_POINT('Ctrl Pts',(-23.6828986556303,3.29137222988386,-1.92148011273296));
#48037=CARTESIAN_POINT('Ctrl Pts',(-23.4841216291403,3.39665395902081,1.72857147389278));
#48038=CARTESIAN_POINT('Ctrl Pts',(-23.2853446026503,0.383854227871474,
3.79181560291581));
#48039=CARTESIAN_POINT('Ctrl Pts',(-23.0865675761604,-2.98131793970147,
2.37422770895388));
#48040=CARTESIAN_POINT('Ctrl Pts',(-22.8877905496704,-3.60968219524731,
-1.22286877331386));
#48041=CARTESIAN_POINT('Ctrl Pts',(-22.6890135231804,-0.924408668548408,
-3.69738843419269));
#48042=CARTESIAN_POINT('Ctrl Pts',(-22.4902364966904,2.60945901488757,-2.7777575280647));
#48043=CARTESIAN_POINT('Ctrl Pts',(-22.2914594702004,3.74787990632693,0.691815984784808));
#48044=CARTESIAN_POINT('Ctrl Pts',(-22.0926824437105,1.44579953705816,3.52631205824809));
#48045=CARTESIAN_POINT('Ctrl Pts',(-21.8939054172205,-2.18350454511998,
3.12370309444941));
#48046=CARTESIAN_POINT('Ctrl Pts',(-21.6951283907305,-3.80838204867393,
-0.146421563192979));
#48047=CARTESIAN_POINT('Ctrl Pts',(-21.4963513642405,-1.93721818400033,
-3.28213326926849));
#48048=CARTESIAN_POINT('Ctrl Pts',(-21.2975743377506,1.71228483279679,-3.40489261991708));
#48049=CARTESIAN_POINT('Ctrl Pts',(-21.0987973112606,3.78993436216897,-0.402008244909776));
#48050=CARTESIAN_POINT('Ctrl Pts',(-20.9000202847706,2.38847724265994,2.96991406583087));
#48051=CARTESIAN_POINT('Ctrl Pts',(-20.7012432582806,-1.20556852363392,
3.6154968722977));
#48052=CARTESIAN_POINT('Ctrl Pts',(-20.5024662317906,-3.6929192749503,0.942104201733542));
#48053=CARTESIAN_POINT('Ctrl Pts',(-20.3036892053007,-2.79022186851798,
-2.59612692727992));
#48054=CARTESIAN_POINT('Ctrl Pts',(-20.1049121788107,0.673860123029691,
-3.75114990807958));
#48055=CARTESIAN_POINT('Ctrl Pts',(-19.9061351523207,3.51934796221725,-1.4626698257142));
#48056=CARTESIAN_POINT('Ctrl Pts',(-19.7073581258307,3.13412367710237,2.16852066508976));
#48057=CARTESIAN_POINT('Ctrl Pts',(-19.5085810993407,-0.128182235481189,
3.80903956563999));
#48058=CARTESIAN_POINT('Ctrl Pts',(-19.3098040728508,-3.27281865164731,
1.95291350849262));
#48059=CARTESIAN_POINT('Ctrl Pts',(-19.1110270463608,-3.41305339688629,
-1.69595978984593));
#48060=CARTESIAN_POINT('Ctrl Pts',(-18.9122500198708,-0.420152939479476,
-3.78796576074431));
#48061=CARTESIAN_POINT('Ctrl Pts',(-18.7134729933808,2.95844202985016,-2.40267223202429));
#48062=CARTESIAN_POINT('Ctrl Pts',(-18.5146959668909,3.62122866324853,1.18824074591766));
#48063=CARTESIAN_POINT('Ctrl Pts',(-18.3159189404009,0.959778114968857,
3.68836536418065));
#48064=CARTESIAN_POINT('Ctrl Pts',(-18.1171419139109,-2.58273529443711,
2.80262225454995));
#48065=CARTESIAN_POINT('Ctrl Pts',(-17.9183648874209,-3.75433389118585,
-0.655888827718381));
#48066=CARTESIAN_POINT('Ctrl Pts',(-17.719587860931,-1.47950656459142,-3.51230314164857));
#48067=CARTESIAN_POINT('Ctrl Pts',(-17.520810834441,2.15348704471131,-3.14447240364953));
#48068=CARTESIAN_POINT('Ctrl Pts',(-17.322033807951,3.80960974798971,0.109939997816874));
#48069=CARTESIAN_POINT('Ctrl Pts',(-17.123256781461,1.96856401336108,3.2634289244733));
#48070=CARTESIAN_POINT('Ctrl Pts',(-16.924479754971,-1.67959578872999,3.42113600634526));
#48071=CARTESIAN_POINT('Ctrl Pts',(-16.725702728481,-3.78591041591479,0.438287798390658));
#48072=CARTESIAN_POINT('Ctrl Pts',(-16.5269257019911,-2.41681187751612,
-2.94690176006388));
#48073=CARTESIAN_POINT('Ctrl Pts',(-16.3281486755011,1.17088524590524,-3.62687816153355));
#48074=CARTESIAN_POINT('Ctrl Pts',(-16.1293716490111,3.68372778490734,-0.977428557993123));
#48075=CARTESIAN_POINT('Ctrl Pts',(-15.9305946225211,2.81495659078308,2.56928160070777));
#48076=CARTESIAN_POINT('Ctrl Pts',(-15.7318175960312,-0.637899043196787,
3.75743726813516));
#48077=CARTESIAN_POINT('Ctrl Pts',(-15.5330405695412,-3.50518446122928,
1.49629872229138));
#48078=CARTESIAN_POINT('Ctrl Pts',(-15.3342635430512,-3.1547360469966,-2.13838337790581));
#48079=CARTESIAN_POINT('Ctrl Pts',(-15.1354865165612,0.0916700791133597,
-3.81013263943217));
#48080=CARTESIAN_POINT('Ctrl Pts',(-14.9367094900712,3.25401315877339,-1.98409164271898));
#48081=CARTESIAN_POINT('Ctrl Pts',(-14.7379324635813,3.42904549919622,1.66304249739848));
#48082=CARTESIAN_POINT('Ctrl Pts',(-14.5391554370913,0.456596238902905,
3.78406071648658));
#48083=CARTESIAN_POINT('Ctrl Pts',(-14.3403784106013,-2.93565034971678,
2.4303285905913));
#48084=CARTESIAN_POINT('Ctrl Pts',(-14.1416013841113,-3.63175054292818,
-1.15239988609244));
#48085=CARTESIAN_POINT('Ctrl Pts',(-13.9428243576214,-0.996428292621477,
-3.68116757779027));
#48086=CARTESIAN_POINT('Ctrl Pts',(-13.7440473311314,2.55868629948601,-2.82280937030186));
#48087=CARTESIAN_POINT('Ctrl Pts',(-13.6115293134714,3.35441720163723,-0.534867526133269));
#48088=CARTESIAN_POINT('Ctrl Pts',(-13.5452703046414,3.17983384142184,0.524189186695443));
#48089=CARTESIAN_POINT('Ctrl Pts',(-13.9553333333333,3.88062570733446,0.639713310456247));
#48090=CARTESIAN_POINT('Ctrl Pts',(-14.0215923421633,4.0936848511486,-0.652745009784315));
#48091=CARTESIAN_POINT('Ctrl Pts',(-14.0878513509933,3.60813529903304,-2.04883146903726));
#48092=CARTESIAN_POINT('Ctrl Pts',(-14.1541103598233,2.64225832295155,-2.92146280044285));
#48093=CARTESIAN_POINT('Ctrl Pts',(-14.2203693686533,1.67638134687004,-3.79409413184845));
#48094=CARTESIAN_POINT('Ctrl Pts',(-14.2866283774833,0.2301769468226,-4.14327033540667));
#48095=CARTESIAN_POINT('Ctrl Pts',(-14.3528873863133,-1.02894378863703,
-3.8035128559561));
#48096=CARTESIAN_POINT('Ctrl Pts',(-14.4191463951433,-2.28806452409662,
-3.46375537650554));
#48097=CARTESIAN_POINT('Ctrl Pts',(-14.4854054039733,-3.36010159496844,
-2.43506421404616));
#48098=CARTESIAN_POINT('Ctrl Pts',(-14.5516644128033,-3.75453493867364,
-1.19199983164787));
#48099=CARTESIAN_POINT('Ctrl Pts',(-14.5720551011905,-3.87591869528357,
-0.809456553166102));
#48100=CARTESIAN_POINT('Ctrl Pts',(-14.5924457895778,-3.93312984357014,
-0.406611012275522));
#48101=CARTESIAN_POINT('Ctrl Pts',(-14.612836477965,-3.92993428904087,-0.00292452251886177));
#48102=CARTESIAN_POINT('Origin',(0.4,7.96243204728166,-1.20090627961635));
#48103=CARTESIAN_POINT('',(6.4,7.90447580357277,-1.2325835755569));
#48104=CARTESIAN_POINT('',(0.4,7.90447580357277,-1.2325835755569));
#48105=CARTESIAN_POINT('',(3.25,7.90447580357277,-1.2325835755569));
#48106=CARTESIAN_POINT('',(6.4,7.68150047349522,-1.35445578580206));
#48107=CARTESIAN_POINT('',(6.4,7.96243204728166,-1.20090627961635));
#48108=CARTESIAN_POINT('',(0.4,7.68150047349522,-1.35445578580206));
#48109=CARTESIAN_POINT('',(0.4,7.68150047349522,-1.35445578580206));
#48110=CARTESIAN_POINT('',(0.4,7.96243204728166,-1.20090627961635));
#48111=CARTESIAN_POINT('Origin',(0.4,7.80460144262175,-1.37616180801042));
#48112=CARTESIAN_POINT('',(0.4,7.84934599497093,-1.54524025679951));
#48113=CARTESIAN_POINT('Origin',(0.4,0.,0.));
#48114=CARTESIAN_POINT('',(0.4,7.68150047349522,-1.35445578580206));
#48115=CARTESIAN_POINT('Origin',(0.4,7.68150047349522,-1.35445578580206));
#48116=CARTESIAN_POINT('',(6.4,7.84934599497093,-1.54524025679951));
#48117=CARTESIAN_POINT('',(3.25,7.84934599497093,-1.54524025679951));
#48118=CARTESIAN_POINT('',(6.4,7.68150047349522,-1.35445578580206));
#48119=CARTESIAN_POINT('Origin',(6.4,7.80460144262175,-1.37616180801042));
#48120=CARTESIAN_POINT('Origin',(6.4,0.,0.));
#48121=CARTESIAN_POINT('Origin',(0.4,7.63292962599169,-2.56532362961446));
#48122=CARTESIAN_POINT('',(6.4,7.57035316313822,-2.58645568014671));
#48123=CARTESIAN_POINT('',(0.4,7.57035316313822,-2.58645568014671));
#48124=CARTESIAN_POINT('',(3.25,7.57035316313822,-2.58645568014671));
#48125=CARTESIAN_POINT('',(6.4,7.32960244213008,-2.66775711794022));
#48126=CARTESIAN_POINT('',(6.4,7.63292962599169,-2.56532362961446));
#48127=CARTESIAN_POINT('',(0.4,7.32960244213008,-2.66775711794022));
#48128=CARTESIAN_POINT('',(0.4,7.32960244213008,-2.66775711794022));
#48129=CARTESIAN_POINT('',(0.4,7.63292962599169,-2.56532362961446));
#48130=CARTESIAN_POINT('Origin',(0.4,7.44706401972832,-2.71050963585593));
#48131=CARTESIAN_POINT('',(0.4,7.46176863727188,-2.88478921306666));
#48132=CARTESIAN_POINT('Origin',(0.4,0.,0.));
#48133=CARTESIAN_POINT('',(0.4,7.32960244213008,-2.66775711794022));
#48134=CARTESIAN_POINT('Origin',(0.4,7.32960244213008,-2.66775711794022));
#48135=CARTESIAN_POINT('',(6.4,7.46176863727188,-2.88478921306666));
#48136=CARTESIAN_POINT('',(3.25,7.46176863727188,-2.88478921306666));
#48137=CARTESIAN_POINT('',(6.4,7.32960244213008,-2.66775711794022));
#48138=CARTESIAN_POINT('Origin',(6.4,7.44706401972832,-2.71050963585593));
#48139=CARTESIAN_POINT('Origin',(6.4,0.,0.));
#48140=CARTESIAN_POINT('Origin',(0.4,7.07150450046473,-3.85179491924312));
#48141=CARTESIAN_POINT('',(6.4,7.00620917262526,-3.86173963770497));
#48142=CARTESIAN_POINT('',(0.4,7.00620917262526,-3.86173963770497));
#48143=CARTESIAN_POINT('',(3.25,7.00620917262526,-3.86173963770497));
#48144=CARTESIAN_POINT('',(6.4,6.75499814951862,-3.9));
#48145=CARTESIAN_POINT('',(6.4,7.07150450046473,-3.85179491924312));
#48146=CARTESIAN_POINT('',(0.4,6.75499814951862,-3.9));
#48147=CARTESIAN_POINT('',(0.4,6.75499814951862,-3.9));
#48148=CARTESIAN_POINT('',(0.4,7.07150450046473,-3.85179491924312));
#48149=CARTESIAN_POINT('Origin',(0.4,6.86325132499167,-3.9625));
#48150=CARTESIAN_POINT('',(0.4,6.84746921536645,-4.13668530886854));
#48151=CARTESIAN_POINT('Origin',(0.4,0.,0.));
#48152=CARTESIAN_POINT('',(0.4,6.75499814951862,-3.9));
#48153=CARTESIAN_POINT('Origin',(0.4,6.75499814951862,-3.9));
#48154=CARTESIAN_POINT('',(6.4,6.84746921536645,-4.13668530886854));
#48155=CARTESIAN_POINT('',(3.25,6.84746921536645,-4.13668530886854));
#48156=CARTESIAN_POINT('',(6.4,6.75499814951862,-3.9));
#48157=CARTESIAN_POINT('Origin',(6.4,6.86325132499167,-3.9625));
#48158=CARTESIAN_POINT('Origin',(6.4,0.,0.));
#48159=CARTESIAN_POINT('Origin',(0.4,6.29521528904508,-5.02123136935285));
#48160=CARTESIAN_POINT('',(6.4,6.22918506171498,-5.01968659050612));
#48161=CARTESIAN_POINT('',(0.4,6.22918506171498,-5.01968659050612));
#48162=CARTESIAN_POINT('',(3.25,6.22918506171498,-5.01968659050612));
#48163=CARTESIAN_POINT('',(6.4,5.97514665632803,-5.01374335555501));
#48164=CARTESIAN_POINT('',(6.4,6.29521528904508,-5.02123136935285));
#48165=CARTESIAN_POINT('',(0.4,5.97514665632803,-5.01374335555501));
#48166=CARTESIAN_POINT('',(0.4,5.97514665632803,-5.01374335555501));
#48167=CARTESIAN_POINT('',(0.4,6.29521528904508,-5.02123136935285));
#48168=CARTESIAN_POINT('Origin',(0.4,6.0709022117179,-5.09409180676583));
#48169=CARTESIAN_POINT('',(0.4,6.02511290633871,-5.26289031482423));
#48170=CARTESIAN_POINT('Origin',(0.4,0.,0.));
#48171=CARTESIAN_POINT('',(0.4,5.97514665632803,-5.01374335555501));
#48172=CARTESIAN_POINT('Origin',(0.4,5.97514665632803,-5.01374335555501));
#48173=CARTESIAN_POINT('',(6.4,6.02511290633871,-5.26289031482423));
#48174=CARTESIAN_POINT('',(3.25,6.02511290633871,-5.26289031482423));
#48175=CARTESIAN_POINT('',(6.4,5.97514665632803,-5.01374335555501));
#48176=CARTESIAN_POINT('Origin',(6.4,6.0709022117179,-5.09409180676583));
#48177=CARTESIAN_POINT('Origin',(6.4,0.,0.));
#48178=CARTESIAN_POINT('Origin',(0.4,5.32764914660044,-6.03810024517047));
#48179=CARTESIAN_POINT('',(6.4,5.26289031482423,-6.02511290633871));
#48180=CARTESIAN_POINT('',(0.4,5.26289031482423,-6.02511290633871));
#48181=CARTESIAN_POINT('',(3.25,5.26289031482423,-6.02511290633871));
#48182=CARTESIAN_POINT('',(6.4,5.01374335555501,-5.97514665632803));
#48183=CARTESIAN_POINT('',(6.4,5.32764914660044,-6.03810024517047));
#48184=CARTESIAN_POINT('',(0.4,5.01374335555501,-5.97514665632803));
#48185=CARTESIAN_POINT('',(0.4,5.01374335555501,-5.97514665632803));
#48186=CARTESIAN_POINT('',(0.4,5.32764914660044,-6.03810024517047));
#48187=CARTESIAN_POINT('Origin',(0.4,5.09409180676582,-6.0709022117179));
#48188=CARTESIAN_POINT('',(0.4,5.01968659050612,-6.22918506171498));
#48189=CARTESIAN_POINT('Origin',(0.4,0.,0.));
#48190=CARTESIAN_POINT('',(0.4,5.01374335555501,-5.97514665632803));
#48191=CARTESIAN_POINT('Origin',(0.4,5.01374335555501,-5.97514665632803));
#48192=CARTESIAN_POINT('',(6.4,5.01968659050612,-6.22918506171498));
#48193=CARTESIAN_POINT('',(3.25,5.01968659050612,-6.22918506171498));
#48194=CARTESIAN_POINT('',(6.4,5.01374335555501,-5.97514665632803));
#48195=CARTESIAN_POINT('Origin',(6.4,5.09409180676582,-6.0709022117179));
#48196=CARTESIAN_POINT('Origin',(6.4,0.,0.));
#48197=CARTESIAN_POINT('Origin',(0.4,4.19820508075689,-6.87150450046473));
#48198=CARTESIAN_POINT('',(6.4,4.13668530886854,-6.84746921536645));
#48199=CARTESIAN_POINT('',(0.4,4.13668530886854,-6.84746921536645));
#48200=CARTESIAN_POINT('',(3.25,4.13668530886854,-6.84746921536645));
#48201=CARTESIAN_POINT('',(6.4,3.9,-6.75499814951862));
#48202=CARTESIAN_POINT('',(6.4,4.19820508075689,-6.87150450046473));
#48203=CARTESIAN_POINT('',(0.4,3.9,-6.75499814951862));
#48204=CARTESIAN_POINT('',(0.4,3.9,-6.75499814951862));
#48205=CARTESIAN_POINT('',(0.4,4.19820508075689,-6.87150450046473));
#48206=CARTESIAN_POINT('Origin',(0.4,3.9625,-6.86325132499168));
#48207=CARTESIAN_POINT('',(0.4,3.86173963770497,-7.00620917262526));
#48208=CARTESIAN_POINT('Origin',(0.4,0.,0.));
#48209=CARTESIAN_POINT('',(0.4,3.9,-6.75499814951862));
#48210=CARTESIAN_POINT('Origin',(0.4,3.9,-6.75499814951862));
#48211=CARTESIAN_POINT('',(6.4,3.86173963770497,-7.00620917262526));
#48212=CARTESIAN_POINT('',(3.25,3.86173963770497,-7.00620917262526));
#48213=CARTESIAN_POINT('',(6.4,3.9,-6.75499814951862));
#48214=CARTESIAN_POINT('Origin',(6.4,3.9625,-6.86325132499168));
#48215=CARTESIAN_POINT('Origin',(6.4,0.,0.));
#48216=CARTESIAN_POINT('Origin',(0.4,2.94120067792881,-7.49612156866143));
#48217=CARTESIAN_POINT('',(6.4,2.88478921306664,-7.46176863727189));
#48218=CARTESIAN_POINT('',(0.4,2.88478921306664,-7.46176863727189));
#48219=CARTESIAN_POINT('',(3.25,2.88478921306664,-7.46176863727189));
#48220=CARTESIAN_POINT('',(6.4,2.66775711794021,-7.32960244213009));
#48221=CARTESIAN_POINT('',(6.4,2.94120067792881,-7.49612156866143));
#48222=CARTESIAN_POINT('',(0.4,2.66775711794021,-7.32960244213009));
#48223=CARTESIAN_POINT('',(0.4,2.66775711794021,-7.32960244213009));
#48224=CARTESIAN_POINT('',(0.4,2.94120067792881,-7.49612156866143));
#48225=CARTESIAN_POINT('Origin',(0.4,2.71050963585592,-7.44706401972833));
#48226=CARTESIAN_POINT('',(0.4,2.5864556801467,-7.57035316313822));
#48227=CARTESIAN_POINT('Origin',(0.4,0.,0.));
#48228=CARTESIAN_POINT('',(0.4,2.66775711794021,-7.32960244213009));
#48229=CARTESIAN_POINT('Origin',(0.4,2.66775711794021,-7.32960244213009));
#48230=CARTESIAN_POINT('',(6.4,2.5864556801467,-7.57035316313822));
#48231=CARTESIAN_POINT('',(3.25,2.5864556801467,-7.57035316313822));
#48232=CARTESIAN_POINT('',(6.4,2.66775711794021,-7.32960244213009));
#48233=CARTESIAN_POINT('Origin',(6.4,2.71050963585592,-7.44706401972833));
#48234=CARTESIAN_POINT('Origin',(6.4,0.,0.));
#48235=CARTESIAN_POINT('Origin',(0.4,1.59482938082123,-7.89297277621489));
#48236=CARTESIAN_POINT('',(6.4,1.5452402567995,-7.84934599497093));
#48237=CARTESIAN_POINT('',(0.4,1.5452402567995,-7.84934599497093));
#48238=CARTESIAN_POINT('',(3.25,1.5452402567995,-7.84934599497093));
#48239=CARTESIAN_POINT('',(6.4,1.35445578580205,-7.68150047349522));
#48240=CARTESIAN_POINT('',(6.4,1.59482938082123,-7.89297277621489));
#48241=CARTESIAN_POINT('',(0.4,1.35445578580205,-7.68150047349522));
#48242=CARTESIAN_POINT('',(0.4,1.35445578580205,-7.68150047349522));
#48243=CARTESIAN_POINT('',(0.4,1.59482938082123,-7.89297277621489));
#48244=CARTESIAN_POINT('Origin',(0.4,1.37616180801042,-7.80460144262175));
#48245=CARTESIAN_POINT('',(0.4,1.2325835755569,-7.90447580357277));
#48246=CARTESIAN_POINT('Origin',(0.4,0.,0.));
#48247=CARTESIAN_POINT('',(0.4,1.35445578580205,-7.68150047349522));
#48248=CARTESIAN_POINT('Origin',(0.4,1.35445578580205,-7.68150047349522));
#48249=CARTESIAN_POINT('',(6.4,1.2325835755569,-7.90447580357277));
#48250=CARTESIAN_POINT('',(3.25,1.2325835755569,-7.90447580357277));
#48251=CARTESIAN_POINT('',(6.4,1.35445578580205,-7.68150047349522));
#48252=CARTESIAN_POINT('Origin',(6.4,1.37616180801042,-7.80460144262175));
#48253=CARTESIAN_POINT('Origin',(6.4,0.,0.));
#48254=CARTESIAN_POINT('Origin',(0.4,0.199999999999999,-8.05));
#48255=CARTESIAN_POINT('',(6.4,0.158739957258808,-7.99842494657351));
#48256=CARTESIAN_POINT('',(0.4,0.158739957258808,-7.99842494657351));
#48257=CARTESIAN_POINT('',(3.25,0.158739957258808,-7.99842494657351));
#48258=CARTESIAN_POINT('',(6.4,-1.4328367550024E-15,-7.8));
#48259=CARTESIAN_POINT('',(6.4,0.199999999999999,-8.05));
#48260=CARTESIAN_POINT('',(0.4,-1.4328367550024E-15,-7.8));
#48261=CARTESIAN_POINT('',(0.4,-1.4328367550024E-15,-7.8));
#48262=CARTESIAN_POINT('',(0.4,0.199999999999999,-8.05));
#48263=CARTESIAN_POINT('Origin',(0.4,-1.45579888248642E-15,-7.925));
#48264=CARTESIAN_POINT('',(0.4,-0.158739957258811,-7.99842494657351));
#48265=CARTESIAN_POINT('Origin',(0.4,0.,0.));
#48266=CARTESIAN_POINT('',(0.4,-1.4328367550024E-15,-7.8));
#48267=CARTESIAN_POINT('Origin',(0.4,-1.4328367550024E-15,-7.8));
#48268=CARTESIAN_POINT('',(6.4,-0.158739957258811,-7.99842494657351));
#48269=CARTESIAN_POINT('',(3.25,-0.158739957258811,-7.99842494657351));
#48270=CARTESIAN_POINT('',(6.4,-1.4328367550024E-15,-7.8));
#48271=CARTESIAN_POINT('Origin',(6.4,-1.45579888248642E-15,-7.925));
#48272=CARTESIAN_POINT('Origin',(6.4,0.,0.));
#48273=CARTESIAN_POINT('Origin',(0.4,-1.20090627961635,-7.96243204728166));
#48274=CARTESIAN_POINT('',(6.4,-1.2325835755569,-7.90447580357277));
#48275=CARTESIAN_POINT('',(0.4,-1.2325835755569,-7.90447580357277));
#48276=CARTESIAN_POINT('',(3.25,-1.2325835755569,-7.90447580357277));
#48277=CARTESIAN_POINT('',(6.4,-1.35445578580206,-7.68150047349522));
#48278=CARTESIAN_POINT('',(6.4,-1.20090627961635,-7.96243204728166));
#48279=CARTESIAN_POINT('',(0.4,-1.35445578580206,-7.68150047349522));
#48280=CARTESIAN_POINT('',(0.4,-1.35445578580206,-7.68150047349522));
#48281=CARTESIAN_POINT('',(0.4,-1.20090627961635,-7.96243204728166));
#48282=CARTESIAN_POINT('Origin',(0.4,-1.37616180801042,-7.80460144262175));
#48283=CARTESIAN_POINT('',(0.4,-1.54524025679951,-7.84934599497093));
#48284=CARTESIAN_POINT('Origin',(0.4,0.,0.));
#48285=CARTESIAN_POINT('',(0.4,-1.35445578580206,-7.68150047349522));
#48286=CARTESIAN_POINT('Origin',(0.4,-1.35445578580206,-7.68150047349522));
#48287=CARTESIAN_POINT('',(6.4,-1.54524025679951,-7.84934599497093));
#48288=CARTESIAN_POINT('',(3.25,-1.54524025679951,-7.84934599497093));
#48289=CARTESIAN_POINT('',(6.4,-1.35445578580206,-7.68150047349522));
#48290=CARTESIAN_POINT('Origin',(6.4,-1.37616180801042,-7.80460144262175));
#48291=CARTESIAN_POINT('Origin',(6.4,0.,0.));
#48292=CARTESIAN_POINT('Origin',(0.4,-2.56532362961446,-7.6329296259917));
#48293=CARTESIAN_POINT('',(6.4,-2.58645568014671,-7.57035316313822));
#48294=CARTESIAN_POINT('',(0.4,-2.58645568014671,-7.57035316313822));
#48295=CARTESIAN_POINT('',(3.25,-2.58645568014671,-7.57035316313822));
#48296=CARTESIAN_POINT('',(6.4,-2.66775711794022,-7.32960244213008));
#48297=CARTESIAN_POINT('',(6.4,-2.56532362961446,-7.6329296259917));
#48298=CARTESIAN_POINT('',(0.4,-2.66775711794022,-7.32960244213008));
#48299=CARTESIAN_POINT('',(0.4,-2.66775711794022,-7.32960244213008));
#48300=CARTESIAN_POINT('',(0.4,-2.56532362961446,-7.6329296259917));
#48301=CARTESIAN_POINT('Origin',(0.4,-2.71050963585593,-7.44706401972832));
#48302=CARTESIAN_POINT('',(0.4,-2.88478921306665,-7.46176863727188));
#48303=CARTESIAN_POINT('Origin',(0.4,0.,0.));
#48304=CARTESIAN_POINT('',(0.4,-2.66775711794022,-7.32960244213008));
#48305=CARTESIAN_POINT('Origin',(0.4,-2.66775711794022,-7.32960244213008));
#48306=CARTESIAN_POINT('',(6.4,-2.88478921306665,-7.46176863727188));
#48307=CARTESIAN_POINT('',(3.25,-2.88478921306665,-7.46176863727188));
#48308=CARTESIAN_POINT('',(6.4,-2.66775711794022,-7.32960244213008));
#48309=CARTESIAN_POINT('Origin',(6.4,-2.71050963585593,-7.44706401972832));
#48310=CARTESIAN_POINT('Origin',(6.4,0.,0.));
#48311=CARTESIAN_POINT('Origin',(0.4,-3.85179491924312,-7.07150450046473));
#48312=CARTESIAN_POINT('',(6.4,-3.86173963770497,-7.00620917262526));
#48313=CARTESIAN_POINT('',(0.4,-3.86173963770497,-7.00620917262526));
#48314=CARTESIAN_POINT('',(3.25,-3.86173963770497,-7.00620917262526));
#48315=CARTESIAN_POINT('',(6.4,-3.9,-6.75499814951862));
#48316=CARTESIAN_POINT('',(6.4,-3.85179491924312,-7.07150450046473));
#48317=CARTESIAN_POINT('',(0.4,-3.9,-6.75499814951862));
#48318=CARTESIAN_POINT('',(0.4,-3.9,-6.75499814951862));
#48319=CARTESIAN_POINT('',(0.4,-3.85179491924312,-7.07150450046473));
#48320=CARTESIAN_POINT('Origin',(0.4,-3.9625,-6.86325132499167));
#48321=CARTESIAN_POINT('',(0.4,-4.13668530886854,-6.84746921536645));
#48322=CARTESIAN_POINT('Origin',(0.4,0.,0.));
#48323=CARTESIAN_POINT('',(0.4,-3.9,-6.75499814951862));
#48324=CARTESIAN_POINT('Origin',(0.4,-3.9,-6.75499814951862));
#48325=CARTESIAN_POINT('',(6.4,-4.13668530886854,-6.84746921536645));
#48326=CARTESIAN_POINT('',(3.25,-4.13668530886854,-6.84746921536645));
#48327=CARTESIAN_POINT('',(6.4,-3.9,-6.75499814951862));
#48328=CARTESIAN_POINT('Origin',(6.4,-3.9625,-6.86325132499167));
#48329=CARTESIAN_POINT('Origin',(6.4,0.,0.));
#48330=CARTESIAN_POINT('Origin',(0.4,-5.02123136935285,-6.29521528904508));
#48331=CARTESIAN_POINT('',(6.4,-5.01968659050612,-6.22918506171498));
#48332=CARTESIAN_POINT('',(0.4,-5.01968659050612,-6.22918506171498));
#48333=CARTESIAN_POINT('',(3.25,-5.01968659050612,-6.22918506171498));
#48334=CARTESIAN_POINT('',(6.4,-5.01374335555501,-5.97514665632803));
#48335=CARTESIAN_POINT('',(6.4,-5.02123136935285,-6.29521528904508));
#48336=CARTESIAN_POINT('',(0.4,-5.01374335555501,-5.97514665632803));
#48337=CARTESIAN_POINT('',(0.4,-5.01374335555501,-5.97514665632803));
#48338=CARTESIAN_POINT('',(0.4,-5.02123136935285,-6.29521528904508));
#48339=CARTESIAN_POINT('Origin',(0.4,-5.09409180676582,-6.0709022117179));
#48340=CARTESIAN_POINT('',(0.4,-5.26289031482423,-6.02511290633871));
#48341=CARTESIAN_POINT('Origin',(0.4,0.,0.));
#48342=CARTESIAN_POINT('',(0.4,-5.01374335555501,-5.97514665632803));
#48343=CARTESIAN_POINT('Origin',(0.4,-5.01374335555501,-5.97514665632803));
#48344=CARTESIAN_POINT('',(6.4,-5.26289031482423,-6.02511290633871));
#48345=CARTESIAN_POINT('',(3.25,-5.26289031482423,-6.02511290633871));
#48346=CARTESIAN_POINT('',(6.4,-5.01374335555501,-5.97514665632803));
#48347=CARTESIAN_POINT('Origin',(6.4,-5.09409180676582,-6.0709022117179));
#48348=CARTESIAN_POINT('Origin',(6.4,0.,0.));
#48349=CARTESIAN_POINT('Origin',(0.4,-6.03810024517047,-5.32764914660044));
#48350=CARTESIAN_POINT('',(6.4,-6.02511290633871,-5.26289031482423));
#48351=CARTESIAN_POINT('',(0.4,-6.02511290633871,-5.26289031482423));
#48352=CARTESIAN_POINT('',(3.25,-6.02511290633871,-5.26289031482423));
#48353=CARTESIAN_POINT('',(6.4,-5.97514665632803,-5.01374335555501));
#48354=CARTESIAN_POINT('',(6.4,-6.03810024517047,-5.32764914660044));
#48355=CARTESIAN_POINT('',(0.4,-5.97514665632803,-5.01374335555501));
#48356=CARTESIAN_POINT('',(0.4,-5.97514665632803,-5.01374335555501));
#48357=CARTESIAN_POINT('',(0.4,-6.03810024517047,-5.32764914660044));
#48358=CARTESIAN_POINT('Origin',(0.4,-6.0709022117179,-5.09409180676582));
#48359=CARTESIAN_POINT('',(0.4,-6.22918506171498,-5.01968659050612));
#48360=CARTESIAN_POINT('Origin',(0.4,0.,0.));
#48361=CARTESIAN_POINT('',(0.4,-5.97514665632803,-5.01374335555501));
#48362=CARTESIAN_POINT('Origin',(0.4,-5.97514665632803,-5.01374335555501));
#48363=CARTESIAN_POINT('',(6.4,-6.22918506171498,-5.01968659050612));
#48364=CARTESIAN_POINT('',(3.25,-6.22918506171498,-5.01968659050612));
#48365=CARTESIAN_POINT('',(6.4,-5.97514665632803,-5.01374335555501));
#48366=CARTESIAN_POINT('Origin',(6.4,-6.0709022117179,-5.09409180676582));
#48367=CARTESIAN_POINT('Origin',(6.4,0.,0.));
#48368=CARTESIAN_POINT('Origin',(0.4,-6.87150450046473,-4.19820508075689));
#48369=CARTESIAN_POINT('',(6.4,-6.84746921536645,-4.13668530886854));
#48370=CARTESIAN_POINT('',(0.4,-6.84746921536645,-4.13668530886854));
#48371=CARTESIAN_POINT('',(3.25,-6.84746921536645,-4.13668530886854));
#48372=CARTESIAN_POINT('',(6.4,-6.75499814951862,-3.9));
#48373=CARTESIAN_POINT('',(6.4,-6.87150450046473,-4.19820508075689));
#48374=CARTESIAN_POINT('',(0.4,-6.75499814951862,-3.9));
#48375=CARTESIAN_POINT('',(0.4,-6.75499814951862,-3.9));
#48376=CARTESIAN_POINT('',(0.4,-6.87150450046473,-4.19820508075689));
#48377=CARTESIAN_POINT('Origin',(0.4,-6.86325132499168,-3.9625));
#48378=CARTESIAN_POINT('',(0.4,-7.00620917262526,-3.86173963770497));
#48379=CARTESIAN_POINT('Origin',(0.4,0.,0.));
#48380=CARTESIAN_POINT('',(0.4,-6.75499814951862,-3.9));
#48381=CARTESIAN_POINT('Origin',(0.4,-6.75499814951862,-3.9));
#48382=CARTESIAN_POINT('',(6.4,-7.00620917262526,-3.86173963770497));
#48383=CARTESIAN_POINT('',(3.25,-7.00620917262526,-3.86173963770497));
#48384=CARTESIAN_POINT('',(6.4,-6.75499814951862,-3.9));
#48385=CARTESIAN_POINT('Origin',(6.4,-6.86325132499168,-3.9625));
#48386=CARTESIAN_POINT('Origin',(6.4,0.,0.));
#48387=CARTESIAN_POINT('Origin',(0.4,-7.49612156866143,-2.94120067792881));
#48388=CARTESIAN_POINT('',(6.4,-7.46176863727189,-2.88478921306665));
#48389=CARTESIAN_POINT('',(0.4,-7.46176863727189,-2.88478921306665));
#48390=CARTESIAN_POINT('',(3.25,-7.46176863727188,-2.88478921306665));
#48391=CARTESIAN_POINT('',(6.4,-7.32960244213009,-2.66775711794022));
#48392=CARTESIAN_POINT('',(6.4,-7.49612156866143,-2.94120067792881));
#48393=CARTESIAN_POINT('',(0.4,-7.32960244213009,-2.66775711794022));
#48394=CARTESIAN_POINT('',(0.4,-7.32960244213009,-2.66775711794022));
#48395=CARTESIAN_POINT('',(0.4,-7.49612156866143,-2.94120067792881));
#48396=CARTESIAN_POINT('Origin',(0.4,-7.44706401972832,-2.71050963585592));
#48397=CARTESIAN_POINT('',(0.4,-7.57035316313822,-2.5864556801467));
#48398=CARTESIAN_POINT('Origin',(0.4,0.,0.));
#48399=CARTESIAN_POINT('',(0.4,-7.32960244213009,-2.66775711794022));
#48400=CARTESIAN_POINT('Origin',(0.4,-7.32960244213009,-2.66775711794022));
#48401=CARTESIAN_POINT('',(6.4,-7.57035316313822,-2.5864556801467));
#48402=CARTESIAN_POINT('',(3.25,-7.57035316313822,-2.5864556801467));
#48403=CARTESIAN_POINT('',(6.4,-7.32960244213009,-2.66775711794022));
#48404=CARTESIAN_POINT('Origin',(6.4,-7.44706401972832,-2.71050963585592));
#48405=CARTESIAN_POINT('Origin',(6.4,0.,0.));
#48406=CARTESIAN_POINT('Origin',(0.4,-7.89297277621489,-1.59482938082123));
#48407=CARTESIAN_POINT('',(6.4,-7.84934599497093,-1.5452402567995));
#48408=CARTESIAN_POINT('',(0.4,-7.84934599497093,-1.5452402567995));
#48409=CARTESIAN_POINT('',(3.25,-7.84934599497093,-1.5452402567995));
#48410=CARTESIAN_POINT('',(6.4,-7.68150047349522,-1.35445578580205));
#48411=CARTESIAN_POINT('',(6.4,-7.89297277621489,-1.59482938082123));
#48412=CARTESIAN_POINT('',(0.4,-7.68150047349522,-1.35445578580205));
#48413=CARTESIAN_POINT('',(0.4,-7.68150047349522,-1.35445578580205));
#48414=CARTESIAN_POINT('',(0.4,-7.89297277621489,-1.59482938082123));
#48415=CARTESIAN_POINT('Origin',(0.4,-7.80460144262175,-1.37616180801042));
#48416=CARTESIAN_POINT('',(0.4,-7.90447580357277,-1.2325835755569));
#48417=CARTESIAN_POINT('Origin',(0.4,0.,0.));
#48418=CARTESIAN_POINT('',(0.4,-7.68150047349522,-1.35445578580205));
#48419=CARTESIAN_POINT('Origin',(0.4,-7.68150047349522,-1.35445578580205));
#48420=CARTESIAN_POINT('',(6.4,-7.90447580357277,-1.2325835755569));
#48421=CARTESIAN_POINT('',(3.25,-7.90447580357277,-1.2325835755569));
#48422=CARTESIAN_POINT('',(6.4,-7.68150047349522,-1.35445578580205));
#48423=CARTESIAN_POINT('Origin',(6.4,-7.80460144262175,-1.37616180801042));
#48424=CARTESIAN_POINT('Origin',(6.4,0.,0.));
#48425=CARTESIAN_POINT('Origin',(0.4,-8.05,-0.199999999999999));
#48426=CARTESIAN_POINT('',(6.4,-7.99842494657351,-0.158739957258808));
#48427=CARTESIAN_POINT('',(0.4,-7.99842494657351,-0.158739957258808));
#48428=CARTESIAN_POINT('',(3.25,-7.99842494657351,-0.158739957258808));
#48429=CARTESIAN_POINT('',(6.4,-7.8,9.55224503334935E-16));
#48430=CARTESIAN_POINT('',(6.4,-8.05,-0.199999999999999));
#48431=CARTESIAN_POINT('',(0.4,-7.8,9.55224503334935E-16));
#48432=CARTESIAN_POINT('',(0.4,-7.8,9.55224503334935E-16));
#48433=CARTESIAN_POINT('',(0.4,-8.05,-0.199999999999999));
#48434=CARTESIAN_POINT('Origin',(0.4,-7.925,9.70532588324277E-16));
#48435=CARTESIAN_POINT('',(0.4,-8.,-9.79717439317883E-16));
#48436=CARTESIAN_POINT('Origin',(0.4,0.,0.));
#48437=CARTESIAN_POINT('',(0.4,-7.99842494657351,0.15873995725881));
#48438=CARTESIAN_POINT('',(0.4,-7.8,9.55224503334935E-16));
#48439=CARTESIAN_POINT('Origin',(0.4,0.,0.));
#48440=CARTESIAN_POINT('Origin',(0.4,-7.8,9.55224503334935E-16));
#48441=CARTESIAN_POINT('',(6.4,-7.99842494657351,0.15873995725881));
#48442=CARTESIAN_POINT('',(3.25,-7.99842494657351,0.15873995725881));
#48443=CARTESIAN_POINT('',(6.4,-7.8,9.55224503334935E-16));
#48444=CARTESIAN_POINT('Origin',(6.4,-7.925,9.70532588324277E-16));
#48445=CARTESIAN_POINT('',(6.4,-8.,-9.79717439317883E-16));
#48446=CARTESIAN_POINT('Origin',(6.4,0.,0.));
#48447=CARTESIAN_POINT('Origin',(6.4,0.,0.));
#48448=CARTESIAN_POINT('Origin',(0.4,-7.96243204728166,1.20090627961635));
#48449=CARTESIAN_POINT('',(6.4,-7.90447580357277,1.23258357555691));
#48450=CARTESIAN_POINT('',(0.4,-7.90447580357277,1.23258357555691));
#48451=CARTESIAN_POINT('',(3.25,-7.90447580357277,1.23258357555691));
#48452=CARTESIAN_POINT('',(6.4,-7.68150047349522,1.35445578580206));
#48453=CARTESIAN_POINT('',(6.4,-7.96243204728166,1.20090627961635));
#48454=CARTESIAN_POINT('',(0.4,-7.68150047349522,1.35445578580206));
#48455=CARTESIAN_POINT('',(0.4,-7.68150047349522,1.35445578580206));
#48456=CARTESIAN_POINT('',(0.4,-7.96243204728166,1.20090627961635));
#48457=CARTESIAN_POINT('Origin',(0.4,-7.80460144262175,1.37616180801043));
#48458=CARTESIAN_POINT('',(0.4,-7.84934599497093,1.54524025679951));
#48459=CARTESIAN_POINT('Origin',(0.4,0.,0.));
#48460=CARTESIAN_POINT('',(0.4,-7.68150047349522,1.35445578580206));
#48461=CARTESIAN_POINT('Origin',(0.4,-7.68150047349522,1.35445578580206));
#48462=CARTESIAN_POINT('',(6.4,-7.84934599497093,1.54524025679951));
#48463=CARTESIAN_POINT('',(3.25,-7.84934599497093,1.54524025679951));
#48464=CARTESIAN_POINT('',(6.4,-7.68150047349522,1.35445578580206));
#48465=CARTESIAN_POINT('Origin',(6.4,-7.80460144262175,1.37616180801043));
#48466=CARTESIAN_POINT('Origin',(6.4,0.,0.));
#48467=CARTESIAN_POINT('Origin',(0.4,-7.6329296259917,2.56532362961445));
#48468=CARTESIAN_POINT('',(6.4,-7.57035316313822,2.58645568014671));
#48469=CARTESIAN_POINT('',(0.4,-7.57035316313822,2.58645568014671));
#48470=CARTESIAN_POINT('',(3.25,-7.57035316313822,2.58645568014671));
#48471=CARTESIAN_POINT('',(6.4,-7.32960244213009,2.66775711794022));
#48472=CARTESIAN_POINT('',(6.4,-7.6329296259917,2.56532362961445));
#48473=CARTESIAN_POINT('',(0.4,-7.32960244213009,2.66775711794022));
#48474=CARTESIAN_POINT('',(0.4,-7.32960244213009,2.66775711794022));
#48475=CARTESIAN_POINT('',(0.4,-7.6329296259917,2.56532362961445));
#48476=CARTESIAN_POINT('Origin',(0.4,-7.44706401972832,2.71050963585593));
#48477=CARTESIAN_POINT('',(0.4,-7.46176863727188,2.88478921306665));
#48478=CARTESIAN_POINT('Origin',(0.4,0.,0.));
#48479=CARTESIAN_POINT('',(0.4,-7.32960244213009,2.66775711794022));
#48480=CARTESIAN_POINT('Origin',(0.4,-7.32960244213009,2.66775711794022));
#48481=CARTESIAN_POINT('',(6.4,-7.46176863727188,2.88478921306665));
#48482=CARTESIAN_POINT('',(3.25,-7.46176863727188,2.88478921306665));
#48483=CARTESIAN_POINT('',(6.4,-7.32960244213009,2.66775711794022));
#48484=CARTESIAN_POINT('Origin',(6.4,-7.44706401972832,2.71050963585593));
#48485=CARTESIAN_POINT('Origin',(6.4,0.,0.));
#48486=CARTESIAN_POINT('Origin',(0.4,-7.07150450046473,3.85179491924311));
#48487=CARTESIAN_POINT('',(6.4,-7.00620917262526,3.86173963770497));
#48488=CARTESIAN_POINT('',(0.4,-7.00620917262526,3.86173963770497));
#48489=CARTESIAN_POINT('',(3.25,-7.00620917262526,3.86173963770497));
#48490=CARTESIAN_POINT('',(6.4,-6.75499814951862,3.9));
#48491=CARTESIAN_POINT('',(6.4,-7.07150450046473,3.85179491924311));
#48492=CARTESIAN_POINT('',(0.4,-6.75499814951862,3.9));
#48493=CARTESIAN_POINT('',(0.4,-6.75499814951862,3.9));
#48494=CARTESIAN_POINT('',(0.4,-7.07150450046473,3.85179491924311));
#48495=CARTESIAN_POINT('Origin',(0.4,-6.86325132499168,3.9625));
#48496=CARTESIAN_POINT('',(0.4,-6.84746921536645,4.13668530886854));
#48497=CARTESIAN_POINT('Origin',(0.4,0.,0.));
#48498=CARTESIAN_POINT('',(0.4,-6.75499814951862,3.9));
#48499=CARTESIAN_POINT('Origin',(0.4,-6.75499814951862,3.9));
#48500=CARTESIAN_POINT('',(6.4,-6.84746921536645,4.13668530886854));
#48501=CARTESIAN_POINT('',(3.25,-6.84746921536645,4.13668530886854));
#48502=CARTESIAN_POINT('',(6.4,-6.75499814951862,3.9));
#48503=CARTESIAN_POINT('Origin',(6.4,-6.86325132499168,3.9625));
#48504=CARTESIAN_POINT('Origin',(6.4,0.,0.));
#48505=CARTESIAN_POINT('Origin',(0.4,-6.29521528904508,5.02123136935285));
#48506=CARTESIAN_POINT('',(6.4,-6.22918506171498,5.01968659050612));
#48507=CARTESIAN_POINT('',(0.4,-6.22918506171498,5.01968659050612));
#48508=CARTESIAN_POINT('',(3.25,-6.22918506171498,5.01968659050612));
#48509=CARTESIAN_POINT('',(6.4,-5.97514665632803,5.01374335555501));
#48510=CARTESIAN_POINT('',(6.4,-6.29521528904508,5.02123136935285));
#48511=CARTESIAN_POINT('',(0.4,-5.97514665632803,5.01374335555501));
#48512=CARTESIAN_POINT('',(0.4,-5.97514665632803,5.01374335555501));
#48513=CARTESIAN_POINT('',(0.4,-6.29521528904508,5.02123136935285));
#48514=CARTESIAN_POINT('Origin',(0.4,-6.0709022117179,5.09409180676582));
#48515=CARTESIAN_POINT('',(0.4,-6.02511290633871,5.26289031482423));
#48516=CARTESIAN_POINT('Origin',(0.4,0.,0.));
#48517=CARTESIAN_POINT('',(0.4,-5.97514665632803,5.01374335555501));
#48518=CARTESIAN_POINT('Origin',(0.4,-5.97514665632803,5.01374335555501));
#48519=CARTESIAN_POINT('',(6.4,-6.02511290633871,5.26289031482423));
#48520=CARTESIAN_POINT('',(3.25,-6.02511290633871,5.26289031482423));
#48521=CARTESIAN_POINT('',(6.4,-5.97514665632803,5.01374335555501));
#48522=CARTESIAN_POINT('Origin',(6.4,-6.0709022117179,5.09409180676582));
#48523=CARTESIAN_POINT('Origin',(6.4,0.,0.));
#48524=CARTESIAN_POINT('Origin',(0.4,-5.32764914660044,6.03810024517047));
#48525=CARTESIAN_POINT('',(6.4,-5.26289031482423,6.02511290633871));
#48526=CARTESIAN_POINT('',(0.4,-5.26289031482423,6.02511290633871));
#48527=CARTESIAN_POINT('',(3.25,-5.26289031482423,6.02511290633871));
#48528=CARTESIAN_POINT('',(6.4,-5.01374335555501,5.97514665632803));
#48529=CARTESIAN_POINT('',(6.4,-5.32764914660044,6.03810024517047));
#48530=CARTESIAN_POINT('',(0.4,-5.01374335555501,5.97514665632803));
#48531=CARTESIAN_POINT('',(0.4,-5.01374335555501,5.97514665632803));
#48532=CARTESIAN_POINT('',(0.4,-5.32764914660044,6.03810024517047));
#48533=CARTESIAN_POINT('Origin',(0.4,-5.09409180676582,6.0709022117179));
#48534=CARTESIAN_POINT('',(0.4,-5.01968659050612,6.22918506171498));
#48535=CARTESIAN_POINT('Origin',(0.4,0.,0.));
#48536=CARTESIAN_POINT('',(0.4,-5.01374335555501,5.97514665632803));
#48537=CARTESIAN_POINT('Origin',(0.4,-5.01374335555501,5.97514665632803));
#48538=CARTESIAN_POINT('',(6.4,-5.01968659050612,6.22918506171498));
#48539=CARTESIAN_POINT('',(3.25,-5.01968659050612,6.22918506171498));
#48540=CARTESIAN_POINT('',(6.4,-5.01374335555501,5.97514665632803));
#48541=CARTESIAN_POINT('Origin',(6.4,-5.09409180676582,6.0709022117179));
#48542=CARTESIAN_POINT('Origin',(6.4,0.,0.));
#48543=CARTESIAN_POINT('Origin',(0.4,-4.19820508075689,6.87150450046473));
#48544=CARTESIAN_POINT('',(6.4,-4.13668530886854,6.84746921536645));
#48545=CARTESIAN_POINT('',(0.4,-4.13668530886854,6.84746921536645));
#48546=CARTESIAN_POINT('',(3.25,-4.13668530886854,6.84746921536645));
#48547=CARTESIAN_POINT('',(6.4,-3.9,6.75499814951862));
#48548=CARTESIAN_POINT('',(6.4,-4.19820508075689,6.87150450046473));
#48549=CARTESIAN_POINT('',(0.4,-3.9,6.75499814951862));
#48550=CARTESIAN_POINT('',(0.4,-3.9,6.75499814951862));
#48551=CARTESIAN_POINT('',(0.4,-4.19820508075689,6.87150450046473));
#48552=CARTESIAN_POINT('Origin',(0.4,-3.9625,6.86325132499168));
#48553=CARTESIAN_POINT('',(0.4,-3.86173963770497,7.00620917262526));
#48554=CARTESIAN_POINT('Origin',(0.4,0.,0.));
#48555=CARTESIAN_POINT('',(0.4,-3.9,6.75499814951862));
#48556=CARTESIAN_POINT('Origin',(0.4,-3.9,6.75499814951862));
#48557=CARTESIAN_POINT('',(6.4,-3.86173963770497,7.00620917262526));
#48558=CARTESIAN_POINT('',(3.25,-3.86173963770497,7.00620917262526));
#48559=CARTESIAN_POINT('',(6.4,-3.9,6.75499814951862));
#48560=CARTESIAN_POINT('Origin',(6.4,-3.9625,6.86325132499168));
#48561=CARTESIAN_POINT('Origin',(6.4,0.,0.));
#48562=CARTESIAN_POINT('Origin',(0.4,-2.94120067792882,7.49612156866143));
#48563=CARTESIAN_POINT('',(6.4,-2.88478921306665,7.46176863727188));
#48564=CARTESIAN_POINT('',(0.4,-2.88478921306665,7.46176863727188));
#48565=CARTESIAN_POINT('',(3.25,-2.88478921306665,7.46176863727188));
#48566=CARTESIAN_POINT('',(6.4,-2.66775711794022,7.32960244213009));
#48567=CARTESIAN_POINT('',(6.4,-2.94120067792882,7.49612156866143));
#48568=CARTESIAN_POINT('',(0.4,-2.66775711794022,7.32960244213009));
#48569=CARTESIAN_POINT('',(0.4,-2.66775711794022,7.32960244213009));
#48570=CARTESIAN_POINT('',(0.4,-2.94120067792882,7.49612156866143));
#48571=CARTESIAN_POINT('Origin',(0.4,-2.71050963585592,7.44706401972832));
#48572=CARTESIAN_POINT('',(0.4,-2.5864556801467,7.57035316313822));
#48573=CARTESIAN_POINT('Origin',(0.4,0.,0.));
#48574=CARTESIAN_POINT('',(0.4,-2.66775711794022,7.32960244213009));
#48575=CARTESIAN_POINT('Origin',(0.4,-2.66775711794022,7.32960244213009));
#48576=CARTESIAN_POINT('',(6.4,-2.5864556801467,7.57035316313822));
#48577=CARTESIAN_POINT('',(3.25,-2.5864556801467,7.57035316313822));
#48578=CARTESIAN_POINT('',(6.4,-2.66775711794022,7.32960244213009));
#48579=CARTESIAN_POINT('Origin',(6.4,-2.71050963585592,7.44706401972832));
#48580=CARTESIAN_POINT('Origin',(6.4,0.,0.));
#48581=CARTESIAN_POINT('Origin',(0.4,-1.59482938082123,7.89297277621489));
#48582=CARTESIAN_POINT('',(6.4,-1.5452402567995,7.84934599497093));
#48583=CARTESIAN_POINT('',(0.4,-1.5452402567995,7.84934599497093));
#48584=CARTESIAN_POINT('',(3.25,-1.5452402567995,7.84934599497093));
#48585=CARTESIAN_POINT('',(6.4,-1.35445578580206,7.68150047349522));
#48586=CARTESIAN_POINT('',(6.4,-1.59482938082123,7.89297277621489));
#48587=CARTESIAN_POINT('',(0.4,-1.35445578580206,7.68150047349522));
#48588=CARTESIAN_POINT('',(0.4,-1.35445578580206,7.68150047349522));
#48589=CARTESIAN_POINT('',(0.4,-1.59482938082123,7.89297277621489));
#48590=CARTESIAN_POINT('Origin',(0.4,-1.37616180801042,7.80460144262175));
#48591=CARTESIAN_POINT('',(0.4,-1.2325835755569,7.90447580357277));
#48592=CARTESIAN_POINT('Origin',(0.4,0.,0.));
#48593=CARTESIAN_POINT('',(0.4,-1.35445578580206,7.68150047349522));
#48594=CARTESIAN_POINT('Origin',(0.4,-1.35445578580206,7.68150047349522));
#48595=CARTESIAN_POINT('',(6.4,-1.2325835755569,7.90447580357277));
#48596=CARTESIAN_POINT('',(3.25,-1.2325835755569,7.90447580357277));
#48597=CARTESIAN_POINT('',(6.4,-1.35445578580206,7.68150047349522));
#48598=CARTESIAN_POINT('Origin',(6.4,-1.37616180801042,7.80460144262175));
#48599=CARTESIAN_POINT('Origin',(6.4,0.,0.));
#48600=CARTESIAN_POINT('Origin',(0.4,-0.2,8.05));
#48601=CARTESIAN_POINT('',(6.4,-0.158739957258808,7.99842494657351));
#48602=CARTESIAN_POINT('',(0.4,-0.158739957258808,7.99842494657351));
#48603=CARTESIAN_POINT('',(3.25,-0.158739957258808,7.99842494657351));
#48604=CARTESIAN_POINT('',(6.4,4.77612251667468E-16,7.8));
#48605=CARTESIAN_POINT('',(6.4,-0.2,8.05));
#48606=CARTESIAN_POINT('',(0.4,4.77612251667468E-16,7.8));
#48607=CARTESIAN_POINT('',(0.4,4.77612251667468E-16,7.8));
#48608=CARTESIAN_POINT('',(0.4,-0.2,8.05));
#48609=CARTESIAN_POINT('Origin',(0.4,4.85266294162139E-16,7.925));
#48610=CARTESIAN_POINT('',(0.4,0.158739957258811,7.99842494657351));
#48611=CARTESIAN_POINT('Origin',(0.4,0.,0.));
#48612=CARTESIAN_POINT('',(0.4,4.77612251667468E-16,7.8));
#48613=CARTESIAN_POINT('Origin',(0.4,4.77612251667468E-16,7.8));
#48614=CARTESIAN_POINT('',(6.4,0.158739957258811,7.99842494657351));
#48615=CARTESIAN_POINT('',(3.25,0.158739957258811,7.99842494657351));
#48616=CARTESIAN_POINT('',(6.4,4.77612251667468E-16,7.8));
#48617=CARTESIAN_POINT('Origin',(6.4,4.85266294162139E-16,7.925));
#48618=CARTESIAN_POINT('Origin',(6.4,0.,0.));
#48619=CARTESIAN_POINT('Origin',(0.4,1.20090627961635,7.96243204728166));
#48620=CARTESIAN_POINT('',(6.4,1.2325835755569,7.90447580357277));
#48621=CARTESIAN_POINT('',(0.4,1.2325835755569,7.90447580357277));
#48622=CARTESIAN_POINT('',(3.25,1.2325835755569,7.90447580357277));
#48623=CARTESIAN_POINT('',(6.4,1.35445578580206,7.68150047349522));
#48624=CARTESIAN_POINT('',(6.4,1.20090627961635,7.96243204728166));
#48625=CARTESIAN_POINT('',(0.4,1.35445578580206,7.68150047349522));
#48626=CARTESIAN_POINT('',(0.4,1.35445578580206,7.68150047349522));
#48627=CARTESIAN_POINT('',(0.4,1.20090627961635,7.96243204728166));
#48628=CARTESIAN_POINT('Origin',(0.4,1.37616180801042,7.80460144262175));
#48629=CARTESIAN_POINT('',(0.4,1.54524025679951,7.84934599497093));
#48630=CARTESIAN_POINT('Origin',(0.4,0.,0.));
#48631=CARTESIAN_POINT('',(0.4,1.35445578580206,7.68150047349522));
#48632=CARTESIAN_POINT('Origin',(0.4,1.35445578580206,7.68150047349522));
#48633=CARTESIAN_POINT('',(6.4,1.54524025679951,7.84934599497093));
#48634=CARTESIAN_POINT('',(3.25,1.54524025679951,7.84934599497093));
#48635=CARTESIAN_POINT('',(6.4,1.35445578580206,7.68150047349522));
#48636=CARTESIAN_POINT('Origin',(6.4,1.37616180801042,7.80460144262175));
#48637=CARTESIAN_POINT('Origin',(6.4,0.,0.));
#48638=CARTESIAN_POINT('Origin',(0.4,2.56532362961445,7.6329296259917));
#48639=CARTESIAN_POINT('',(6.4,2.5864556801467,7.57035316313822));
#48640=CARTESIAN_POINT('',(0.4,2.5864556801467,7.57035316313822));
#48641=CARTESIAN_POINT('',(3.25,2.5864556801467,7.57035316313822));
#48642=CARTESIAN_POINT('',(6.4,2.66775711794022,7.32960244213009));
#48643=CARTESIAN_POINT('',(6.4,2.56532362961445,7.6329296259917));
#48644=CARTESIAN_POINT('',(0.4,2.66775711794022,7.32960244213009));
#48645=CARTESIAN_POINT('',(0.4,2.66775711794022,7.32960244213009));
#48646=CARTESIAN_POINT('',(0.4,2.56532362961445,7.6329296259917));
#48647=CARTESIAN_POINT('Origin',(0.4,2.71050963585593,7.44706401972832));
#48648=CARTESIAN_POINT('',(0.4,2.88478921306665,7.46176863727188));
#48649=CARTESIAN_POINT('Origin',(0.4,0.,0.));
#48650=CARTESIAN_POINT('',(0.4,2.66775711794022,7.32960244213009));
#48651=CARTESIAN_POINT('Origin',(0.4,2.66775711794022,7.32960244213009));
#48652=CARTESIAN_POINT('',(6.4,2.88478921306665,7.46176863727188));
#48653=CARTESIAN_POINT('',(3.25,2.88478921306665,7.46176863727188));
#48654=CARTESIAN_POINT('',(6.4,2.66775711794022,7.32960244213009));
#48655=CARTESIAN_POINT('Origin',(6.4,2.71050963585593,7.44706401972832));
#48656=CARTESIAN_POINT('Origin',(6.4,0.,0.));
#48657=CARTESIAN_POINT('Origin',(0.4,3.85179491924311,7.07150450046473));
#48658=CARTESIAN_POINT('',(6.4,3.86173963770497,7.00620917262526));
#48659=CARTESIAN_POINT('',(0.4,3.86173963770497,7.00620917262526));
#48660=CARTESIAN_POINT('',(3.25,3.86173963770497,7.00620917262526));
#48661=CARTESIAN_POINT('',(6.4,3.9,6.75499814951862));
#48662=CARTESIAN_POINT('',(6.4,3.85179491924311,7.07150450046473));
#48663=CARTESIAN_POINT('',(0.4,3.9,6.75499814951862));
#48664=CARTESIAN_POINT('',(0.4,3.9,6.75499814951862));
#48665=CARTESIAN_POINT('',(0.4,3.85179491924311,7.07150450046473));
#48666=CARTESIAN_POINT('Origin',(0.4,3.9625,6.86325132499168));
#48667=CARTESIAN_POINT('',(0.4,4.13668530886854,6.84746921536645));
#48668=CARTESIAN_POINT('Origin',(0.4,0.,0.));
#48669=CARTESIAN_POINT('',(0.4,3.9,6.75499814951862));
#48670=CARTESIAN_POINT('Origin',(0.4,3.9,6.75499814951862));
#48671=CARTESIAN_POINT('',(6.4,4.13668530886854,6.84746921536645));
#48672=CARTESIAN_POINT('',(3.25,4.13668530886854,6.84746921536645));
#48673=CARTESIAN_POINT('',(6.4,3.9,6.75499814951862));
#48674=CARTESIAN_POINT('Origin',(6.4,3.9625,6.86325132499168));
#48675=CARTESIAN_POINT('Origin',(6.4,0.,0.));
#48676=CARTESIAN_POINT('Origin',(0.4,5.02123136935285,6.29521528904508));
#48677=CARTESIAN_POINT('',(6.4,5.01968659050612,6.22918506171498));
#48678=CARTESIAN_POINT('',(0.4,5.01968659050612,6.22918506171498));
#48679=CARTESIAN_POINT('',(3.25,5.01968659050612,6.22918506171498));
#48680=CARTESIAN_POINT('',(6.4,5.01374335555501,5.97514665632803));
#48681=CARTESIAN_POINT('',(6.4,5.02123136935285,6.29521528904508));
#48682=CARTESIAN_POINT('',(0.4,5.01374335555501,5.97514665632803));
#48683=CARTESIAN_POINT('',(0.4,5.01374335555501,5.97514665632803));
#48684=CARTESIAN_POINT('',(0.4,5.02123136935285,6.29521528904508));
#48685=CARTESIAN_POINT('Origin',(0.4,5.09409180676582,6.0709022117179));
#48686=CARTESIAN_POINT('',(0.4,5.26289031482423,6.02511290633871));
#48687=CARTESIAN_POINT('Origin',(0.4,0.,0.));
#48688=CARTESIAN_POINT('',(0.4,5.01374335555501,5.97514665632803));
#48689=CARTESIAN_POINT('Origin',(0.4,5.01374335555501,5.97514665632803));
#48690=CARTESIAN_POINT('',(6.4,5.26289031482423,6.02511290633871));
#48691=CARTESIAN_POINT('',(3.25,5.26289031482423,6.02511290633871));
#48692=CARTESIAN_POINT('',(6.4,5.01374335555501,5.97514665632803));
#48693=CARTESIAN_POINT('Origin',(6.4,5.09409180676582,6.0709022117179));
#48694=CARTESIAN_POINT('Origin',(6.4,0.,0.));
#48695=CARTESIAN_POINT('Origin',(0.4,6.03810024517047,5.32764914660044));
#48696=CARTESIAN_POINT('',(6.4,6.02511290633871,5.26289031482423));
#48697=CARTESIAN_POINT('',(0.4,6.02511290633871,5.26289031482423));
#48698=CARTESIAN_POINT('',(3.25,6.02511290633871,5.26289031482423));
#48699=CARTESIAN_POINT('',(6.4,5.97514665632803,5.01374335555501));
#48700=CARTESIAN_POINT('',(6.4,6.03810024517047,5.32764914660044));
#48701=CARTESIAN_POINT('',(0.4,5.97514665632803,5.01374335555501));
#48702=CARTESIAN_POINT('',(0.4,5.97514665632803,5.01374335555501));
#48703=CARTESIAN_POINT('',(0.4,6.03810024517047,5.32764914660044));
#48704=CARTESIAN_POINT('Origin',(0.4,6.0709022117179,5.09409180676582));
#48705=CARTESIAN_POINT('',(0.4,6.22918506171498,5.01968659050612));
#48706=CARTESIAN_POINT('Origin',(0.4,0.,0.));
#48707=CARTESIAN_POINT('',(0.4,5.97514665632803,5.01374335555501));
#48708=CARTESIAN_POINT('Origin',(0.4,5.97514665632803,5.01374335555501));
#48709=CARTESIAN_POINT('',(6.4,6.22918506171498,5.01968659050612));
#48710=CARTESIAN_POINT('',(3.25,6.22918506171498,5.01968659050612));
#48711=CARTESIAN_POINT('',(6.4,5.97514665632803,5.01374335555501));
#48712=CARTESIAN_POINT('Origin',(6.4,6.0709022117179,5.09409180676582));
#48713=CARTESIAN_POINT('Origin',(6.4,0.,0.));
#48714=CARTESIAN_POINT('Origin',(0.4,6.87150450046473,4.19820508075689));
#48715=CARTESIAN_POINT('',(6.4,6.84746921536645,4.13668530886854));
#48716=CARTESIAN_POINT('',(0.4,6.84746921536645,4.13668530886854));
#48717=CARTESIAN_POINT('',(3.25,6.84746921536645,4.13668530886854));
#48718=CARTESIAN_POINT('',(6.4,6.75499814951862,3.9));
#48719=CARTESIAN_POINT('',(6.4,6.87150450046473,4.19820508075689));
#48720=CARTESIAN_POINT('',(0.4,6.75499814951862,3.9));
#48721=CARTESIAN_POINT('',(0.4,6.75499814951862,3.9));
#48722=CARTESIAN_POINT('',(0.4,6.87150450046473,4.19820508075689));
#48723=CARTESIAN_POINT('Origin',(0.4,6.86325132499168,3.9625));
#48724=CARTESIAN_POINT('',(0.4,7.00620917262526,3.86173963770497));
#48725=CARTESIAN_POINT('Origin',(0.4,0.,0.));
#48726=CARTESIAN_POINT('',(0.4,6.75499814951862,3.9));
#48727=CARTESIAN_POINT('Origin',(0.4,6.75499814951862,3.9));
#48728=CARTESIAN_POINT('',(6.4,7.00620917262526,3.86173963770497));
#48729=CARTESIAN_POINT('',(3.25,7.00620917262526,3.86173963770497));
#48730=CARTESIAN_POINT('',(6.4,6.75499814951862,3.9));
#48731=CARTESIAN_POINT('Origin',(6.4,6.86325132499168,3.9625));
#48732=CARTESIAN_POINT('Origin',(6.4,0.,0.));
#48733=CARTESIAN_POINT('Origin',(0.4,7.49612156866143,2.94120067792882));
#48734=CARTESIAN_POINT('',(6.4,7.46176863727188,2.88478921306665));
#48735=CARTESIAN_POINT('',(0.4,7.46176863727188,2.88478921306665));
#48736=CARTESIAN_POINT('',(3.25,7.46176863727188,2.88478921306665));
#48737=CARTESIAN_POINT('',(6.4,7.32960244213009,2.66775711794022));
#48738=CARTESIAN_POINT('',(6.4,7.49612156866143,2.94120067792882));
#48739=CARTESIAN_POINT('',(0.4,7.32960244213009,2.66775711794022));
#48740=CARTESIAN_POINT('',(0.4,7.32960244213009,2.66775711794022));
#48741=CARTESIAN_POINT('',(0.4,7.49612156866143,2.94120067792882));
#48742=CARTESIAN_POINT('Origin',(0.4,7.44706401972832,2.71050963585592));
#48743=CARTESIAN_POINT('',(0.4,7.57035316313822,2.5864556801467));
#48744=CARTESIAN_POINT('Origin',(0.4,0.,0.));
#48745=CARTESIAN_POINT('',(0.4,7.32960244213009,2.66775711794022));
#48746=CARTESIAN_POINT('Origin',(0.4,7.32960244213009,2.66775711794022));
#48747=CARTESIAN_POINT('',(6.4,7.57035316313822,2.5864556801467));
#48748=CARTESIAN_POINT('',(3.25,7.57035316313822,2.5864556801467));
#48749=CARTESIAN_POINT('',(6.4,7.32960244213009,2.66775711794022));
#48750=CARTESIAN_POINT('Origin',(6.4,7.44706401972832,2.71050963585592));
#48751=CARTESIAN_POINT('Origin',(6.4,0.,0.));
#48752=CARTESIAN_POINT('Origin',(0.4,7.89297277621489,1.59482938082123));
#48753=CARTESIAN_POINT('',(6.4,7.84934599497093,1.5452402567995));
#48754=CARTESIAN_POINT('',(0.4,7.84934599497093,1.5452402567995));
#48755=CARTESIAN_POINT('',(3.25,7.84934599497093,1.5452402567995));
#48756=CARTESIAN_POINT('',(6.4,7.68150047349522,1.35445578580206));
#48757=CARTESIAN_POINT('',(6.4,7.89297277621489,1.59482938082123));
#48758=CARTESIAN_POINT('',(0.4,7.68150047349522,1.35445578580206));
#48759=CARTESIAN_POINT('',(0.4,7.68150047349522,1.35445578580206));
#48760=CARTESIAN_POINT('',(0.4,7.89297277621489,1.59482938082123));
#48761=CARTESIAN_POINT('Origin',(0.4,7.80460144262175,1.37616180801042));
#48762=CARTESIAN_POINT('',(0.4,7.90447580357277,1.2325835755569));
#48763=CARTESIAN_POINT('Origin',(0.4,0.,0.));
#48764=CARTESIAN_POINT('',(0.4,7.68150047349522,1.35445578580206));
#48765=CARTESIAN_POINT('Origin',(0.4,7.68150047349522,1.35445578580206));
#48766=CARTESIAN_POINT('',(6.4,7.90447580357277,1.2325835755569));
#48767=CARTESIAN_POINT('',(3.25,7.90447580357277,1.2325835755569));
#48768=CARTESIAN_POINT('',(6.4,7.68150047349522,1.35445578580206));
#48769=CARTESIAN_POINT('Origin',(6.4,7.80460144262175,1.37616180801042));
#48770=CARTESIAN_POINT('Origin',(6.4,0.,0.));
#48771=CARTESIAN_POINT('Origin',(0.4,8.05,0.2));
#48772=CARTESIAN_POINT('',(6.4,7.99842494657351,0.158739957258809));
#48773=CARTESIAN_POINT('',(0.4,7.99842494657351,0.158739957258809));
#48774=CARTESIAN_POINT('',(3.25,7.99842494657351,0.158739957258809));
#48775=CARTESIAN_POINT('',(6.4,7.8,0.));
#48776=CARTESIAN_POINT('',(6.4,8.05,0.2));
#48777=CARTESIAN_POINT('',(0.4,7.8,0.));
#48778=CARTESIAN_POINT('',(0.4,7.8,0.));
#48779=CARTESIAN_POINT('',(0.4,8.05,0.2));
#48780=CARTESIAN_POINT('Origin',(0.4,7.925,0.));
#48781=CARTESIAN_POINT('',(0.4,7.99842494657351,-0.158739957258809));
#48782=CARTESIAN_POINT('Origin',(0.4,0.,0.));
#48783=CARTESIAN_POINT('',(0.4,7.8,0.));
#48784=CARTESIAN_POINT('Origin',(0.4,7.8,0.));
#48785=CARTESIAN_POINT('',(6.4,7.99842494657351,-0.158739957258809));
#48786=CARTESIAN_POINT('',(3.25,7.99842494657351,-0.158739957258809));
#48787=CARTESIAN_POINT('',(6.4,7.8,0.));
#48788=CARTESIAN_POINT('Origin',(6.4,7.925,0.));
#48789=CARTESIAN_POINT('Origin',(6.4,0.,0.));
#48790=CARTESIAN_POINT('Origin',(1.75392422621555,0.,0.));
#48791=CARTESIAN_POINT('',(0.997848452431099,0.,0.));
#48792=CARTESIAN_POINT('',(2.5,-2.48346726553949,3.04137023753017E-16));
#48793=CARTESIAN_POINT('',(1.75392422621555,-1.25,-1.53080849893419E-16));
#48794=CARTESIAN_POINT('Origin',(2.5,0.,0.));
#48795=CARTESIAN_POINT('Origin',(7.,0.,2.88675134594813));
#48796=CARTESIAN_POINT('',(7.,1.76762539787484E-16,2.88675134594813));
#48797=CARTESIAN_POINT('',(7.,2.5,1.44337567297406));
#48798=CARTESIAN_POINT('',(7.,0.625,2.52590742770461));
#48799=CARTESIAN_POINT('',(2.5,2.77555756156289E-16,2.88675134594813));
#48800=CARTESIAN_POINT('',(7.,1.76762539787484E-16,2.88675134594813));
#48801=CARTESIAN_POINT('',(2.5,2.5,1.44337567297406));
#48802=CARTESIAN_POINT('',(2.5,2.5,1.44337567297406));
#48803=CARTESIAN_POINT('',(7.,2.5,1.44337567297406));
#48804=CARTESIAN_POINT('Origin',(7.,-2.5,1.44337567297406));
#48805=CARTESIAN_POINT('',(7.,-2.5,1.44337567297406));
#48806=CARTESIAN_POINT('',(7.,-1.875,1.80421959121758));
#48807=CARTESIAN_POINT('',(2.5,-2.5,1.44337567297406));
#48808=CARTESIAN_POINT('',(7.,-2.5,1.44337567297406));
#48809=CARTESIAN_POINT('',(2.5,1.76762539787484E-16,2.88675134594813));
#48810=CARTESIAN_POINT('Origin',(7.,-2.5,-1.44337567297406));
#48811=CARTESIAN_POINT('',(7.,-2.5,-1.44337567297406));
#48812=CARTESIAN_POINT('',(7.,-2.5,-0.721687836487033));
#48813=CARTESIAN_POINT('',(2.5,-2.5,-1.44337567297406));
#48814=CARTESIAN_POINT('',(7.,-2.5,-1.44337567297406));
#48815=CARTESIAN_POINT('',(2.5,-2.5,1.44337567297406));
#48816=CARTESIAN_POINT('Origin',(7.,-5.55111512312578E-16,-2.88675134594813));
#48817=CARTESIAN_POINT('',(7.,-5.30287619362453E-16,-2.88675134594813));
#48818=CARTESIAN_POINT('',(7.,-0.625000000000001,-2.52590742770461));
#48819=CARTESIAN_POINT('',(2.5,-5.55111512312578E-16,-2.88675134594813));
#48820=CARTESIAN_POINT('',(7.,-5.30287619362453E-16,-2.88675134594813));
#48821=CARTESIAN_POINT('',(2.5,-2.5,-1.44337567297406));
#48822=CARTESIAN_POINT('Origin',(7.,2.5,-1.44337567297407));
#48823=CARTESIAN_POINT('',(7.,2.5,-1.44337567297407));
#48824=CARTESIAN_POINT('',(7.,1.875,-1.80421959121758));
#48825=CARTESIAN_POINT('',(2.5,2.5,-1.44337567297407));
#48826=CARTESIAN_POINT('',(7.,2.5,-1.44337567297407));
#48827=CARTESIAN_POINT('',(2.5,-5.30287619362453E-16,-2.88675134594813));
#48828=CARTESIAN_POINT('Origin',(7.,2.5,1.44337567297406));
#48829=CARTESIAN_POINT('',(7.,2.5,0.721687836487032));
#48830=CARTESIAN_POINT('',(2.5,2.5,-1.44337567297407));
#48831=CARTESIAN_POINT('Origin',(2.5,0.,0.));
#48832=CARTESIAN_POINT('Origin',(-0.4,0.,0.));
#48833=CARTESIAN_POINT('',(-0.4,-5.,-6.12323399573677E-16));
#48834=CARTESIAN_POINT('',(-0.4,-6.12323399573677E-16,5.));
#48835=CARTESIAN_POINT('Origin',(-0.4,0.,0.));
#48836=CARTESIAN_POINT('',(0.,-6.61309271539571E-16,5.4));
#48837=CARTESIAN_POINT('Origin',(-0.4,-6.61309271539571E-16,5.4));
#48838=CARTESIAN_POINT('Origin',(0.,0.,0.));
#48839=CARTESIAN_POINT('Origin',(-0.4,0.,0.));
#48840=CARTESIAN_POINT('Origin',(-6.,0.,0.));
#48841=CARTESIAN_POINT('',(-12.,-5.,-6.12323399573677E-16));
#48842=CARTESIAN_POINT('',(-6.,-5.,-6.12323399573677E-16));
#48843=CARTESIAN_POINT('Origin',(-12.,0.,0.));
#48844=CARTESIAN_POINT('Origin',(0.,8.,0.));
#48845=CARTESIAN_POINT('',(0.,-8.,-9.79717439317883E-16));
#48846=CARTESIAN_POINT('Origin',(0.,0.,0.));
#48847=CARTESIAN_POINT('Origin',(-27.,3.2,0.));
#48848=CARTESIAN_POINT('',(-27.,-3.2,-3.91886975727153E-16));
#48849=CARTESIAN_POINT('Origin',(-27.,0.,0.));
#48850=CARTESIAN_POINT('Origin',(-26.6,0.,0.));
#48851=CARTESIAN_POINT('',(-26.6,-3.6,-4.40872847693047E-16));
#48852=CARTESIAN_POINT('Origin',(-20.1,0.,0.));
#48853=CARTESIAN_POINT('Origin',(-13.9553333333333,0.,0.));
#48854=CARTESIAN_POINT('Origin',(-13.75,0.,0.));
#48855=CARTESIAN_POINT('',(-13.5,-3.25,-3.9801020972289E-16));
#48856=CARTESIAN_POINT('Origin',(-13.5,0.,0.));
#48857=CARTESIAN_POINT('',(-13.75,-3.625,-4.43934464690916E-16));
#48858=CARTESIAN_POINT('Origin',(-12.75,0.,0.));
#48859=CARTESIAN_POINT('',(-12.,-3.25,-3.9801020972289E-16));
#48860=CARTESIAN_POINT('Origin',(-12.,0.,0.));
#48861=CARTESIAN_POINT('',(-12.75,-3.25,-3.9801020972289E-16));
#48862=CARTESIAN_POINT('Origin',(-12.,5.,0.));
#48863=CARTESIAN_POINT('Origin',(3.25,0.,0.));
#48864=CARTESIAN_POINT('',(6.5,-8.,-9.79717439317883E-16));
#48865=CARTESIAN_POINT('Origin',(6.5,0.,0.));
#48866=CARTESIAN_POINT('',(3.25,-8.,-9.79717439317883E-16));
#48867=CARTESIAN_POINT('',(3.25,-8.,-9.79717439317883E-16));
#48868=CARTESIAN_POINT('Origin',(6.75,0.,0.));
#48869=CARTESIAN_POINT('',(7.,-7.5,-9.18485099360515E-16));
#48870=CARTESIAN_POINT('Origin',(7.,0.,0.));
#48871=CARTESIAN_POINT('',(6.75,-7.75,-9.49101269339199E-16));
#48872=CARTESIAN_POINT('Origin',(7.,0.,0.));
#82349=UNCERTAINTY_MEASURE_WITH_UNIT(LENGTH_MEASURE(0.01),#82385,
'DISTANCE_ACCURACY_VALUE',
'Maximum model space distance between geometric entities at asserted c
onnectivities');
#82363=UNCERTAINTY_MEASURE_WITH_UNIT(LENGTH_MEASURE(0.01),#82385,
'DISTANCE_ACCURACY_VALUE',
'Maximum model space distance between geometric entities at asserted c
onnectivities');
#82370=(
GEOMETRIC_REPRESENTATION_CONTEXT(3)
GLOBAL_UNCERTAINTY_ASSIGNED_CONTEXT((#82349))
GLOBAL_UNIT_ASSIGNED_CONTEXT((#82385,#82387,#82388))
REPRESENTATION_CONTEXT('','3D')
);
#82384=(
GEOMETRIC_REPRESENTATION_CONTEXT(3)
GLOBAL_UNCERTAINTY_ASSIGNED_CONTEXT((#82363))
GLOBAL_UNIT_ASSIGNED_CONTEXT((#82385,#82387,#82388))
REPRESENTATION_CONTEXT('','3D')
);
#82385=(
LENGTH_UNIT()
NAMED_UNIT(*)
SI_UNIT(.MILLI.,.METRE.)
);
#82387=(
NAMED_UNIT(*)
PLANE_ANGLE_UNIT()
SI_UNIT($,.RADIAN.)
);
#82388=(
NAMED_UNIT(*)
SI_UNIT($,.STERADIAN.)
SOLID_ANGLE_UNIT()
);
#82395=SHAPE_DEFINITION_REPRESENTATION(#82415,#82471);
#82415=PRODUCT_DEFINITION_SHAPE('',$,#82492);
#82471=SHAPE_REPRESENTATION('',(#31784),#82370);
#82485=PRODUCT_DEFINITION_CONTEXT('part definition',#82547,'design');
#82492=PRODUCT_DEFINITION('2026-10-20-12-38-20-714',
'11_ISO_7379_Shoulder_Screw_10x12_M8',#82512,#82485);
#82512=PRODUCT_DEFINITION_FORMATION('',$,#82555);
#82547=APPLICATION_CONTEXT(
'Core Data for Automotive Mechanical Design Process');
#82548=PRODUCT_CONTEXT('part definition',#82547,'mechanical');
#82555=PRODUCT('2026-10-20-12-38-20-714',
'11_ISO_7379_Shoulder_Screw_10x12_M8',$,(#82548));
#82632=COLOUR_RGB('Black',0.12,0.14,0.17);
#82633=FILL_AREA_STYLE_COLOUR('',#82632);
#82634=FILL_AREA_STYLE('',(#82633));
#82635=SURFACE_STYLE_FILL_AREA(#82634);
#82636=SURFACE_SIDE_STYLE('',(#82635));
#82637=SURFACE_STYLE_USAGE(.BOTH.,#82636);
#82638=PRESENTATION_STYLE_ASSIGNMENT((#82637));
ENDSEC;
END-ISO-10303-21;
